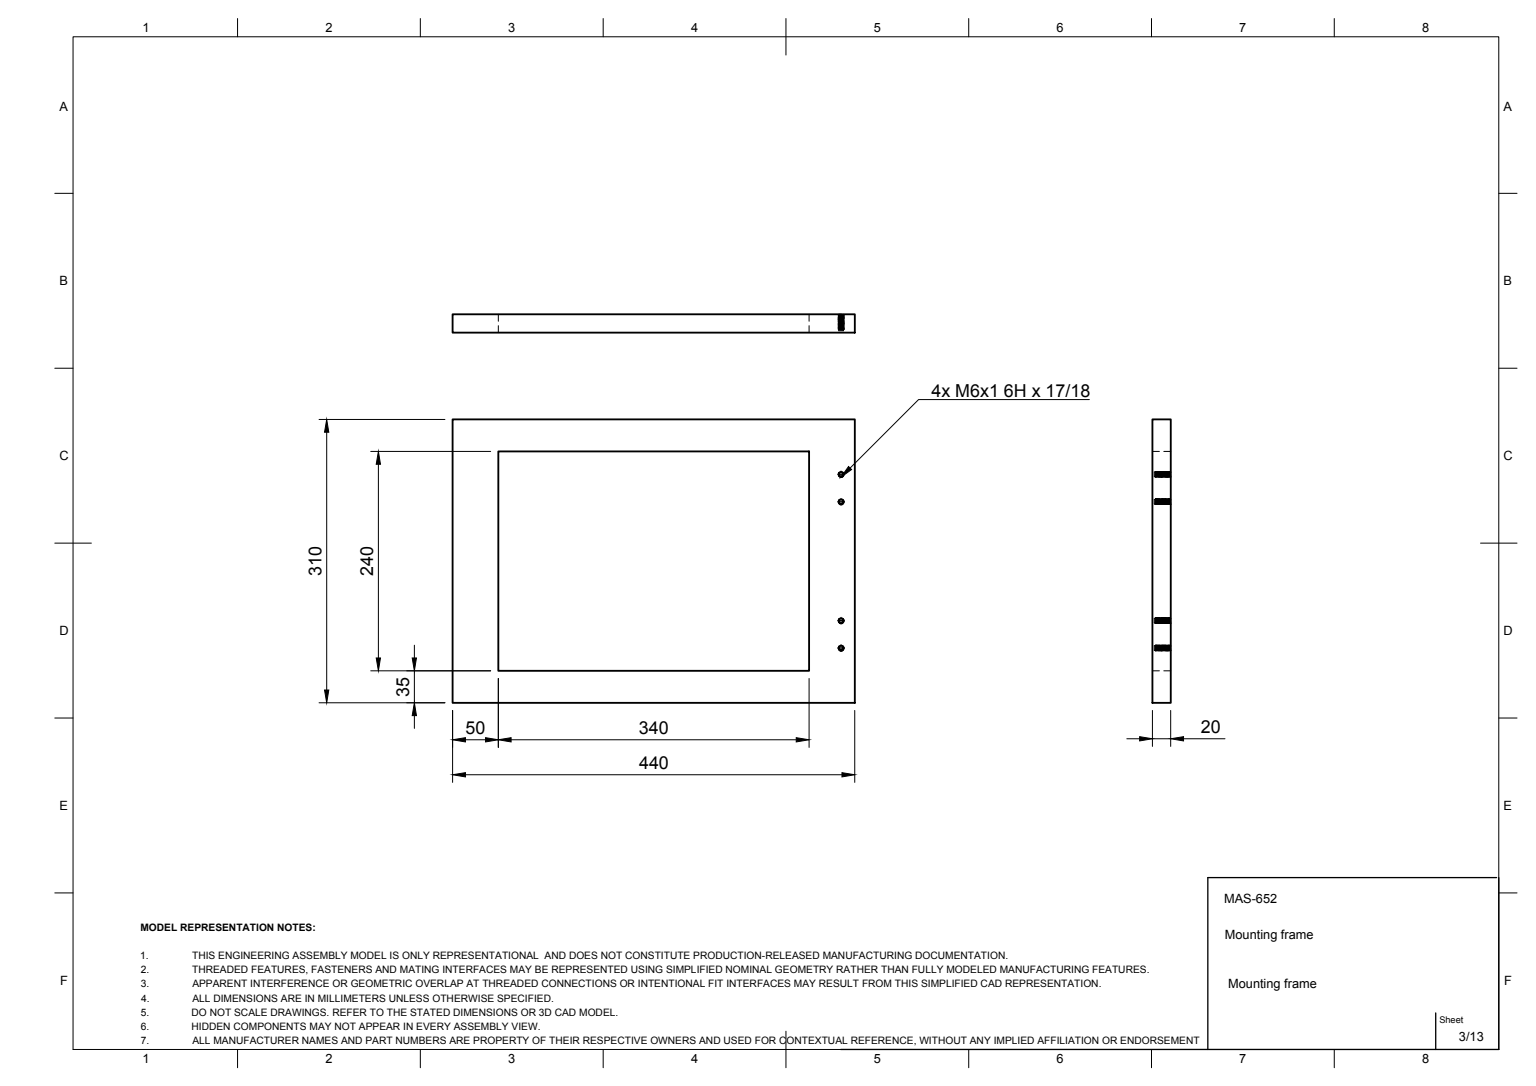
ISO-10303-21;
HEADER;
/* Generated by software containing ST-Developer
 * from STEP Tools, Inc. (www.steptools.com) 
 */

FILE_DESCRIPTION(
/* description */ ('Independent hinged machine back cover with retained hinge pins, perim
eter gasket and quarter-turn cam latch. Nominal cover 360 x 260 x 3 mm
, frame 430 x 300 x 20 mm. No guarding, structural or ingress rating a
ssigned.'),
/* implementation_level */ '2;1');

FILE_NAME(
/* name */ 'Mounting frame.step',
/* time_stamp */ '2026-11-09T19:36:59-08:00',
/* author */ (''),
/* organization */ (''),
/* preprocessor_version */ 'ST-DEVELOPER v20.2',
/* originating_system */ 'Autodesk Translation Framework v15.17.0.0',
/* authorisation */ '');

FILE_SCHEMA (('AUTOMOTIVE_DESIGN { 1 0 10303 214 3 1 1 }'));
ENDSEC;

DATA;
#10=MECHANICAL_DESIGN_GEOMETRIC_PRESENTATION_REPRESENTATION('',(#198),#32627);
#162=SHAPE_REPRESENTATION_RELATIONSHIP('SRR','None',#32708,#180);
#180=ADVANCED_BREP_SHAPE_REPRESENTATION('',(#216),#32609);
#198=STYLED_ITEM('',(#32807),#216);
#216=MANIFOLD_SOLID_BREP('Body1',#8675);
#234=FACE_BOUND('',#1096,.T.);
#235=FACE_BOUND('',#1098,.T.);
#236=FACE_BOUND('',#1099,.T.);
#237=FACE_BOUND('',#1100,.T.);
#238=FACE_BOUND('',#1101,.T.);
#239=FACE_BOUND('',#1102,.T.);
#293=B_SPLINE_SURFACE_WITH_KNOTS('',3,3,((#16428,#16429,#16430,#16431,#16432,
#16433,#16434,#16435,#16436,#16437,#16438,#16439,#16440,#16441,#16442,#16443,
#16444,#16445,#16446,#16447,#16448,#16449,#16450,#16451,#16452,#16453,#16454,
#16455,#16456,#16457,#16458,#16459,#16460,#16461,#16462,#16463,#16464,#16465,
#16466,#16467,#16468,#16469,#16470,#16471,#16472,#16473,#16474,#16475,#16476,
#16477,#16478,#16479,#16480,#16481,#16482,#16483,#16484,#16485,#16486,#16487,
#16488,#16489,#16490,#16491,#16492,#16493,#16494,#16495,#16496,#16497,#16498,
#16499,#16500,#16501,#16502,#16503,#16504,#16505,#16506,#16507,#16508,#16509,
#16510,#16511,#16512,#16513,#16514,#16515,#16516,#16517,#16518,#16519,#16520,
#16521,#16522,#16523,#16524,#16525,#16526,#16527,#16528,#16529,#16530,#16531,
#16532,#16533,#16534,#16535,#16536,#16537,#16538,#16539),(#16540,#16541,
#16542,#16543,#16544,#16545,#16546,#16547,#16548,#16549,#16550,#16551,#16552,
#16553,#16554,#16555,#16556,#16557,#16558,#16559,#16560,#16561,#16562,#16563,
#16564,#16565,#16566,#16567,#16568,#16569,#16570,#16571,#16572,#16573,#16574,
#16575,#16576,#16577,#16578,#16579,#16580,#16581,#16582,#16583,#16584,#16585,
#16586,#16587,#16588,#16589,#16590,#16591,#16592,#16593,#16594,#16595,#16596,
#16597,#16598,#16599,#16600,#16601,#16602,#16603,#16604,#16605,#16606,#16607,
#16608,#16609,#16610,#16611,#16612,#16613,#16614,#16615,#16616,#16617,#16618,
#16619,#16620,#16621,#16622,#16623,#16624,#16625,#16626,#16627,#16628,#16629,
#16630,#16631,#16632,#16633,#16634,#16635,#16636,#16637,#16638,#16639,#16640,
#16641,#16642,#16643,#16644,#16645,#16646,#16647,#16648,#16649,#16650,#16651),
(#16652,#16653,#16654,#16655,#16656,#16657,#16658,#16659,#16660,#16661,
#16662,#16663,#16664,#16665,#16666,#16667,#16668,#16669,#16670,#16671,#16672,
#16673,#16674,#16675,#16676,#16677,#16678,#16679,#16680,#16681,#16682,#16683,
#16684,#16685,#16686,#16687,#16688,#16689,#16690,#16691,#16692,#16693,#16694,
#16695,#16696,#16697,#16698,#16699,#16700,#16701,#16702,#16703,#16704,#16705,
#16706,#16707,#16708,#16709,#16710,#16711,#16712,#16713,#16714,#16715,#16716,
#16717,#16718,#16719,#16720,#16721,#16722,#16723,#16724,#16725,#16726,#16727,
#16728,#16729,#16730,#16731,#16732,#16733,#16734,#16735,#16736,#16737,#16738,
#16739,#16740,#16741,#16742,#16743,#16744,#16745,#16746,#16747,#16748,#16749,
#16750,#16751,#16752,#16753,#16754,#16755,#16756,#16757,#16758,#16759,#16760,
#16761,#16762,#16763),(#16764,#16765,#16766,#16767,#16768,#16769,#16770,
#16771,#16772,#16773,#16774,#16775,#16776,#16777,#16778,#16779,#16780,#16781,
#16782,#16783,#16784,#16785,#16786,#16787,#16788,#16789,#16790,#16791,#16792,
#16793,#16794,#16795,#16796,#16797,#16798,#16799,#16800,#16801,#16802,#16803,
#16804,#16805,#16806,#16807,#16808,#16809,#16810,#16811,#16812,#16813,#16814,
#16815,#16816,#16817,#16818,#16819,#16820,#16821,#16822,#16823,#16824,#16825,
#16826,#16827,#16828,#16829,#16830,#16831,#16832,#16833,#16834,#16835,#16836,
#16837,#16838,#16839,#16840,#16841,#16842,#16843,#16844,#16845,#16846,#16847,
#16848,#16849,#16850,#16851,#16852,#16853,#16854,#16855,#16856,#16857,#16858,
#16859,#16860,#16861,#16862,#16863,#16864,#16865,#16866,#16867,#16868,#16869,
#16870,#16871,#16872,#16873,#16874,#16875)),.UNSPECIFIED.,.F.,.F.,.F.,(4,
4),(4,1,1,1,1,1,1,1,1,1,1,1,1,1,1,1,1,1,1,1,1,1,1,1,1,1,1,1,1,1,1,1,1,1,
1,1,1,1,1,1,1,1,1,1,1,1,1,1,1,1,1,1,1,1,1,1,1,1,1,1,1,1,1,1,1,1,1,1,1,1,
1,1,1,1,1,1,1,1,1,1,1,1,1,1,1,1,1,1,1,1,1,1,1,1,1,1,1,1,1,1,1,1,1,1,1,1,
1,1,1,4),(0.,0.064201349933888),(11.8589888623077,12.8574392762075,13.8558896901074,
14.8543401040072,15.852790517907,16.8512409318069,17.8496913457067,18.8481417596065,
19.8465921735064,20.8450425874062,21.843493001306,22.8419434152058,23.8403938291057,
24.8388442430055,25.8372946569053,26.8357450708052,27.834195484705,28.8326458986048,
29.8310963125046,30.8295467264045,31.8279971403043,32.8264475542041,33.824897968104,
34.8233483820038,35.8217987959036,36.8202492098035,37.8186996237033,38.8171500376031,
39.8156004515029,40.8140508654028,41.8125012793026,42.8109516932024,43.8094021071023,
44.8078525210021,45.8063029349019,46.8047533488018,47.8032037627016,48.8016541766014,
49.8001045905012,50.7985550044011,51.7970054183009,52.7954558322007,53.7939062461006,
54.7923566600004,55.7908070739002,56.7892574878001,57.7877079016999,58.7861583155997,
59.7846087294995,60.7830591433994,61.7815095572992,62.779959971199,63.7784103850989,
64.7768607989987,65.7753112128985,66.7737616267983,67.7722120406982,68.770662454598,
69.7691128684978,70.7675632823977,71.7660136962975,72.7644641101973,73.7629145240972,
74.761364937997,75.7598153518968,76.7582657657966,77.7567161796965,78.7551665935963,
79.7536170074961,80.7520674213959,81.7505178352958,82.7489682491956,83.7474186630954,
84.7458690769953,85.7443194908951,86.7427699047949,87.7412203186948,88.7396707325946,
89.7381211464944,90.7365715603943,91.7350219742941,92.7334723881939,93.7319228020937,
94.7303732159936,95.7288236298934,96.7272740437932,97.7257244576931,98.7241748715929,
99.7226252854927,100.721075699393,101.719526113292,102.717976527192,103.716426941092,
104.714877354992,105.713327768892,106.711778182792,107.710228596691,108.708679010591,
109.707129424491,110.705579838391,111.704030252291,112.70248066619,113.70093108009,
114.69938149399,115.69783190789,116.69628232179,117.69473273569,118.693183149589,
119.691633563489,120.690083977389),.UNSPECIFIED.);
#294=B_SPLINE_SURFACE_WITH_KNOTS('',3,3,((#16998,#16999,#17000,#17001,#17002,
#17003,#17004,#17005,#17006,#17007,#17008,#17009,#17010,#17011,#17012,#17013,
#17014,#17015,#17016,#17017,#17018,#17019,#17020,#17021,#17022,#17023,#17024,
#17025,#17026,#17027,#17028,#17029,#17030,#17031,#17032,#17033,#17034,#17035,
#17036,#17037,#17038,#17039,#17040,#17041,#17042,#17043,#17044,#17045,#17046,
#17047,#17048,#17049,#17050,#17051,#17052,#17053,#17054,#17055,#17056,#17057,
#17058,#17059,#17060,#17061,#17062,#17063,#17064,#17065,#17066,#17067,#17068,
#17069,#17070,#17071,#17072,#17073,#17074,#17075,#17076,#17077,#17078,#17079,
#17080,#17081,#17082,#17083,#17084,#17085,#17086,#17087,#17088,#17089,#17090,
#17091,#17092,#17093,#17094,#17095,#17096,#17097,#17098,#17099,#17100,#17101,
#17102,#17103,#17104,#17105,#17106,#17107,#17108,#17109),(#17110,#17111,
#17112,#17113,#17114,#17115,#17116,#17117,#17118,#17119,#17120,#17121,#17122,
#17123,#17124,#17125,#17126,#17127,#17128,#17129,#17130,#17131,#17132,#17133,
#17134,#17135,#17136,#17137,#17138,#17139,#17140,#17141,#17142,#17143,#17144,
#17145,#17146,#17147,#17148,#17149,#17150,#17151,#17152,#17153,#17154,#17155,
#17156,#17157,#17158,#17159,#17160,#17161,#17162,#17163,#17164,#17165,#17166,
#17167,#17168,#17169,#17170,#17171,#17172,#17173,#17174,#17175,#17176,#17177,
#17178,#17179,#17180,#17181,#17182,#17183,#17184,#17185,#17186,#17187,#17188,
#17189,#17190,#17191,#17192,#17193,#17194,#17195,#17196,#17197,#17198,#17199,
#17200,#17201,#17202,#17203,#17204,#17205,#17206,#17207,#17208,#17209,#17210,
#17211,#17212,#17213,#17214,#17215,#17216,#17217,#17218,#17219,#17220,#17221),
(#17222,#17223,#17224,#17225,#17226,#17227,#17228,#17229,#17230,#17231,
#17232,#17233,#17234,#17235,#17236,#17237,#17238,#17239,#17240,#17241,#17242,
#17243,#17244,#17245,#17246,#17247,#17248,#17249,#17250,#17251,#17252,#17253,
#17254,#17255,#17256,#17257,#17258,#17259,#17260,#17261,#17262,#17263,#17264,
#17265,#17266,#17267,#17268,#17269,#17270,#17271,#17272,#17273,#17274,#17275,
#17276,#17277,#17278,#17279,#17280,#17281,#17282,#17283,#17284,#17285,#17286,
#17287,#17288,#17289,#17290,#17291,#17292,#17293,#17294,#17295,#17296,#17297,
#17298,#17299,#17300,#17301,#17302,#17303,#17304,#17305,#17306,#17307,#17308,
#17309,#17310,#17311,#17312,#17313,#17314,#17315,#17316,#17317,#17318,#17319,
#17320,#17321,#17322,#17323,#17324,#17325,#17326,#17327,#17328,#17329,#17330,
#17331,#17332,#17333),(#17334,#17335,#17336,#17337,#17338,#17339,#17340,
#17341,#17342,#17343,#17344,#17345,#17346,#17347,#17348,#17349,#17350,#17351,
#17352,#17353,#17354,#17355,#17356,#17357,#17358,#17359,#17360,#17361,#17362,
#17363,#17364,#17365,#17366,#17367,#17368,#17369,#17370,#17371,#17372,#17373,
#17374,#17375,#17376,#17377,#17378,#17379,#17380,#17381,#17382,#17383,#17384,
#17385,#17386,#17387,#17388,#17389,#17390,#17391,#17392,#17393,#17394,#17395,
#17396,#17397,#17398,#17399,#17400,#17401,#17402,#17403,#17404,#17405,#17406,
#17407,#17408,#17409,#17410,#17411,#17412,#17413,#17414,#17415,#17416,#17417,
#17418,#17419,#17420,#17421,#17422,#17423,#17424,#17425,#17426,#17427,#17428,
#17429,#17430,#17431,#17432,#17433,#17434,#17435,#17436,#17437,#17438,#17439,
#17440,#17441,#17442,#17443,#17444,#17445)),.UNSPECIFIED.,.F.,.F.,.F.,(4,
4),(4,1,1,1,1,1,1,1,1,1,1,1,1,1,1,1,1,1,1,1,1,1,1,1,1,1,1,1,1,1,1,1,1,1,
1,1,1,1,1,1,1,1,1,1,1,1,1,1,1,1,1,1,1,1,1,1,1,1,1,1,1,1,1,1,1,1,1,1,1,1,
1,1,1,1,1,1,1,1,1,1,1,1,1,1,1,1,1,1,1,1,1,1,1,1,1,1,1,1,1,1,1,1,1,1,1,1,
1,1,1,4),(0.,0.064201349933888),(14.3984001269718,15.3968505408716,16.3953009547714,
17.3937513686712,18.3922017825711,19.3906521964709,20.3891026103707,21.3875530242706,
22.3860034381704,23.3844538520702,24.3829042659701,25.3813546798699,26.3798050937697,
27.3782555076695,28.3767059215694,29.3751563354692,30.373606749369,31.3720571632689,
32.3705075771687,33.3689579910685,34.3674084049683,35.3658588188682,36.364309232768,
37.3627596466678,38.3612100605677,39.3596604744675,40.3581108883673,41.3565613022672,
42.355011716167,43.3534621300668,44.3519125439666,45.3503629578665,46.3488133717663,
47.3472637856661,48.345714199566,49.3441646134658,50.3426150273656,51.3410654412654,
52.3395158551653,53.3379662690651,54.3364166829649,55.3348670968648,56.3333175107646,
57.3317679246644,58.3302183385643,59.3286687524641,60.3271191663639,61.3255695802637,
62.3240199941636,63.3224704080634,64.3209208219632,65.3193712358631,66.3178216497629,
67.3162720636627,68.3147224775625,69.3131728914624,70.3116233053622,71.310073719262,
72.3085241331619,73.3069745470617,74.3054249609615,75.3038753748613,76.3023257887612,
77.300776202661,78.2992266165608,79.2976770304607,80.2961274443605,81.2945778582603,
82.2930282721602,83.29147868606,84.2899290999598,85.2883795138596,86.2868299277595,
87.2852803416593,88.2837307555591,89.282181169459,90.2806315833588,91.2790819972586,
92.2775324111584,93.2759828250583,94.2744332389581,95.2728836528579,96.2713340667578,
97.2697844806576,98.2682348945574,99.2666853084573,100.265135722357,101.263586136257,
102.262036550157,103.260486964057,104.258937377956,105.257387791856,106.255838205756,
107.254288619656,108.252739033556,109.251189447456,110.249639861355,111.248090275255,
112.246540689155,113.244991103055,114.243441516955,115.241891930855,116.240342344754,
117.238792758654,118.237243172554,119.235693586454,120.234144000354,121.232594414253,
122.231044828153,123.229495242053),.UNSPECIFIED.);
#295=B_SPLINE_SURFACE_WITH_KNOTS('',3,3,((#17768,#17769,#17770,#17771,#17772,
#17773,#17774,#17775,#17776,#17777,#17778,#17779,#17780,#17781,#17782,#17783,
#17784,#17785,#17786,#17787,#17788,#17789,#17790,#17791,#17792,#17793,#17794,
#17795,#17796,#17797,#17798,#17799,#17800,#17801,#17802,#17803,#17804,#17805,
#17806,#17807,#17808,#17809,#17810,#17811,#17812,#17813,#17814,#17815,#17816,
#17817,#17818,#17819,#17820,#17821,#17822,#17823,#17824,#17825,#17826,#17827,
#17828,#17829,#17830,#17831,#17832,#17833,#17834,#17835,#17836,#17837,#17838,
#17839,#17840,#17841,#17842,#17843,#17844,#17845,#17846,#17847,#17848,#17849,
#17850,#17851,#17852,#17853,#17854,#17855,#17856,#17857,#17858,#17859,#17860,
#17861,#17862,#17863,#17864,#17865,#17866,#17867,#17868,#17869,#17870,#17871,
#17872,#17873,#17874,#17875,#17876,#17877,#17878,#17879),(#17880,#17881,
#17882,#17883,#17884,#17885,#17886,#17887,#17888,#17889,#17890,#17891,#17892,
#17893,#17894,#17895,#17896,#17897,#17898,#17899,#17900,#17901,#17902,#17903,
#17904,#17905,#17906,#17907,#17908,#17909,#17910,#17911,#17912,#17913,#17914,
#17915,#17916,#17917,#17918,#17919,#17920,#17921,#17922,#17923,#17924,#17925,
#17926,#17927,#17928,#17929,#17930,#17931,#17932,#17933,#17934,#17935,#17936,
#17937,#17938,#17939,#17940,#17941,#17942,#17943,#17944,#17945,#17946,#17947,
#17948,#17949,#17950,#17951,#17952,#17953,#17954,#17955,#17956,#17957,#17958,
#17959,#17960,#17961,#17962,#17963,#17964,#17965,#17966,#17967,#17968,#17969,
#17970,#17971,#17972,#17973,#17974,#17975,#17976,#17977,#17978,#17979,#17980,
#17981,#17982,#17983,#17984,#17985,#17986,#17987,#17988,#17989,#17990,#17991),
(#17992,#17993,#17994,#17995,#17996,#17997,#17998,#17999,#18000,#18001,
#18002,#18003,#18004,#18005,#18006,#18007,#18008,#18009,#18010,#18011,#18012,
#18013,#18014,#18015,#18016,#18017,#18018,#18019,#18020,#18021,#18022,#18023,
#18024,#18025,#18026,#18027,#18028,#18029,#18030,#18031,#18032,#18033,#18034,
#18035,#18036,#18037,#18038,#18039,#18040,#18041,#18042,#18043,#18044,#18045,
#18046,#18047,#18048,#18049,#18050,#18051,#18052,#18053,#18054,#18055,#18056,
#18057,#18058,#18059,#18060,#18061,#18062,#18063,#18064,#18065,#18066,#18067,
#18068,#18069,#18070,#18071,#18072,#18073,#18074,#18075,#18076,#18077,#18078,
#18079,#18080,#18081,#18082,#18083,#18084,#18085,#18086,#18087,#18088,#18089,
#18090,#18091,#18092,#18093,#18094,#18095,#18096,#18097,#18098,#18099,#18100,
#18101,#18102,#18103),(#18104,#18105,#18106,#18107,#18108,#18109,#18110,
#18111,#18112,#18113,#18114,#18115,#18116,#18117,#18118,#18119,#18120,#18121,
#18122,#18123,#18124,#18125,#18126,#18127,#18128,#18129,#18130,#18131,#18132,
#18133,#18134,#18135,#18136,#18137,#18138,#18139,#18140,#18141,#18142,#18143,
#18144,#18145,#18146,#18147,#18148,#18149,#18150,#18151,#18152,#18153,#18154,
#18155,#18156,#18157,#18158,#18159,#18160,#18161,#18162,#18163,#18164,#18165,
#18166,#18167,#18168,#18169,#18170,#18171,#18172,#18173,#18174,#18175,#18176,
#18177,#18178,#18179,#18180,#18181,#18182,#18183,#18184,#18185,#18186,#18187,
#18188,#18189,#18190,#18191,#18192,#18193,#18194,#18195,#18196,#18197,#18198,
#18199,#18200,#18201,#18202,#18203,#18204,#18205,#18206,#18207,#18208,#18209,
#18210,#18211,#18212,#18213,#18214,#18215)),.UNSPECIFIED.,.F.,.F.,.F.,(4,
4),(4,1,1,1,1,1,1,1,1,1,1,1,1,1,1,1,1,1,1,1,1,1,1,1,1,1,1,1,1,1,1,1,1,1,
1,1,1,1,1,1,1,1,1,1,1,1,1,1,1,1,1,1,1,1,1,1,1,1,1,1,1,1,1,1,1,1,1,1,1,1,
1,1,1,1,1,1,1,1,1,1,1,1,1,1,1,1,1,1,1,1,1,1,1,1,1,1,1,1,1,1,1,1,1,1,1,1,
1,1,1,4),(0.,0.064201349933888),(11.8589888623077,12.8574392762076,13.8558896901074,
14.8543401040072,15.852790517907,16.8512409318069,17.8496913457067,18.8481417596065,
19.8465921735064,20.8450425874062,21.843493001306,22.8419434152058,23.8403938291057,
24.8388442430055,25.8372946569053,26.8357450708052,27.834195484705,28.8326458986048,
29.8310963125047,30.8295467264045,31.8279971403043,32.8264475542041,33.824897968104,
34.8233483820038,35.8217987959036,36.8202492098035,37.8186996237033,38.8171500376031,
39.8156004515029,40.8140508654028,41.8125012793026,42.8109516932024,43.8094021071023,
44.8078525210021,45.8063029349019,46.8047533488018,47.8032037627016,48.8016541766014,
49.8001045905012,50.7985550044011,51.7970054183009,52.7954558322007,53.7939062461006,
54.7923566600004,55.7908070739002,56.7892574878001,57.7877079016999,58.7861583155997,
59.7846087294995,60.7830591433994,61.7815095572992,62.779959971199,63.7784103850989,
64.7768607989987,65.7753112128985,66.7737616267983,67.7722120406982,68.770662454598,
69.7691128684978,70.7675632823977,71.7660136962975,72.7644641101973,73.7629145240971,
74.761364937997,75.7598153518968,76.7582657657966,77.7567161796965,78.7551665935963,
79.7536170074961,80.7520674213959,81.7505178352958,82.7489682491956,83.7474186630954,
84.7458690769953,85.7443194908951,86.7427699047949,87.7412203186948,88.7396707325946,
89.7381211464944,90.7365715603942,91.7350219742941,92.7334723881939,93.7319228020937,
94.7303732159936,95.7288236298934,96.7272740437932,97.725724457693,98.7241748715929,
99.7226252854927,100.721075699393,101.719526113292,102.717976527192,103.716426941092,
104.714877354992,105.713327768892,106.711778182792,107.710228596691,108.708679010591,
109.707129424491,110.705579838391,111.704030252291,112.70248066619,113.70093108009,
114.69938149399,115.69783190789,116.69628232179,117.69473273569,118.693183149589,
119.691633563489,120.690083977389),.UNSPECIFIED.);
#296=B_SPLINE_SURFACE_WITH_KNOTS('',3,3,((#18338,#18339,#18340,#18341,#18342,
#18343,#18344,#18345,#18346,#18347,#18348,#18349,#18350,#18351,#18352,#18353,
#18354,#18355,#18356,#18357,#18358,#18359,#18360,#18361,#18362,#18363,#18364,
#18365,#18366,#18367,#18368,#18369,#18370,#18371,#18372,#18373,#18374,#18375,
#18376,#18377,#18378,#18379,#18380,#18381,#18382,#18383,#18384,#18385,#18386,
#18387,#18388,#18389,#18390,#18391,#18392,#18393,#18394,#18395,#18396,#18397,
#18398,#18399,#18400,#18401,#18402,#18403,#18404,#18405,#18406,#18407,#18408,
#18409,#18410,#18411,#18412,#18413,#18414,#18415,#18416,#18417,#18418,#18419,
#18420,#18421,#18422,#18423,#18424,#18425,#18426,#18427,#18428,#18429,#18430,
#18431,#18432,#18433,#18434,#18435,#18436,#18437,#18438,#18439,#18440,#18441,
#18442,#18443,#18444,#18445,#18446,#18447,#18448,#18449),(#18450,#18451,
#18452,#18453,#18454,#18455,#18456,#18457,#18458,#18459,#18460,#18461,#18462,
#18463,#18464,#18465,#18466,#18467,#18468,#18469,#18470,#18471,#18472,#18473,
#18474,#18475,#18476,#18477,#18478,#18479,#18480,#18481,#18482,#18483,#18484,
#18485,#18486,#18487,#18488,#18489,#18490,#18491,#18492,#18493,#18494,#18495,
#18496,#18497,#18498,#18499,#18500,#18501,#18502,#18503,#18504,#18505,#18506,
#18507,#18508,#18509,#18510,#18511,#18512,#18513,#18514,#18515,#18516,#18517,
#18518,#18519,#18520,#18521,#18522,#18523,#18524,#18525,#18526,#18527,#18528,
#18529,#18530,#18531,#18532,#18533,#18534,#18535,#18536,#18537,#18538,#18539,
#18540,#18541,#18542,#18543,#18544,#18545,#18546,#18547,#18548,#18549,#18550,
#18551,#18552,#18553,#18554,#18555,#18556,#18557,#18558,#18559,#18560,#18561),
(#18562,#18563,#18564,#18565,#18566,#18567,#18568,#18569,#18570,#18571,
#18572,#18573,#18574,#18575,#18576,#18577,#18578,#18579,#18580,#18581,#18582,
#18583,#18584,#18585,#18586,#18587,#18588,#18589,#18590,#18591,#18592,#18593,
#18594,#18595,#18596,#18597,#18598,#18599,#18600,#18601,#18602,#18603,#18604,
#18605,#18606,#18607,#18608,#18609,#18610,#18611,#18612,#18613,#18614,#18615,
#18616,#18617,#18618,#18619,#18620,#18621,#18622,#18623,#18624,#18625,#18626,
#18627,#18628,#18629,#18630,#18631,#18632,#18633,#18634,#18635,#18636,#18637,
#18638,#18639,#18640,#18641,#18642,#18643,#18644,#18645,#18646,#18647,#18648,
#18649,#18650,#18651,#18652,#18653,#18654,#18655,#18656,#18657,#18658,#18659,
#18660,#18661,#18662,#18663,#18664,#18665,#18666,#18667,#18668,#18669,#18670,
#18671,#18672,#18673),(#18674,#18675,#18676,#18677,#18678,#18679,#18680,
#18681,#18682,#18683,#18684,#18685,#18686,#18687,#18688,#18689,#18690,#18691,
#18692,#18693,#18694,#18695,#18696,#18697,#18698,#18699,#18700,#18701,#18702,
#18703,#18704,#18705,#18706,#18707,#18708,#18709,#18710,#18711,#18712,#18713,
#18714,#18715,#18716,#18717,#18718,#18719,#18720,#18721,#18722,#18723,#18724,
#18725,#18726,#18727,#18728,#18729,#18730,#18731,#18732,#18733,#18734,#18735,
#18736,#18737,#18738,#18739,#18740,#18741,#18742,#18743,#18744,#18745,#18746,
#18747,#18748,#18749,#18750,#18751,#18752,#18753,#18754,#18755,#18756,#18757,
#18758,#18759,#18760,#18761,#18762,#18763,#18764,#18765,#18766,#18767,#18768,
#18769,#18770,#18771,#18772,#18773,#18774,#18775,#18776,#18777,#18778,#18779,
#18780,#18781,#18782,#18783,#18784,#18785)),.UNSPECIFIED.,.F.,.F.,.F.,(4,
4),(4,1,1,1,1,1,1,1,1,1,1,1,1,1,1,1,1,1,1,1,1,1,1,1,1,1,1,1,1,1,1,1,1,1,
1,1,1,1,1,1,1,1,1,1,1,1,1,1,1,1,1,1,1,1,1,1,1,1,1,1,1,1,1,1,1,1,1,1,1,1,
1,1,1,1,1,1,1,1,1,1,1,1,1,1,1,1,1,1,1,1,1,1,1,1,1,1,1,1,1,1,1,1,1,1,1,1,
1,1,1,4),(0.,0.064201349933888),(14.3984001269718,15.3968505408716,16.3953009547714,
17.3937513686712,18.3922017825711,19.3906521964709,20.3891026103707,21.3875530242706,
22.3860034381704,23.3844538520702,24.38290426597,25.3813546798699,26.3798050937697,
27.3782555076695,28.3767059215694,29.3751563354692,30.373606749369,31.3720571632688,
32.3705075771687,33.3689579910685,34.3674084049683,35.3658588188682,36.364309232768,
37.3627596466678,38.3612100605677,39.3596604744675,40.3581108883673,41.3565613022671,
42.355011716167,43.3534621300668,44.3519125439666,45.3503629578665,46.3488133717663,
47.3472637856661,48.3457141995659,49.3441646134658,50.3426150273656,51.3410654412654,
52.3395158551653,53.3379662690651,54.3364166829649,55.3348670968648,56.3333175107646,
57.3317679246644,58.3302183385642,59.3286687524641,60.3271191663639,61.3255695802637,
62.3240199941636,63.3224704080634,64.3209208219632,65.319371235863,66.3178216497629,
67.3162720636627,68.3147224775625,69.3131728914624,70.3116233053622,71.310073719262,
72.3085241331619,73.3069745470617,74.3054249609615,75.3038753748613,76.3023257887612,
77.300776202661,78.2992266165608,79.2976770304607,80.2961274443605,81.2945778582603,
82.2930282721601,83.29147868606,84.2899290999598,85.2883795138596,86.2868299277595,
87.2852803416593,88.2837307555591,89.282181169459,90.2806315833588,91.2790819972586,
92.2775324111584,93.2759828250583,94.2744332389581,95.2728836528579,96.2713340667578,
97.2697844806576,98.2682348945574,99.2666853084572,100.265135722357,101.263586136257,
102.262036550157,103.260486964057,104.258937377956,105.257387791856,106.255838205756,
107.254288619656,108.252739033556,109.251189447456,110.249639861355,111.248090275255,
112.246540689155,113.244991103055,114.243441516955,115.241891930855,116.240342344754,
117.238792758654,118.237243172554,119.235693586454,120.234144000354,121.232594414253,
122.231044828153,123.229495242053),.UNSPECIFIED.);
#297=B_SPLINE_SURFACE_WITH_KNOTS('',3,3,((#19108,#19109,#19110,#19111,#19112,
#19113,#19114,#19115,#19116,#19117,#19118,#19119,#19120,#19121,#19122,#19123,
#19124,#19125,#19126,#19127,#19128,#19129,#19130,#19131,#19132,#19133,#19134,
#19135,#19136,#19137,#19138,#19139,#19140,#19141,#19142,#19143,#19144,#19145,
#19146,#19147,#19148,#19149,#19150,#19151,#19152,#19153,#19154,#19155,#19156,
#19157,#19158,#19159,#19160,#19161,#19162,#19163,#19164,#19165,#19166,#19167,
#19168,#19169,#19170,#19171,#19172,#19173,#19174,#19175,#19176,#19177,#19178,
#19179,#19180,#19181,#19182,#19183,#19184,#19185,#19186,#19187,#19188,#19189,
#19190,#19191,#19192,#19193,#19194,#19195,#19196,#19197,#19198,#19199,#19200,
#19201,#19202,#19203,#19204,#19205,#19206,#19207,#19208,#19209,#19210,#19211,
#19212,#19213,#19214,#19215,#19216,#19217,#19218,#19219),(#19220,#19221,
#19222,#19223,#19224,#19225,#19226,#19227,#19228,#19229,#19230,#19231,#19232,
#19233,#19234,#19235,#19236,#19237,#19238,#19239,#19240,#19241,#19242,#19243,
#19244,#19245,#19246,#19247,#19248,#19249,#19250,#19251,#19252,#19253,#19254,
#19255,#19256,#19257,#19258,#19259,#19260,#19261,#19262,#19263,#19264,#19265,
#19266,#19267,#19268,#19269,#19270,#19271,#19272,#19273,#19274,#19275,#19276,
#19277,#19278,#19279,#19280,#19281,#19282,#19283,#19284,#19285,#19286,#19287,
#19288,#19289,#19290,#19291,#19292,#19293,#19294,#19295,#19296,#19297,#19298,
#19299,#19300,#19301,#19302,#19303,#19304,#19305,#19306,#19307,#19308,#19309,
#19310,#19311,#19312,#19313,#19314,#19315,#19316,#19317,#19318,#19319,#19320,
#19321,#19322,#19323,#19324,#19325,#19326,#19327,#19328,#19329,#19330,#19331),
(#19332,#19333,#19334,#19335,#19336,#19337,#19338,#19339,#19340,#19341,
#19342,#19343,#19344,#19345,#19346,#19347,#19348,#19349,#19350,#19351,#19352,
#19353,#19354,#19355,#19356,#19357,#19358,#19359,#19360,#19361,#19362,#19363,
#19364,#19365,#19366,#19367,#19368,#19369,#19370,#19371,#19372,#19373,#19374,
#19375,#19376,#19377,#19378,#19379,#19380,#19381,#19382,#19383,#19384,#19385,
#19386,#19387,#19388,#19389,#19390,#19391,#19392,#19393,#19394,#19395,#19396,
#19397,#19398,#19399,#19400,#19401,#19402,#19403,#19404,#19405,#19406,#19407,
#19408,#19409,#19410,#19411,#19412,#19413,#19414,#19415,#19416,#19417,#19418,
#19419,#19420,#19421,#19422,#19423,#19424,#19425,#19426,#19427,#19428,#19429,
#19430,#19431,#19432,#19433,#19434,#19435,#19436,#19437,#19438,#19439,#19440,
#19441,#19442,#19443),(#19444,#19445,#19446,#19447,#19448,#19449,#19450,
#19451,#19452,#19453,#19454,#19455,#19456,#19457,#19458,#19459,#19460,#19461,
#19462,#19463,#19464,#19465,#19466,#19467,#19468,#19469,#19470,#19471,#19472,
#19473,#19474,#19475,#19476,#19477,#19478,#19479,#19480,#19481,#19482,#19483,
#19484,#19485,#19486,#19487,#19488,#19489,#19490,#19491,#19492,#19493,#19494,
#19495,#19496,#19497,#19498,#19499,#19500,#19501,#19502,#19503,#19504,#19505,
#19506,#19507,#19508,#19509,#19510,#19511,#19512,#19513,#19514,#19515,#19516,
#19517,#19518,#19519,#19520,#19521,#19522,#19523,#19524,#19525,#19526,#19527,
#19528,#19529,#19530,#19531,#19532,#19533,#19534,#19535,#19536,#19537,#19538,
#19539,#19540,#19541,#19542,#19543,#19544,#19545,#19546,#19547,#19548,#19549,
#19550,#19551,#19552,#19553,#19554,#19555)),.UNSPECIFIED.,.F.,.F.,.F.,(4,
4),(4,1,1,1,1,1,1,1,1,1,1,1,1,1,1,1,1,1,1,1,1,1,1,1,1,1,1,1,1,1,1,1,1,1,
1,1,1,1,1,1,1,1,1,1,1,1,1,1,1,1,1,1,1,1,1,1,1,1,1,1,1,1,1,1,1,1,1,1,1,1,
1,1,1,1,1,1,1,1,1,1,1,1,1,1,1,1,1,1,1,1,1,1,1,1,1,1,1,1,1,1,1,1,1,1,1,1,
1,1,1,4),(0.,0.064201349933888),(11.8589888623077,12.8574392762076,13.8558896901074,
14.8543401040072,15.852790517907,16.8512409318069,17.8496913457067,18.8481417596065,
19.8465921735064,20.8450425874062,21.843493001306,22.8419434152058,23.8403938291057,
24.8388442430055,25.8372946569053,26.8357450708052,27.834195484705,28.8326458986048,
29.8310963125047,30.8295467264045,31.8279971403043,32.8264475542041,33.824897968104,
34.8233483820038,35.8217987959036,36.8202492098035,37.8186996237033,38.8171500376031,
39.8156004515029,40.8140508654028,41.8125012793026,42.8109516932024,43.8094021071023,
44.8078525210021,45.8063029349019,46.8047533488018,47.8032037627016,48.8016541766014,
49.8001045905012,50.7985550044011,51.7970054183009,52.7954558322007,53.7939062461006,
54.7923566600004,55.7908070739002,56.7892574878,57.7877079016999,58.7861583155997,
59.7846087294995,60.7830591433994,61.7815095572992,62.779959971199,63.7784103850989,
64.7768607989987,65.7753112128985,66.7737616267983,67.7722120406982,68.770662454598,
69.7691128684978,70.7675632823977,71.7660136962975,72.7644641101973,73.7629145240972,
74.761364937997,75.7598153518968,76.7582657657966,77.7567161796965,78.7551665935963,
79.7536170074961,80.752067421396,81.7505178352958,82.7489682491956,83.7474186630954,
84.7458690769953,85.7443194908951,86.7427699047949,87.7412203186948,88.7396707325946,
89.7381211464944,90.7365715603943,91.7350219742941,92.7334723881939,93.7319228020937,
94.7303732159936,95.7288236298934,96.7272740437932,97.7257244576931,98.7241748715929,
99.7226252854927,100.721075699393,101.719526113292,102.717976527192,103.716426941092,
104.714877354992,105.713327768892,106.711778182792,107.710228596691,108.708679010591,
109.707129424491,110.705579838391,111.704030252291,112.70248066619,113.70093108009,
114.69938149399,115.69783190789,116.69628232179,117.69473273569,118.693183149589,
119.691633563489,120.690083977389),.UNSPECIFIED.);
#298=B_SPLINE_SURFACE_WITH_KNOTS('',3,3,((#19678,#19679,#19680,#19681,#19682,
#19683,#19684,#19685,#19686,#19687,#19688,#19689,#19690,#19691,#19692,#19693,
#19694,#19695,#19696,#19697,#19698,#19699,#19700,#19701,#19702,#19703,#19704,
#19705,#19706,#19707,#19708,#19709,#19710,#19711,#19712,#19713,#19714,#19715,
#19716,#19717,#19718,#19719,#19720,#19721,#19722,#19723,#19724,#19725,#19726,
#19727,#19728,#19729,#19730,#19731,#19732,#19733,#19734,#19735,#19736,#19737,
#19738,#19739,#19740,#19741,#19742,#19743,#19744,#19745,#19746,#19747,#19748,
#19749,#19750,#19751,#19752,#19753,#19754,#19755,#19756,#19757,#19758,#19759,
#19760,#19761,#19762,#19763,#19764,#19765,#19766,#19767,#19768,#19769,#19770,
#19771,#19772,#19773,#19774,#19775,#19776,#19777,#19778,#19779,#19780,#19781,
#19782,#19783,#19784,#19785,#19786,#19787,#19788,#19789),(#19790,#19791,
#19792,#19793,#19794,#19795,#19796,#19797,#19798,#19799,#19800,#19801,#19802,
#19803,#19804,#19805,#19806,#19807,#19808,#19809,#19810,#19811,#19812,#19813,
#19814,#19815,#19816,#19817,#19818,#19819,#19820,#19821,#19822,#19823,#19824,
#19825,#19826,#19827,#19828,#19829,#19830,#19831,#19832,#19833,#19834,#19835,
#19836,#19837,#19838,#19839,#19840,#19841,#19842,#19843,#19844,#19845,#19846,
#19847,#19848,#19849,#19850,#19851,#19852,#19853,#19854,#19855,#19856,#19857,
#19858,#19859,#19860,#19861,#19862,#19863,#19864,#19865,#19866,#19867,#19868,
#19869,#19870,#19871,#19872,#19873,#19874,#19875,#19876,#19877,#19878,#19879,
#19880,#19881,#19882,#19883,#19884,#19885,#19886,#19887,#19888,#19889,#19890,
#19891,#19892,#19893,#19894,#19895,#19896,#19897,#19898,#19899,#19900,#19901),
(#19902,#19903,#19904,#19905,#19906,#19907,#19908,#19909,#19910,#19911,
#19912,#19913,#19914,#19915,#19916,#19917,#19918,#19919,#19920,#19921,#19922,
#19923,#19924,#19925,#19926,#19927,#19928,#19929,#19930,#19931,#19932,#19933,
#19934,#19935,#19936,#19937,#19938,#19939,#19940,#19941,#19942,#19943,#19944,
#19945,#19946,#19947,#19948,#19949,#19950,#19951,#19952,#19953,#19954,#19955,
#19956,#19957,#19958,#19959,#19960,#19961,#19962,#19963,#19964,#19965,#19966,
#19967,#19968,#19969,#19970,#19971,#19972,#19973,#19974,#19975,#19976,#19977,
#19978,#19979,#19980,#19981,#19982,#19983,#19984,#19985,#19986,#19987,#19988,
#19989,#19990,#19991,#19992,#19993,#19994,#19995,#19996,#19997,#19998,#19999,
#20000,#20001,#20002,#20003,#20004,#20005,#20006,#20007,#20008,#20009,#20010,
#20011,#20012,#20013),(#20014,#20015,#20016,#20017,#20018,#20019,#20020,
#20021,#20022,#20023,#20024,#20025,#20026,#20027,#20028,#20029,#20030,#20031,
#20032,#20033,#20034,#20035,#20036,#20037,#20038,#20039,#20040,#20041,#20042,
#20043,#20044,#20045,#20046,#20047,#20048,#20049,#20050,#20051,#20052,#20053,
#20054,#20055,#20056,#20057,#20058,#20059,#20060,#20061,#20062,#20063,#20064,
#20065,#20066,#20067,#20068,#20069,#20070,#20071,#20072,#20073,#20074,#20075,
#20076,#20077,#20078,#20079,#20080,#20081,#20082,#20083,#20084,#20085,#20086,
#20087,#20088,#20089,#20090,#20091,#20092,#20093,#20094,#20095,#20096,#20097,
#20098,#20099,#20100,#20101,#20102,#20103,#20104,#20105,#20106,#20107,#20108,
#20109,#20110,#20111,#20112,#20113,#20114,#20115,#20116,#20117,#20118,#20119,
#20120,#20121,#20122,#20123,#20124,#20125)),.UNSPECIFIED.,.F.,.F.,.F.,(4,
4),(4,1,1,1,1,1,1,1,1,1,1,1,1,1,1,1,1,1,1,1,1,1,1,1,1,1,1,1,1,1,1,1,1,1,
1,1,1,1,1,1,1,1,1,1,1,1,1,1,1,1,1,1,1,1,1,1,1,1,1,1,1,1,1,1,1,1,1,1,1,1,
1,1,1,1,1,1,1,1,1,1,1,1,1,1,1,1,1,1,1,1,1,1,1,1,1,1,1,1,1,1,1,1,1,1,1,1,
1,1,1,4),(0.,0.064201349933888),(14.3984001269717,15.3968505408716,16.3953009547714,
17.3937513686712,18.3922017825711,19.3906521964709,20.3891026103707,21.3875530242705,
22.3860034381704,23.3844538520702,24.38290426597,25.3813546798699,26.3798050937697,
27.3782555076695,28.3767059215694,29.3751563354692,30.373606749369,31.3720571632688,
32.3705075771687,33.3689579910685,34.3674084049683,35.3658588188682,36.364309232768,
37.3627596466678,38.3612100605677,39.3596604744675,40.3581108883673,41.3565613022671,
42.355011716167,43.3534621300668,44.3519125439666,45.3503629578665,46.3488133717663,
47.3472637856661,48.3457141995659,49.3441646134658,50.3426150273656,51.3410654412654,
52.3395158551653,53.3379662690651,54.3364166829649,55.3348670968648,56.3333175107646,
57.3317679246644,58.3302183385642,59.3286687524641,60.3271191663639,61.3255695802637,
62.3240199941636,63.3224704080634,64.3209208219632,65.319371235863,66.3178216497629,
67.3162720636627,68.3147224775625,69.3131728914624,70.3116233053622,71.310073719262,
72.3085241331619,73.3069745470617,74.3054249609615,75.3038753748613,76.3023257887612,
77.300776202661,78.2992266165608,79.2976770304606,80.2961274443605,81.2945778582603,
82.2930282721601,83.29147868606,84.2899290999598,85.2883795138596,86.2868299277595,
87.2852803416593,88.2837307555591,89.282181169459,90.2806315833588,91.2790819972586,
92.2775324111584,93.2759828250583,94.2744332389581,95.2728836528579,96.2713340667578,
97.2697844806576,98.2682348945574,99.2666853084572,100.265135722357,101.263586136257,
102.262036550157,103.260486964057,104.258937377956,105.257387791856,106.255838205756,
107.254288619656,108.252739033556,109.251189447456,110.249639861355,111.248090275255,
112.246540689155,113.244991103055,114.243441516955,115.241891930855,116.240342344754,
117.238792758654,118.237243172554,119.235693586454,120.234144000354,121.232594414253,
122.231044828153,123.229495242053),.UNSPECIFIED.);
#299=B_SPLINE_SURFACE_WITH_KNOTS('',3,3,((#20448,#20449,#20450,#20451,#20452,
#20453,#20454,#20455,#20456,#20457,#20458,#20459,#20460,#20461,#20462,#20463,
#20464,#20465,#20466,#20467,#20468,#20469,#20470,#20471,#20472,#20473,#20474,
#20475,#20476,#20477,#20478,#20479,#20480,#20481,#20482,#20483,#20484,#20485,
#20486,#20487,#20488,#20489,#20490,#20491,#20492,#20493,#20494,#20495,#20496,
#20497,#20498,#20499,#20500,#20501,#20502,#20503,#20504,#20505,#20506,#20507,
#20508,#20509,#20510,#20511,#20512,#20513,#20514,#20515,#20516,#20517,#20518,
#20519,#20520,#20521,#20522,#20523,#20524,#20525,#20526,#20527,#20528,#20529,
#20530,#20531,#20532,#20533,#20534,#20535,#20536,#20537,#20538,#20539,#20540,
#20541,#20542,#20543,#20544,#20545,#20546,#20547,#20548,#20549,#20550,#20551,
#20552,#20553,#20554,#20555,#20556,#20557,#20558,#20559),(#20560,#20561,
#20562,#20563,#20564,#20565,#20566,#20567,#20568,#20569,#20570,#20571,#20572,
#20573,#20574,#20575,#20576,#20577,#20578,#20579,#20580,#20581,#20582,#20583,
#20584,#20585,#20586,#20587,#20588,#20589,#20590,#20591,#20592,#20593,#20594,
#20595,#20596,#20597,#20598,#20599,#20600,#20601,#20602,#20603,#20604,#20605,
#20606,#20607,#20608,#20609,#20610,#20611,#20612,#20613,#20614,#20615,#20616,
#20617,#20618,#20619,#20620,#20621,#20622,#20623,#20624,#20625,#20626,#20627,
#20628,#20629,#20630,#20631,#20632,#20633,#20634,#20635,#20636,#20637,#20638,
#20639,#20640,#20641,#20642,#20643,#20644,#20645,#20646,#20647,#20648,#20649,
#20650,#20651,#20652,#20653,#20654,#20655,#20656,#20657,#20658,#20659,#20660,
#20661,#20662,#20663,#20664,#20665,#20666,#20667,#20668,#20669,#20670,#20671),
(#20672,#20673,#20674,#20675,#20676,#20677,#20678,#20679,#20680,#20681,
#20682,#20683,#20684,#20685,#20686,#20687,#20688,#20689,#20690,#20691,#20692,
#20693,#20694,#20695,#20696,#20697,#20698,#20699,#20700,#20701,#20702,#20703,
#20704,#20705,#20706,#20707,#20708,#20709,#20710,#20711,#20712,#20713,#20714,
#20715,#20716,#20717,#20718,#20719,#20720,#20721,#20722,#20723,#20724,#20725,
#20726,#20727,#20728,#20729,#20730,#20731,#20732,#20733,#20734,#20735,#20736,
#20737,#20738,#20739,#20740,#20741,#20742,#20743,#20744,#20745,#20746,#20747,
#20748,#20749,#20750,#20751,#20752,#20753,#20754,#20755,#20756,#20757,#20758,
#20759,#20760,#20761,#20762,#20763,#20764,#20765,#20766,#20767,#20768,#20769,
#20770,#20771,#20772,#20773,#20774,#20775,#20776,#20777,#20778,#20779,#20780,
#20781,#20782,#20783),(#20784,#20785,#20786,#20787,#20788,#20789,#20790,
#20791,#20792,#20793,#20794,#20795,#20796,#20797,#20798,#20799,#20800,#20801,
#20802,#20803,#20804,#20805,#20806,#20807,#20808,#20809,#20810,#20811,#20812,
#20813,#20814,#20815,#20816,#20817,#20818,#20819,#20820,#20821,#20822,#20823,
#20824,#20825,#20826,#20827,#20828,#20829,#20830,#20831,#20832,#20833,#20834,
#20835,#20836,#20837,#20838,#20839,#20840,#20841,#20842,#20843,#20844,#20845,
#20846,#20847,#20848,#20849,#20850,#20851,#20852,#20853,#20854,#20855,#20856,
#20857,#20858,#20859,#20860,#20861,#20862,#20863,#20864,#20865,#20866,#20867,
#20868,#20869,#20870,#20871,#20872,#20873,#20874,#20875,#20876,#20877,#20878,
#20879,#20880,#20881,#20882,#20883,#20884,#20885,#20886,#20887,#20888,#20889,
#20890,#20891,#20892,#20893,#20894,#20895)),.UNSPECIFIED.,.F.,.F.,.F.,(4,
4),(4,1,1,1,1,1,1,1,1,1,1,1,1,1,1,1,1,1,1,1,1,1,1,1,1,1,1,1,1,1,1,1,1,1,
1,1,1,1,1,1,1,1,1,1,1,1,1,1,1,1,1,1,1,1,1,1,1,1,1,1,1,1,1,1,1,1,1,1,1,1,
1,1,1,1,1,1,1,1,1,1,1,1,1,1,1,1,1,1,1,1,1,1,1,1,1,1,1,1,1,1,1,1,1,1,1,1,
1,1,1,4),(0.,0.064201349933888),(11.8589888623077,12.8574392762076,13.8558896901074,
14.8543401040072,15.852790517907,16.8512409318069,17.8496913457067,18.8481417596065,
19.8465921735064,20.8450425874062,21.843493001306,22.8419434152059,23.8403938291057,
24.8388442430055,25.8372946569053,26.8357450708052,27.834195484705,28.8326458986048,
29.8310963125047,30.8295467264045,31.8279971403043,32.8264475542042,33.824897968104,
34.8233483820038,35.8217987959036,36.8202492098035,37.8186996237033,38.8171500376031,
39.815600451503,40.8140508654028,41.8125012793026,42.8109516932024,43.8094021071023,
44.8078525210021,45.8063029349019,46.8047533488018,47.8032037627016,48.8016541766014,
49.8001045905012,50.7985550044011,51.7970054183009,52.7954558322007,53.7939062461006,
54.7923566600004,55.7908070739002,56.7892574878001,57.7877079016999,58.7861583155997,
59.7846087294995,60.7830591433994,61.7815095572992,62.779959971199,63.7784103850989,
64.7768607989987,65.7753112128985,66.7737616267983,67.7722120406982,68.770662454598,
69.7691128684978,70.7675632823977,71.7660136962975,72.7644641101973,73.7629145240972,
74.761364937997,75.7598153518968,76.7582657657966,77.7567161796965,78.7551665935963,
79.7536170074961,80.7520674213959,81.7505178352958,82.7489682491956,83.7474186630954,
84.7458690769953,85.7443194908951,86.7427699047949,87.7412203186948,88.7396707325946,
89.7381211464944,90.7365715603942,91.7350219742941,92.7334723881939,93.7319228020937,
94.7303732159936,95.7288236298934,96.7272740437932,97.725724457693,98.7241748715929,
99.7226252854927,100.721075699393,101.719526113292,102.717976527192,103.716426941092,
104.714877354992,105.713327768892,106.711778182792,107.710228596691,108.708679010591,
109.707129424491,110.705579838391,111.704030252291,112.70248066619,113.70093108009,
114.69938149399,115.69783190789,116.69628232179,117.69473273569,118.693183149589,
119.691633563489,120.690083977389),.UNSPECIFIED.);
#300=B_SPLINE_SURFACE_WITH_KNOTS('',3,3,((#21018,#21019,#21020,#21021,#21022,
#21023,#21024,#21025,#21026,#21027,#21028,#21029,#21030,#21031,#21032,#21033,
#21034,#21035,#21036,#21037,#21038,#21039,#21040,#21041,#21042,#21043,#21044,
#21045,#21046,#21047,#21048,#21049,#21050,#21051,#21052,#21053,#21054,#21055,
#21056,#21057,#21058,#21059,#21060,#21061,#21062,#21063,#21064,#21065,#21066,
#21067,#21068,#21069,#21070,#21071,#21072,#21073,#21074,#21075,#21076,#21077,
#21078,#21079,#21080,#21081,#21082,#21083,#21084,#21085,#21086,#21087,#21088,
#21089,#21090,#21091,#21092,#21093,#21094,#21095,#21096,#21097,#21098,#21099,
#21100,#21101,#21102,#21103,#21104,#21105,#21106,#21107,#21108,#21109,#21110,
#21111,#21112,#21113,#21114,#21115,#21116,#21117,#21118,#21119,#21120,#21121,
#21122,#21123,#21124,#21125,#21126,#21127,#21128,#21129),(#21130,#21131,
#21132,#21133,#21134,#21135,#21136,#21137,#21138,#21139,#21140,#21141,#21142,
#21143,#21144,#21145,#21146,#21147,#21148,#21149,#21150,#21151,#21152,#21153,
#21154,#21155,#21156,#21157,#21158,#21159,#21160,#21161,#21162,#21163,#21164,
#21165,#21166,#21167,#21168,#21169,#21170,#21171,#21172,#21173,#21174,#21175,
#21176,#21177,#21178,#21179,#21180,#21181,#21182,#21183,#21184,#21185,#21186,
#21187,#21188,#21189,#21190,#21191,#21192,#21193,#21194,#21195,#21196,#21197,
#21198,#21199,#21200,#21201,#21202,#21203,#21204,#21205,#21206,#21207,#21208,
#21209,#21210,#21211,#21212,#21213,#21214,#21215,#21216,#21217,#21218,#21219,
#21220,#21221,#21222,#21223,#21224,#21225,#21226,#21227,#21228,#21229,#21230,
#21231,#21232,#21233,#21234,#21235,#21236,#21237,#21238,#21239,#21240,#21241),
(#21242,#21243,#21244,#21245,#21246,#21247,#21248,#21249,#21250,#21251,
#21252,#21253,#21254,#21255,#21256,#21257,#21258,#21259,#21260,#21261,#21262,
#21263,#21264,#21265,#21266,#21267,#21268,#21269,#21270,#21271,#21272,#21273,
#21274,#21275,#21276,#21277,#21278,#21279,#21280,#21281,#21282,#21283,#21284,
#21285,#21286,#21287,#21288,#21289,#21290,#21291,#21292,#21293,#21294,#21295,
#21296,#21297,#21298,#21299,#21300,#21301,#21302,#21303,#21304,#21305,#21306,
#21307,#21308,#21309,#21310,#21311,#21312,#21313,#21314,#21315,#21316,#21317,
#21318,#21319,#21320,#21321,#21322,#21323,#21324,#21325,#21326,#21327,#21328,
#21329,#21330,#21331,#21332,#21333,#21334,#21335,#21336,#21337,#21338,#21339,
#21340,#21341,#21342,#21343,#21344,#21345,#21346,#21347,#21348,#21349,#21350,
#21351,#21352,#21353),(#21354,#21355,#21356,#21357,#21358,#21359,#21360,
#21361,#21362,#21363,#21364,#21365,#21366,#21367,#21368,#21369,#21370,#21371,
#21372,#21373,#21374,#21375,#21376,#21377,#21378,#21379,#21380,#21381,#21382,
#21383,#21384,#21385,#21386,#21387,#21388,#21389,#21390,#21391,#21392,#21393,
#21394,#21395,#21396,#21397,#21398,#21399,#21400,#21401,#21402,#21403,#21404,
#21405,#21406,#21407,#21408,#21409,#21410,#21411,#21412,#21413,#21414,#21415,
#21416,#21417,#21418,#21419,#21420,#21421,#21422,#21423,#21424,#21425,#21426,
#21427,#21428,#21429,#21430,#21431,#21432,#21433,#21434,#21435,#21436,#21437,
#21438,#21439,#21440,#21441,#21442,#21443,#21444,#21445,#21446,#21447,#21448,
#21449,#21450,#21451,#21452,#21453,#21454,#21455,#21456,#21457,#21458,#21459,
#21460,#21461,#21462,#21463,#21464,#21465)),.UNSPECIFIED.,.F.,.F.,.F.,(4,
4),(4,1,1,1,1,1,1,1,1,1,1,1,1,1,1,1,1,1,1,1,1,1,1,1,1,1,1,1,1,1,1,1,1,1,
1,1,1,1,1,1,1,1,1,1,1,1,1,1,1,1,1,1,1,1,1,1,1,1,1,1,1,1,1,1,1,1,1,1,1,1,
1,1,1,1,1,1,1,1,1,1,1,1,1,1,1,1,1,1,1,1,1,1,1,1,1,1,1,1,1,1,1,1,1,1,1,1,
1,1,1,4),(0.,0.064201349933888),(14.3984001269718,15.3968505408716,16.3953009547714,
17.3937513686712,18.3922017825711,19.3906521964709,20.3891026103707,21.3875530242706,
22.3860034381704,23.3844538520702,24.38290426597,25.3813546798699,26.3798050937697,
27.3782555076695,28.3767059215694,29.3751563354692,30.373606749369,31.3720571632689,
32.3705075771687,33.3689579910685,34.3674084049683,35.3658588188682,36.364309232768,
37.3627596466678,38.3612100605677,39.3596604744675,40.3581108883673,41.3565613022671,
42.355011716167,43.3534621300668,44.3519125439666,45.3503629578665,46.3488133717663,
47.3472637856661,48.345714199566,49.3441646134658,50.3426150273656,51.3410654412654,
52.3395158551653,53.3379662690651,54.3364166829649,55.3348670968648,56.3333175107646,
57.3317679246644,58.3302183385643,59.3286687524641,60.3271191663639,61.3255695802637,
62.3240199941636,63.3224704080634,64.3209208219632,65.3193712358631,66.3178216497629,
67.3162720636627,68.3147224775625,69.3131728914624,70.3116233053622,71.310073719262,
72.3085241331619,73.3069745470617,74.3054249609615,75.3038753748613,76.3023257887612,
77.300776202661,78.2992266165608,79.2976770304607,80.2961274443605,81.2945778582603,
82.2930282721602,83.29147868606,84.2899290999598,85.2883795138596,86.2868299277595,
87.2852803416593,88.2837307555591,89.282181169459,90.2806315833588,91.2790819972586,
92.2775324111584,93.2759828250583,94.2744332389581,95.2728836528579,96.2713340667578,
97.2697844806576,98.2682348945574,99.2666853084573,100.265135722357,101.263586136257,
102.262036550157,103.260486964057,104.258937377956,105.257387791856,106.255838205756,
107.254288619656,108.252739033556,109.251189447456,110.249639861355,111.248090275255,
112.246540689155,113.244991103055,114.243441516955,115.241891930855,116.240342344754,
117.238792758654,118.237243172554,119.235693586454,120.234144000354,121.232594414253,
122.231044828153,123.229495242053),.UNSPECIFIED.);
#311=PLANE('',#9054);
#312=PLANE('',#9057);
#313=PLANE('',#9060);
#314=PLANE('',#9063);
#315=PLANE('',#9066);
#316=PLANE('',#9067);
#317=PLANE('',#9068);
#318=PLANE('',#9069);
#319=PLANE('',#9070);
#320=PLANE('',#9071);
#321=PLANE('',#9072);
#322=PLANE('',#9073);
#323=PLANE('',#9074);
#324=PLANE('',#9075);
#325=PLANE('',#9076);
#326=PLANE('',#9077);
#327=PLANE('',#9078);
#328=PLANE('',#9079);
#452=FACE_OUTER_BOUND('',#927,.T.);
#453=FACE_OUTER_BOUND('',#928,.T.);
#454=FACE_OUTER_BOUND('',#929,.T.);
#455=FACE_OUTER_BOUND('',#930,.T.);
#456=FACE_OUTER_BOUND('',#931,.T.);
#457=FACE_OUTER_BOUND('',#932,.T.);
#458=FACE_OUTER_BOUND('',#933,.T.);
#459=FACE_OUTER_BOUND('',#934,.T.);
#460=FACE_OUTER_BOUND('',#935,.T.);
#461=FACE_OUTER_BOUND('',#936,.T.);
#462=FACE_OUTER_BOUND('',#937,.T.);
#463=FACE_OUTER_BOUND('',#938,.T.);
#464=FACE_OUTER_BOUND('',#939,.T.);
#465=FACE_OUTER_BOUND('',#940,.T.);
#466=FACE_OUTER_BOUND('',#941,.T.);
#467=FACE_OUTER_BOUND('',#942,.T.);
#468=FACE_OUTER_BOUND('',#943,.T.);
#469=FACE_OUTER_BOUND('',#944,.T.);
#470=FACE_OUTER_BOUND('',#945,.T.);
#471=FACE_OUTER_BOUND('',#946,.T.);
#472=FACE_OUTER_BOUND('',#947,.T.);
#473=FACE_OUTER_BOUND('',#948,.T.);
#474=FACE_OUTER_BOUND('',#949,.T.);
#475=FACE_OUTER_BOUND('',#950,.T.);
#476=FACE_OUTER_BOUND('',#951,.T.);
#477=FACE_OUTER_BOUND('',#952,.T.);
#478=FACE_OUTER_BOUND('',#953,.T.);
#479=FACE_OUTER_BOUND('',#954,.T.);
#480=FACE_OUTER_BOUND('',#955,.T.);
#481=FACE_OUTER_BOUND('',#956,.T.);
#482=FACE_OUTER_BOUND('',#957,.T.);
#483=FACE_OUTER_BOUND('',#958,.T.);
#484=FACE_OUTER_BOUND('',#959,.T.);
#485=FACE_OUTER_BOUND('',#960,.T.);
#486=FACE_OUTER_BOUND('',#961,.T.);
#487=FACE_OUTER_BOUND('',#962,.T.);
#488=FACE_OUTER_BOUND('',#963,.T.);
#489=FACE_OUTER_BOUND('',#964,.T.);
#490=FACE_OUTER_BOUND('',#965,.T.);
#491=FACE_OUTER_BOUND('',#966,.T.);
#492=FACE_OUTER_BOUND('',#967,.T.);
#493=FACE_OUTER_BOUND('',#968,.T.);
#494=FACE_OUTER_BOUND('',#969,.T.);
#495=FACE_OUTER_BOUND('',#970,.T.);
#496=FACE_OUTER_BOUND('',#971,.T.);
#497=FACE_OUTER_BOUND('',#972,.T.);
#498=FACE_OUTER_BOUND('',#973,.T.);
#499=FACE_OUTER_BOUND('',#974,.T.);
#500=FACE_OUTER_BOUND('',#975,.T.);
#501=FACE_OUTER_BOUND('',#976,.T.);
#502=FACE_OUTER_BOUND('',#977,.T.);
#503=FACE_OUTER_BOUND('',#978,.T.);
#504=FACE_OUTER_BOUND('',#979,.T.);
#505=FACE_OUTER_BOUND('',#980,.T.);
#506=FACE_OUTER_BOUND('',#981,.T.);
#507=FACE_OUTER_BOUND('',#982,.T.);
#508=FACE_OUTER_BOUND('',#983,.T.);
#509=FACE_OUTER_BOUND('',#984,.T.);
#510=FACE_OUTER_BOUND('',#985,.T.);
#511=FACE_OUTER_BOUND('',#986,.T.);
#512=FACE_OUTER_BOUND('',#987,.T.);
#513=FACE_OUTER_BOUND('',#988,.T.);
#514=FACE_OUTER_BOUND('',#989,.T.);
#515=FACE_OUTER_BOUND('',#990,.T.);
#516=FACE_OUTER_BOUND('',#991,.T.);
#517=FACE_OUTER_BOUND('',#992,.T.);
#518=FACE_OUTER_BOUND('',#993,.T.);
#519=FACE_OUTER_BOUND('',#994,.T.);
#520=FACE_OUTER_BOUND('',#995,.T.);
#521=FACE_OUTER_BOUND('',#996,.T.);
#522=FACE_OUTER_BOUND('',#997,.T.);
#523=FACE_OUTER_BOUND('',#998,.T.);
#524=FACE_OUTER_BOUND('',#999,.T.);
#525=FACE_OUTER_BOUND('',#1000,.T.);
#526=FACE_OUTER_BOUND('',#1001,.T.);
#527=FACE_OUTER_BOUND('',#1002,.T.);
#528=FACE_OUTER_BOUND('',#1003,.T.);
#529=FACE_OUTER_BOUND('',#1004,.T.);
#530=FACE_OUTER_BOUND('',#1005,.T.);
#531=FACE_OUTER_BOUND('',#1006,.T.);
#532=FACE_OUTER_BOUND('',#1007,.T.);
#533=FACE_OUTER_BOUND('',#1008,.T.);
#534=FACE_OUTER_BOUND('',#1009,.T.);
#535=FACE_OUTER_BOUND('',#1010,.T.);
#536=FACE_OUTER_BOUND('',#1011,.T.);
#537=FACE_OUTER_BOUND('',#1012,.T.);
#538=FACE_OUTER_BOUND('',#1013,.T.);
#539=FACE_OUTER_BOUND('',#1014,.T.);
#540=FACE_OUTER_BOUND('',#1015,.T.);
#541=FACE_OUTER_BOUND('',#1016,.T.);
#542=FACE_OUTER_BOUND('',#1017,.T.);
#543=FACE_OUTER_BOUND('',#1018,.T.);
#544=FACE_OUTER_BOUND('',#1019,.T.);
#545=FACE_OUTER_BOUND('',#1020,.T.);
#546=FACE_OUTER_BOUND('',#1021,.T.);
#547=FACE_OUTER_BOUND('',#1022,.T.);
#548=FACE_OUTER_BOUND('',#1023,.T.);
#549=FACE_OUTER_BOUND('',#1024,.T.);
#550=FACE_OUTER_BOUND('',#1025,.T.);
#551=FACE_OUTER_BOUND('',#1026,.T.);
#552=FACE_OUTER_BOUND('',#1027,.T.);
#553=FACE_OUTER_BOUND('',#1028,.T.);
#554=FACE_OUTER_BOUND('',#1029,.T.);
#555=FACE_OUTER_BOUND('',#1030,.T.);
#556=FACE_OUTER_BOUND('',#1031,.T.);
#557=FACE_OUTER_BOUND('',#1032,.T.);
#558=FACE_OUTER_BOUND('',#1033,.T.);
#559=FACE_OUTER_BOUND('',#1034,.T.);
#560=FACE_OUTER_BOUND('',#1035,.T.);
#561=FACE_OUTER_BOUND('',#1036,.T.);
#562=FACE_OUTER_BOUND('',#1037,.T.);
#563=FACE_OUTER_BOUND('',#1038,.T.);
#564=FACE_OUTER_BOUND('',#1039,.T.);
#565=FACE_OUTER_BOUND('',#1040,.T.);
#566=FACE_OUTER_BOUND('',#1041,.T.);
#567=FACE_OUTER_BOUND('',#1042,.T.);
#568=FACE_OUTER_BOUND('',#1043,.T.);
#569=FACE_OUTER_BOUND('',#1044,.T.);
#570=FACE_OUTER_BOUND('',#1045,.T.);
#571=FACE_OUTER_BOUND('',#1046,.T.);
#572=FACE_OUTER_BOUND('',#1047,.T.);
#573=FACE_OUTER_BOUND('',#1048,.T.);
#574=FACE_OUTER_BOUND('',#1049,.T.);
#575=FACE_OUTER_BOUND('',#1050,.T.);
#576=FACE_OUTER_BOUND('',#1051,.T.);
#577=FACE_OUTER_BOUND('',#1052,.T.);
#578=FACE_OUTER_BOUND('',#1053,.T.);
#579=FACE_OUTER_BOUND('',#1054,.T.);
#580=FACE_OUTER_BOUND('',#1055,.T.);
#581=FACE_OUTER_BOUND('',#1056,.T.);
#582=FACE_OUTER_BOUND('',#1057,.T.);
#583=FACE_OUTER_BOUND('',#1058,.T.);
#584=FACE_OUTER_BOUND('',#1059,.T.);
#585=FACE_OUTER_BOUND('',#1060,.T.);
#586=FACE_OUTER_BOUND('',#1061,.T.);
#587=FACE_OUTER_BOUND('',#1062,.T.);
#588=FACE_OUTER_BOUND('',#1063,.T.);
#589=FACE_OUTER_BOUND('',#1064,.T.);
#590=FACE_OUTER_BOUND('',#1065,.T.);
#591=FACE_OUTER_BOUND('',#1066,.T.);
#592=FACE_OUTER_BOUND('',#1067,.T.);
#593=FACE_OUTER_BOUND('',#1068,.T.);
#594=FACE_OUTER_BOUND('',#1069,.T.);
#595=FACE_OUTER_BOUND('',#1070,.T.);
#596=FACE_OUTER_BOUND('',#1071,.T.);
#597=FACE_OUTER_BOUND('',#1072,.T.);
#598=FACE_OUTER_BOUND('',#1073,.T.);
#599=FACE_OUTER_BOUND('',#1074,.T.);
#600=FACE_OUTER_BOUND('',#1075,.T.);
#601=FACE_OUTER_BOUND('',#1076,.T.);
#602=FACE_OUTER_BOUND('',#1077,.T.);
#603=FACE_OUTER_BOUND('',#1078,.T.);
#604=FACE_OUTER_BOUND('',#1079,.T.);
#605=FACE_OUTER_BOUND('',#1080,.T.);
#606=FACE_OUTER_BOUND('',#1081,.T.);
#607=FACE_OUTER_BOUND('',#1082,.T.);
#608=FACE_OUTER_BOUND('',#1083,.T.);
#609=FACE_OUTER_BOUND('',#1084,.T.);
#610=FACE_OUTER_BOUND('',#1085,.T.);
#611=FACE_OUTER_BOUND('',#1086,.T.);
#612=FACE_OUTER_BOUND('',#1087,.T.);
#613=FACE_OUTER_BOUND('',#1088,.T.);
#614=FACE_OUTER_BOUND('',#1089,.T.);
#615=FACE_OUTER_BOUND('',#1090,.T.);
#616=FACE_OUTER_BOUND('',#1091,.T.);
#617=FACE_OUTER_BOUND('',#1092,.T.);
#618=FACE_OUTER_BOUND('',#1093,.T.);
#619=FACE_OUTER_BOUND('',#1094,.T.);
#620=FACE_OUTER_BOUND('',#1095,.T.);
#621=FACE_OUTER_BOUND('',#1097,.T.);
#927=EDGE_LOOP('',(#5367,#5368,#5369,#5370,#5371,#5372,#5373,#5374));
#928=EDGE_LOOP('',(#5375,#5376,#5377,#5378));
#929=EDGE_LOOP('',(#5379,#5380,#5381,#5382));
#930=EDGE_LOOP('',(#5383,#5384,#5385,#5386));
#931=EDGE_LOOP('',(#5387,#5388,#5389,#5390));
#932=EDGE_LOOP('',(#5391,#5392,#5393,#5394));
#933=EDGE_LOOP('',(#5395,#5396,#5397,#5398));
#934=EDGE_LOOP('',(#5399,#5400,#5401,#5402));
#935=EDGE_LOOP('',(#5403,#5404,#5405,#5406));
#936=EDGE_LOOP('',(#5407,#5408,#5409,#5410));
#937=EDGE_LOOP('',(#5411,#5412,#5413,#5414));
#938=EDGE_LOOP('',(#5415,#5416,#5417,#5418));
#939=EDGE_LOOP('',(#5419,#5420,#5421,#5422));
#940=EDGE_LOOP('',(#5423,#5424,#5425,#5426));
#941=EDGE_LOOP('',(#5427,#5428,#5429,#5430));
#942=EDGE_LOOP('',(#5431,#5432,#5433,#5434));
#943=EDGE_LOOP('',(#5435,#5436,#5437,#5438));
#944=EDGE_LOOP('',(#5439,#5440,#5441,#5442));
#945=EDGE_LOOP('',(#5443,#5444,#5445,#5446));
#946=EDGE_LOOP('',(#5447,#5448,#5449,#5450));
#947=EDGE_LOOP('',(#5451,#5452,#5453,#5454));
#948=EDGE_LOOP('',(#5455,#5456,#5457,#5458));
#949=EDGE_LOOP('',(#5459,#5460,#5461,#5462));
#950=EDGE_LOOP('',(#5463,#5464,#5465,#5466));
#951=EDGE_LOOP('',(#5467,#5468,#5469,#5470));
#952=EDGE_LOOP('',(#5471,#5472,#5473,#5474));
#953=EDGE_LOOP('',(#5475,#5476,#5477,#5478));
#954=EDGE_LOOP('',(#5479,#5480,#5481,#5482));
#955=EDGE_LOOP('',(#5483,#5484,#5485,#5486));
#956=EDGE_LOOP('',(#5487,#5488,#5489,#5490));
#957=EDGE_LOOP('',(#5491,#5492,#5493,#5494));
#958=EDGE_LOOP('',(#5495,#5496,#5497,#5498));
#959=EDGE_LOOP('',(#5499,#5500,#5501,#5502));
#960=EDGE_LOOP('',(#5503,#5504,#5505,#5506));
#961=EDGE_LOOP('',(#5507,#5508,#5509,#5510,#5511,#5512,#5513,#5514));
#962=EDGE_LOOP('',(#5515,#5516,#5517,#5518));
#963=EDGE_LOOP('',(#5519,#5520,#5521,#5522));
#964=EDGE_LOOP('',(#5523,#5524,#5525,#5526));
#965=EDGE_LOOP('',(#5527,#5528,#5529,#5530));
#966=EDGE_LOOP('',(#5531,#5532,#5533,#5534));
#967=EDGE_LOOP('',(#5535,#5536,#5537,#5538));
#968=EDGE_LOOP('',(#5539,#5540,#5541,#5542));
#969=EDGE_LOOP('',(#5543,#5544,#5545,#5546));
#970=EDGE_LOOP('',(#5547,#5548,#5549,#5550));
#971=EDGE_LOOP('',(#5551,#5552,#5553,#5554));
#972=EDGE_LOOP('',(#5555,#5556,#5557,#5558));
#973=EDGE_LOOP('',(#5559,#5560,#5561,#5562));
#974=EDGE_LOOP('',(#5563,#5564,#5565,#5566));
#975=EDGE_LOOP('',(#5567,#5568,#5569,#5570));
#976=EDGE_LOOP('',(#5571,#5572,#5573,#5574));
#977=EDGE_LOOP('',(#5575,#5576,#5577,#5578));
#978=EDGE_LOOP('',(#5579,#5580,#5581,#5582));
#979=EDGE_LOOP('',(#5583,#5584,#5585,#5586));
#980=EDGE_LOOP('',(#5587,#5588,#5589,#5590));
#981=EDGE_LOOP('',(#5591,#5592,#5593,#5594));
#982=EDGE_LOOP('',(#5595,#5596,#5597,#5598));
#983=EDGE_LOOP('',(#5599,#5600,#5601,#5602));
#984=EDGE_LOOP('',(#5603,#5604,#5605,#5606));
#985=EDGE_LOOP('',(#5607,#5608,#5609,#5610));
#986=EDGE_LOOP('',(#5611,#5612,#5613,#5614));
#987=EDGE_LOOP('',(#5615,#5616,#5617,#5618));
#988=EDGE_LOOP('',(#5619,#5620,#5621,#5622));
#989=EDGE_LOOP('',(#5623,#5624,#5625,#5626));
#990=EDGE_LOOP('',(#5627,#5628,#5629,#5630));
#991=EDGE_LOOP('',(#5631,#5632,#5633,#5634));
#992=EDGE_LOOP('',(#5635,#5636,#5637,#5638));
#993=EDGE_LOOP('',(#5639,#5640,#5641,#5642));
#994=EDGE_LOOP('',(#5643,#5644,#5645,#5646));
#995=EDGE_LOOP('',(#5647,#5648,#5649,#5650,#5651,#5652,#5653,#5654));
#996=EDGE_LOOP('',(#5655,#5656,#5657,#5658));
#997=EDGE_LOOP('',(#5659,#5660,#5661,#5662));
#998=EDGE_LOOP('',(#5663,#5664,#5665,#5666));
#999=EDGE_LOOP('',(#5667,#5668,#5669,#5670));
#1000=EDGE_LOOP('',(#5671,#5672,#5673,#5674));
#1001=EDGE_LOOP('',(#5675,#5676,#5677,#5678));
#1002=EDGE_LOOP('',(#5679,#5680,#5681,#5682));
#1003=EDGE_LOOP('',(#5683,#5684,#5685,#5686));
#1004=EDGE_LOOP('',(#5687,#5688,#5689,#5690));
#1005=EDGE_LOOP('',(#5691,#5692,#5693,#5694));
#1006=EDGE_LOOP('',(#5695,#5696,#5697,#5698));
#1007=EDGE_LOOP('',(#5699,#5700,#5701,#5702));
#1008=EDGE_LOOP('',(#5703,#5704,#5705,#5706));
#1009=EDGE_LOOP('',(#5707,#5708,#5709,#5710));
#1010=EDGE_LOOP('',(#5711,#5712,#5713,#5714));
#1011=EDGE_LOOP('',(#5715,#5716,#5717,#5718));
#1012=EDGE_LOOP('',(#5719,#5720,#5721,#5722));
#1013=EDGE_LOOP('',(#5723,#5724,#5725,#5726));
#1014=EDGE_LOOP('',(#5727,#5728,#5729,#5730));
#1015=EDGE_LOOP('',(#5731,#5732,#5733,#5734));
#1016=EDGE_LOOP('',(#5735,#5736,#5737,#5738));
#1017=EDGE_LOOP('',(#5739,#5740,#5741,#5742));
#1018=EDGE_LOOP('',(#5743,#5744,#5745,#5746));
#1019=EDGE_LOOP('',(#5747,#5748,#5749,#5750));
#1020=EDGE_LOOP('',(#5751,#5752,#5753,#5754));
#1021=EDGE_LOOP('',(#5755,#5756,#5757,#5758));
#1022=EDGE_LOOP('',(#5759,#5760,#5761,#5762));
#1023=EDGE_LOOP('',(#5763,#5764,#5765,#5766));
#1024=EDGE_LOOP('',(#5767,#5768,#5769,#5770));
#1025=EDGE_LOOP('',(#5771,#5772,#5773,#5774));
#1026=EDGE_LOOP('',(#5775,#5776,#5777,#5778));
#1027=EDGE_LOOP('',(#5779,#5780,#5781,#5782));
#1028=EDGE_LOOP('',(#5783,#5784,#5785,#5786));
#1029=EDGE_LOOP('',(#5787,#5788,#5789,#5790,#5791,#5792,#5793,#5794));
#1030=EDGE_LOOP('',(#5795,#5796,#5797,#5798));
#1031=EDGE_LOOP('',(#5799,#5800,#5801,#5802));
#1032=EDGE_LOOP('',(#5803,#5804,#5805,#5806));
#1033=EDGE_LOOP('',(#5807,#5808,#5809,#5810));
#1034=EDGE_LOOP('',(#5811,#5812,#5813,#5814));
#1035=EDGE_LOOP('',(#5815,#5816,#5817,#5818));
#1036=EDGE_LOOP('',(#5819,#5820,#5821,#5822));
#1037=EDGE_LOOP('',(#5823,#5824,#5825,#5826));
#1038=EDGE_LOOP('',(#5827,#5828,#5829,#5830));
#1039=EDGE_LOOP('',(#5831,#5832,#5833,#5834));
#1040=EDGE_LOOP('',(#5835,#5836,#5837,#5838));
#1041=EDGE_LOOP('',(#5839,#5840,#5841,#5842));
#1042=EDGE_LOOP('',(#5843,#5844,#5845,#5846));
#1043=EDGE_LOOP('',(#5847,#5848,#5849,#5850));
#1044=EDGE_LOOP('',(#5851,#5852,#5853,#5854));
#1045=EDGE_LOOP('',(#5855,#5856,#5857,#5858));
#1046=EDGE_LOOP('',(#5859,#5860,#5861,#5862));
#1047=EDGE_LOOP('',(#5863,#5864,#5865,#5866));
#1048=EDGE_LOOP('',(#5867,#5868,#5869,#5870));
#1049=EDGE_LOOP('',(#5871,#5872,#5873,#5874));
#1050=EDGE_LOOP('',(#5875,#5876,#5877,#5878));
#1051=EDGE_LOOP('',(#5879,#5880,#5881,#5882));
#1052=EDGE_LOOP('',(#5883,#5884,#5885,#5886));
#1053=EDGE_LOOP('',(#5887,#5888,#5889,#5890));
#1054=EDGE_LOOP('',(#5891,#5892,#5893,#5894));
#1055=EDGE_LOOP('',(#5895,#5896,#5897,#5898));
#1056=EDGE_LOOP('',(#5899,#5900,#5901,#5902));
#1057=EDGE_LOOP('',(#5903,#5904,#5905,#5906));
#1058=EDGE_LOOP('',(#5907,#5908,#5909,#5910));
#1059=EDGE_LOOP('',(#5911,#5912,#5913,#5914));
#1060=EDGE_LOOP('',(#5915,#5916,#5917,#5918));
#1061=EDGE_LOOP('',(#5919,#5920,#5921,#5922));
#1062=EDGE_LOOP('',(#5923,#5924,#5925,#5926));
#1063=EDGE_LOOP('',(#5927,#5928,#5929,#5930,#5931));
#1064=EDGE_LOOP('',(#5932,#5933,#5934,#5935));
#1065=EDGE_LOOP('',(#5936,#5937,#5938,#5939,#5940,#5941,#5942,#5943,#5944,
#5945,#5946,#5947,#5948,#5949,#5950,#5951,#5952,#5953,#5954,#5955,#5956,
#5957,#5958,#5959,#5960,#5961,#5962,#5963,#5964,#5965,#5966,#5967,#5968,
#5969,#5970,#5971,#5972,#5973));
#1066=EDGE_LOOP('',(#5974,#5975,#5976,#5977,#5978,#5979,#5980,#5981,#5982,
#5983,#5984,#5985,#5986,#5987,#5988,#5989,#5990,#5991,#5992,#5993,#5994,
#5995,#5996,#5997,#5998,#5999,#6000,#6001,#6002,#6003,#6004,#6005,#6006,
#6007,#6008,#6009,#6010,#6011));
#1067=EDGE_LOOP('',(#6012,#6013,#6014,#6015));
#1068=EDGE_LOOP('',(#6016,#6017,#6018,#6019,#6020));
#1069=EDGE_LOOP('',(#6021,#6022,#6023,#6024));
#1070=EDGE_LOOP('',(#6025,#6026,#6027,#6028,#6029,#6030,#6031,#6032,#6033,
#6034,#6035,#6036,#6037,#6038,#6039,#6040,#6041,#6042,#6043,#6044,#6045,
#6046,#6047,#6048,#6049,#6050,#6051,#6052,#6053,#6054,#6055,#6056,#6057,
#6058,#6059,#6060,#6061,#6062));
#1071=EDGE_LOOP('',(#6063,#6064,#6065,#6066,#6067,#6068,#6069,#6070,#6071,
#6072,#6073,#6074,#6075,#6076,#6077,#6078,#6079,#6080,#6081,#6082,#6083,
#6084,#6085,#6086,#6087,#6088,#6089,#6090,#6091,#6092,#6093,#6094,#6095,
#6096,#6097,#6098,#6099,#6100));
#1072=EDGE_LOOP('',(#6101,#6102,#6103,#6104));
#1073=EDGE_LOOP('',(#6105,#6106,#6107,#6108,#6109));
#1074=EDGE_LOOP('',(#6110,#6111,#6112,#6113));
#1075=EDGE_LOOP('',(#6114,#6115,#6116,#6117,#6118,#6119,#6120,#6121,#6122,
#6123,#6124,#6125,#6126,#6127,#6128,#6129,#6130,#6131,#6132,#6133,#6134,
#6135,#6136,#6137,#6138,#6139,#6140,#6141,#6142,#6143,#6144,#6145,#6146,
#6147,#6148,#6149,#6150,#6151));
#1076=EDGE_LOOP('',(#6152,#6153,#6154,#6155,#6156,#6157,#6158,#6159,#6160,
#6161,#6162,#6163,#6164,#6165,#6166,#6167,#6168,#6169,#6170,#6171,#6172,
#6173,#6174,#6175,#6176,#6177,#6178,#6179,#6180,#6181,#6182,#6183,#6184,
#6185,#6186,#6187,#6188,#6189));
#1077=EDGE_LOOP('',(#6190,#6191,#6192,#6193));
#1078=EDGE_LOOP('',(#6194,#6195,#6196,#6197,#6198));
#1079=EDGE_LOOP('',(#6199,#6200,#6201,#6202));
#1080=EDGE_LOOP('',(#6203,#6204,#6205,#6206,#6207,#6208,#6209,#6210,#6211,
#6212,#6213,#6214,#6215,#6216,#6217,#6218,#6219,#6220,#6221,#6222,#6223,
#6224,#6225,#6226,#6227,#6228,#6229,#6230,#6231,#6232,#6233,#6234,#6235,
#6236,#6237,#6238,#6239,#6240));
#1081=EDGE_LOOP('',(#6241,#6242,#6243,#6244,#6245,#6246,#6247,#6248,#6249,
#6250,#6251,#6252,#6253,#6254,#6255,#6256,#6257,#6258,#6259,#6260,#6261,
#6262,#6263,#6264,#6265,#6266,#6267,#6268,#6269,#6270,#6271,#6272,#6273,
#6274,#6275,#6276,#6277,#6278));
#1082=EDGE_LOOP('',(#6279,#6280,#6281,#6282));
#1083=EDGE_LOOP('',(#6283));
#1084=EDGE_LOOP('',(#6284));
#1085=EDGE_LOOP('',(#6285));
#1086=EDGE_LOOP('',(#6286));
#1087=EDGE_LOOP('',(#6287,#6288,#6289,#6290));
#1088=EDGE_LOOP('',(#6291,#6292,#6293,#6294));
#1089=EDGE_LOOP('',(#6295,#6296,#6297,#6298));
#1090=EDGE_LOOP('',(#6299,#6300,#6301,#6302));
#1091=EDGE_LOOP('',(#6303,#6304,#6305,#6306));
#1092=EDGE_LOOP('',(#6307,#6308,#6309,#6310));
#1093=EDGE_LOOP('',(#6311,#6312,#6313,#6314));
#1094=EDGE_LOOP('',(#6315,#6316,#6317,#6318));
#1095=EDGE_LOOP('',(#6319,#6320,#6321,#6322));
#1096=EDGE_LOOP('',(#6323,#6324,#6325,#6326));
#1097=EDGE_LOOP('',(#6327,#6328,#6329,#6330));
#1098=EDGE_LOOP('',(#6331,#6332,#6333,#6334));
#1099=EDGE_LOOP('',(#6335,#6336,#6337,#6338));
#1100=EDGE_LOOP('',(#6339,#6340,#6341,#6342));
#1101=EDGE_LOOP('',(#6343,#6344,#6345,#6346));
#1102=EDGE_LOOP('',(#6347,#6348,#6349,#6350));
#1461=CIRCLE('',#8895,2.5175);
#1462=CIRCLE('',#8896,2.5175);
#1463=CIRCLE('',#8897,2.5175);
#1464=CIRCLE('',#8914,2.5175);
#1465=CIRCLE('',#8916,3.07349999999999);
#1466=CIRCLE('',#8933,3.0735);
#1467=CIRCLE('',#8935,2.5175);
#1468=CIRCLE('',#8936,2.5175);
#1469=CIRCLE('',#8937,2.5175);
#1470=CIRCLE('',#8954,2.5175);
#1471=CIRCLE('',#8956,3.07349999999999);
#1472=CIRCLE('',#8973,3.0735);
#1473=CIRCLE('',#8975,2.5175);
#1474=CIRCLE('',#8976,2.5175);
#1475=CIRCLE('',#8977,2.5175);
#1476=CIRCLE('',#8994,2.5175);
#1477=CIRCLE('',#8996,3.07349999999996);
#1478=CIRCLE('',#9013,3.07349999999996);
#1479=CIRCLE('',#9015,2.5175);
#1480=CIRCLE('',#9016,2.5175);
#1481=CIRCLE('',#9017,2.5175);
#1482=CIRCLE('',#9034,2.5175);
#1483=CIRCLE('',#9036,3.07350000000003);
#1484=CIRCLE('',#9053,3.07350000000003);
#1585=B_SPLINE_CURVE_WITH_KNOTS('',3,(#11356,#11357,#11358,#11359),
 .UNSPECIFIED.,.F.,.F.,(4,4),(108.12371336303,108.831095115081),
 .UNSPECIFIED.);
#1586=B_SPLINE_CURVE_WITH_KNOTS('',3,(#11367,#11368,#11369,#11370,#11371,
#11372,#11373,#11374,#11375,#11376),.UNSPECIFIED.,.F.,.F.,(4,3,3,4),(-106.814150222053,
-105.835743873382,-104.837293459482,-104.379939320515),.UNSPECIFIED.);
#1587=B_SPLINE_CURVE_WITH_KNOTS('',3,(#11381,#11382,#11383,#11384,#11385,
#11386,#11387,#11388,#11389,#11390,#11391,#11392,#11393,#11394,#11395,#11396,
#11397,#11398,#11399,#11400,#11401,#11402),.UNSPECIFIED.,.F.,.F.,(4,3,3,
3,3,3,3,4),(101.84052805585,102.840392631682,103.838843045582,104.837293459482,
105.835743873382,106.834194287282,107.832644701182,108.12371336303),
 .UNSPECIFIED.);
#1588=B_SPLINE_CURVE_WITH_KNOTS('',3,(#11403,#11404,#11405,#11406,#11407,
#11408,#11409,#11410,#11411,#11412,#11413,#11414,#11415,#11416,#11417,#11418,
#11419,#11420,#11421,#11422,#11423,#11424),.UNSPECIFIED.,.F.,.F.,(4,3,3,
3,3,3,3,4),(-104.379939320515,-103.838843045582,-102.840392631682,-101.841942217783,
-100.843491803883,-99.8450413899829,-98.8465909760831,-98.096754013335),
 .UNSPECIFIED.);
#1589=B_SPLINE_CURVE_WITH_KNOTS('',3,(#11429,#11430,#11431,#11432,#11433,
#11434,#11435,#11436,#11437,#11438,#11439,#11440,#11441,#11442,#11443,#11444,
#11445,#11446,#11447,#11448,#11449,#11450),.UNSPECIFIED.,.F.,.F.,(4,3,3,
3,3,3,3,4),(95.5573427486709,95.8512397343836,96.8496901482835,97.8481405621833,
98.8465909760831,99.845041389983,100.843491803883,101.84052805585),
 .UNSPECIFIED.);
#1590=B_SPLINE_CURVE_WITH_KNOTS('',3,(#11451,#11452,#11453,#11454,#11455,
#11456,#11457,#11458,#11459,#11460,#11461,#11462,#11463,#11464,#11465,#11466,
#11467,#11468,#11469,#11470,#11471,#11472,#11473,#11474,#11475),
 .UNSPECIFIED.,.F.,.F.,(4,3,3,3,3,3,3,3,4),(-98.096754013335,-97.8481405621833,
-96.8496901482834,-95.8512397343836,-94.8527893204838,-93.854338906584,
-92.8558884926841,-91.8574380787843,-91.8135687061554),.UNSPECIFIED.);
#1591=B_SPLINE_CURVE_WITH_KNOTS('',3,(#11480,#11481,#11482,#11483,#11484,
#11485,#11486,#11487,#11488,#11489,#11490,#11491,#11492,#11493,#11494,#11495,
#11496,#11497,#11498,#11499,#11500,#11501),.UNSPECIFIED.,.F.,.F.,(4,3,3,
3,3,3,3,4),(89.2741574414913,89.8605372509847,90.8589876648845,91.8574380787843,
92.8558884926841,93.854338906584,94.8527893204838,95.5573427486709),
 .UNSPECIFIED.);
#1592=B_SPLINE_CURVE_WITH_KNOTS('',3,(#11502,#11503,#11504,#11505,#11506,
#11507,#11508,#11509,#11510,#11511,#11512,#11513,#11514,#11515,#11516,#11517,
#11518,#11519,#11520,#11521,#11522,#11523),.UNSPECIFIED.,.F.,.F.,(4,3,3,
3,3,3,3,4),(-91.8135687061554,-90.8589876648845,-89.8605372509847,-88.8620868370848,
-87.863636423185,-86.8651860092852,-85.8667355953853,-85.5303833989758),
 .UNSPECIFIED.);
#1593=B_SPLINE_CURVE_WITH_KNOTS('',3,(#11528,#11529,#11530,#11531,#11532,
#11533,#11534,#11535,#11536,#11537,#11538,#11539,#11540,#11541,#11542,#11543,
#11544,#11545,#11546,#11547,#11548,#11549),.UNSPECIFIED.,.F.,.F.,(4,3,3,
3,3,3,3,4),(82.9909721343117,83.8698347675857,84.8682851814855,85.8667355953854,
86.8651860092852,87.863636423185,88.8620868370848,89.2741574414913),
 .UNSPECIFIED.);
#1594=B_SPLINE_CURVE_WITH_KNOTS('',3,(#11550,#11551,#11552,#11553,#11554,
#11555,#11556,#11557,#11558,#11559,#11560,#11561,#11562,#11563,#11564,#11565,
#11566,#11567,#11568,#11569,#11570,#11571),.UNSPECIFIED.,.F.,.F.,(4,3,3,
3,3,3,3,4),(-85.5303833989758,-84.8682851814855,-83.8698347675857,-82.8713843536859,
-81.872933939786,-80.8744835258862,-79.8760331119863,-79.2471980917962),
 .UNSPECIFIED.);
#1595=B_SPLINE_CURVE_WITH_KNOTS('',3,(#11576,#11577,#11578,#11579,#11580,
#11581,#11582,#11583,#11584,#11585,#11586,#11587,#11588,#11589,#11590,#11591,
#11592,#11593,#11594,#11595,#11596,#11597,#11598,#11599,#11600),
 .UNSPECIFIED.,.F.,.F.,(4,3,3,3,3,3,3,3,4),(76.7077868271321,76.8806818702869,
77.8791322841867,78.8775826980865,79.8760331119864,80.8744835258862,81.872933939786,
82.8713843536859,82.9909721343117),.UNSPECIFIED.);
#1596=B_SPLINE_CURVE_WITH_KNOTS('',3,(#11601,#11602,#11603,#11604,#11605,
#11606,#11607,#11608,#11609,#11610,#11611,#11612,#11613,#11614,#11615,#11616,
#11617,#11618,#11619,#11620,#11621,#11622),.UNSPECIFIED.,.F.,.F.,(4,3,3,
3,3,3,3,4),(-79.2471980917962,-78.8775826980865,-77.8791322841867,-76.8806818702868,
-75.882231456387,-74.8837810424872,-73.8853306285873,-72.9640127846166),
 .UNSPECIFIED.);
#1597=B_SPLINE_CURVE_WITH_KNOTS('',3,(#11627,#11628,#11629,#11630,#11631,
#11632,#11633,#11634,#11635,#11636,#11637,#11638,#11639,#11640,#11641,#11642,
#11643,#11644,#11645,#11646,#11647,#11648),.UNSPECIFIED.,.F.,.F.,(4,3,3,
3,3,3,3,4),(70.4246015199525,70.8899793868879,71.8884298007877,72.8868802146876,
73.8853306285874,74.8837810424872,75.882231456387,76.7077868271321),
 .UNSPECIFIED.);
#1598=B_SPLINE_CURVE_WITH_KNOTS('',3,(#11649,#11650,#11651,#11652,#11653,
#11654,#11655,#11656,#11657,#11658,#11659,#11660,#11661,#11662,#11663,#11664,
#11665,#11666,#11667,#11668,#11669,#11670,#11671,#11672,#11673),
 .UNSPECIFIED.,.F.,.F.,(4,3,3,3,3,3,3,3,4),(-72.9640127846166,-72.8868802146875,
-71.8884298007877,-70.8899793868879,-69.891528972988,-68.8930785590882,
-67.8946281451884,-66.8961777312885,-66.680827477437),.UNSPECIFIED.);
#1599=B_SPLINE_CURVE_WITH_KNOTS('',3,(#11678,#11679,#11680,#11681,#11682,
#11683,#11684,#11685,#11686,#11687,#11688,#11689,#11690,#11691,#11692,#11693,
#11694,#11695,#11696,#11697,#11698,#11699),.UNSPECIFIED.,.F.,.F.,(4,3,3,
3,3,3,3,4),(64.1414162127729,64.8992769034889,65.8977273173887,66.8961777312886,
67.8946281451884,68.8930785590882,69.8915289729881,70.4246015199525),
 .UNSPECIFIED.);
#1600=B_SPLINE_CURVE_WITH_KNOTS('',3,(#11700,#11701,#11702,#11703,#11704,
#11705,#11706,#11707,#11708,#11709,#11710,#11711,#11712,#11713,#11714,#11715,
#11716,#11717,#11718,#11719,#11720,#11721),.UNSPECIFIED.,.F.,.F.,(4,3,3,
3,3,3,3,4),(-66.680827477437,-65.8977273173887,-64.8992769034889,-63.9008264895891,
-62.9023760756892,-61.9039256617894,-60.9054752478896,-60.3976421702574),
 .UNSPECIFIED.);
#1601=B_SPLINE_CURVE_WITH_KNOTS('',3,(#11726,#11727,#11728,#11729,#11730,
#11731,#11732,#11733,#11734,#11735,#11736,#11737,#11738,#11739,#11740,#11741,
#11742,#11743,#11744,#11745,#11746,#11747,#11748,#11749,#11750),
 .UNSPECIFIED.,.F.,.F.,(4,3,3,3,3,3,3,3,4),(57.8582309055933,57.9101240061901,
58.9085744200899,59.9070248339898,60.9054752478896,61.9039256617894,62.9023760756893,
63.9008264895891,64.1414162127729),.UNSPECIFIED.);
#1602=B_SPLINE_CURVE_WITH_KNOTS('',3,(#11751,#11752,#11753,#11754,#11755,
#11756,#11757,#11758,#11759,#11760,#11761,#11762,#11763,#11764,#11765,#11766,
#11767,#11768,#11769,#11770,#11771,#11772),.UNSPECIFIED.,.F.,.F.,(4,3,3,
3,3,3,3,4),(-60.3976421702574,-59.9070248339898,-58.9085744200899,-57.9101240061901,
-56.9116735922903,-55.9132231783904,-54.9147727644906,-54.1144568630778),
 .UNSPECIFIED.);
#1603=B_SPLINE_CURVE_WITH_KNOTS('',3,(#11777,#11778,#11779,#11780,#11781,
#11782,#11783,#11784,#11785,#11786,#11787,#11788,#11789,#11790,#11791,#11792,
#11793,#11794,#11795,#11796,#11797,#11798),.UNSPECIFIED.,.F.,.F.,(4,3,3,
3,3,3,3,4),(51.5750455984138,51.9194215227911,52.917871936691,53.9163223505908,
54.9147727644906,55.9132231783905,56.9116735922903,57.8582309055933),
 .UNSPECIFIED.);
#1604=B_SPLINE_CURVE_WITH_KNOTS('',3,(#11799,#11800,#11801,#11802,#11803,
#11804,#11805,#11806,#11807,#11808,#11809,#11810,#11811,#11812,#11813,#11814,
#11815,#11816,#11817,#11818,#11819,#11820,#11821,#11822,#11823),
 .UNSPECIFIED.,.F.,.F.,(4,3,3,3,3,3,3,3,4),(-54.1144568630778,-53.9163223505908,
-52.917871936691,-51.9194215227911,-50.9209711088913,-49.9225206949915,
-48.9240702810916,-47.9256198671918,-47.8312715558982),.UNSPECIFIED.);
#1605=B_SPLINE_CURVE_WITH_KNOTS('',3,(#11828,#11829,#11830,#11831,#11832,
#11833,#11834,#11835,#11836,#11837,#11838,#11839,#11840,#11841,#11842,#11843,
#11844,#11845,#11846,#11847,#11848,#11849),.UNSPECIFIED.,.F.,.F.,(4,3,3,
3,3,3,3,4),(45.2918602912342,45.9287190393922,46.927169453292,47.9256198671918,
48.9240702810916,49.9225206949915,50.9209711088913,51.5750455984138),
 .UNSPECIFIED.);
#1606=B_SPLINE_CURVE_WITH_KNOTS('',3,(#11850,#11851,#11852,#11853,#11854,
#11855,#11856,#11857,#11858,#11859,#11860,#11861,#11862,#11863,#11864,#11865,
#11866,#11867,#11868,#11869,#11870,#11871),.UNSPECIFIED.,.F.,.F.,(4,3,3,
3,3,3,3,4),(-47.8312715558982,-46.927169453292,-45.9287190393921,-44.9302686254923,
-43.9318182115925,-42.9333677976927,-41.9349173837928,-41.5480862487187),
 .UNSPECIFIED.);
#1607=B_SPLINE_CURVE_WITH_KNOTS('',3,(#11876,#11877,#11878,#11879,#11880,
#11881,#11882,#11883,#11884,#11885,#11886,#11887,#11888,#11889,#11890,#11891,
#11892,#11893,#11894,#11895,#11896,#11897),.UNSPECIFIED.,.F.,.F.,(4,3,3,
3,3,3,3,4),(39.0086749840546,39.9380165559932,40.936466969893,41.9349173837928,
42.9333677976927,43.9318182115925,44.9302686254923,45.2918602912342),
 .UNSPECIFIED.);
#1608=B_SPLINE_CURVE_WITH_KNOTS('',3,(#11898,#11899,#11900,#11901,#11902,
#11903,#11904,#11905,#11906,#11907,#11908,#11909,#11910,#11911,#11912,#11913,
#11914,#11915,#11916,#11917,#11918,#11919),.UNSPECIFIED.,.F.,.F.,(4,3,3,
3,3,3,3,4),(-41.5480862487187,-40.936466969893,-39.9380165559932,-38.9395661420933,
-37.9411157281935,-36.9426653142937,-35.9442149003939,-35.2649009415391),
 .UNSPECIFIED.);
#1609=B_SPLINE_CURVE_WITH_KNOTS('',3,(#11924,#11925,#11926,#11927,#11928,
#11929,#11930,#11931,#11932,#11933,#11934,#11935,#11936,#11937,#11938,#11939,
#11940,#11941,#11942,#11943,#11944,#11945,#11946,#11947,#11948),
 .UNSPECIFIED.,.F.,.F.,(4,3,3,3,3,3,3,3,4),(32.725489676875,32.9488636586944,
33.9473140725942,34.945764486494,35.9442149003939,36.9426653142937,37.9411157281935,
38.9395661420933,39.0086749840546),.UNSPECIFIED.);
#1610=B_SPLINE_CURVE_WITH_KNOTS('',3,(#11949,#11950,#11951,#11952,#11953,
#11954,#11955,#11956,#11957,#11958,#11959,#11960,#11961,#11962,#11963,#11964,
#11965,#11966,#11967,#11968,#11969,#11970),.UNSPECIFIED.,.F.,.F.,(4,3,3,
3,3,3,3,4),(-35.2649009415391,-34.945764486494,-33.9473140725942,-32.9488636586944,
-31.9504132447945,-30.9519628308947,-29.9535124169949,-28.9817156343595),
 .UNSPECIFIED.);
#1611=B_SPLINE_CURVE_WITH_KNOTS('',3,(#11975,#11976,#11977,#11978,#11979,
#11980,#11981,#11982,#11983,#11984,#11985,#11986,#11987,#11988,#11989,#11990,
#11991,#11992,#11993,#11994,#11995,#11996),.UNSPECIFIED.,.F.,.F.,(4,3,3,
3,3,3,3,4),(26.4423043696954,26.9581611752954,27.9566115891952,28.955062003095,
29.9535124169949,30.9519628308947,31.9504132447945,32.725489676875),
 .UNSPECIFIED.);
#1612=B_SPLINE_CURVE_WITH_KNOTS('',3,(#11997,#11998,#11999,#12000,#12001,
#12002,#12003,#12004,#12005,#12006,#12007,#12008,#12009,#12010,#12011,#12012,
#12013,#12014,#12015,#12016,#12017,#12018,#12019,#12020,#12021),
 .UNSPECIFIED.,.F.,.F.,(4,3,3,3,3,3,3,3,4),(-28.9817156343595,-28.955062003095,
-27.9566115891952,-26.9581611752954,-25.9597107613956,-24.9612603474957,
-23.9628099335959,-22.9643595196961,-22.6985303271799),.UNSPECIFIED.);
#1613=B_SPLINE_CURVE_WITH_KNOTS('',3,(#12026,#12027,#12028,#12029,#12030,
#12031,#12032,#12033,#12034,#12035,#12036,#12037,#12038,#12039,#12040,#12041,
#12042,#12043,#12044,#12045,#12046,#12047),.UNSPECIFIED.,.F.,.F.,(4,3,3,
3,3,3,3,4),(20.1591190625158,20.9674586918964,21.9659091057962,22.9643595196961,
23.9628099335959,24.9612603474957,25.9597107613956,26.4423043696954),
 .UNSPECIFIED.);
#1614=B_SPLINE_CURVE_WITH_KNOTS('',3,(#12048,#12049,#12050,#12051,#12052,
#12053,#12054,#12055,#12056,#12057,#12058,#12059,#12060,#12061,#12062,#12063,
#12064,#12065,#12066,#12067,#12068,#12069),.UNSPECIFIED.,.F.,.F.,(4,3,3,
3,3,3,3,4),(-22.6985303271799,-21.9659091057962,-20.9674586918964,-19.9690082779966,
-18.9705578640968,-17.9721074501969,-16.9736570362971,-16.4153450200003),
 .UNSPECIFIED.);
#1615=B_SPLINE_CURVE_WITH_KNOTS('',3,(#12074,#12075,#12076,#12077,#12078,
#12079,#12080,#12081,#12082,#12083,#12084,#12085,#12086,#12087,#12088,#12089,
#12090,#12091,#12092,#12093,#12094,#12095,#12096,#12097,#12098),
 .UNSPECIFIED.,.F.,.F.,(4,3,3,3,3,3,3,3,4),(13.8759337553362,13.9783057945976,
14.9767562084974,15.9752066223973,16.9736570362971,17.9721074501969,18.9705578640968,
19.9690082779966,20.1591190625158),.UNSPECIFIED.);
#1616=B_SPLINE_CURVE_WITH_KNOTS('',3,(#12099,#12100,#12101,#12102,#12103,
#12104,#12105,#12106,#12107,#12108,#12109,#12110,#12111,#12112,#12113,#12114,
#12115,#12116,#12117,#12118,#12119,#12120),.UNSPECIFIED.,.F.,.F.,(4,3,3,
3,3,3,3,4),(-16.4153450200003,-15.9752066223973,-14.9767562084974,-13.9783057945976,
-12.9798553806978,-11.9814049667979,-10.9829545528981,-10.1321597128207),
 .UNSPECIFIED.);
#1617=B_SPLINE_CURVE_WITH_KNOTS('',3,(#12126,#12127,#12128,#12129,#12130,
#12131,#12132,#12133,#12134,#12135,#12136,#12137,#12138),.UNSPECIFIED.,
 .F.,.F.,(4,3,3,3,4),(-3.84897440564113,-2.99535124169948,-1.99690082779965,
-0.998450413899827,0.),.UNSPECIFIED.);
#1618=B_SPLINE_CURVE_WITH_KNOTS('',3,(#12141,#12142,#12143,#12144,#12145,
#12146,#12147,#12148,#12149,#12150,#12151,#12152,#12153,#12154,#12155,#12156,
#12157,#12158,#12159),.UNSPECIFIED.,.F.,.F.,(4,3,3,3,3,3,4),(2.01694489302838,
2.99535124169949,3.99380165559932,4.99225206949915,5.99070248339898,6.98915289729881,
7.59274844815663),.UNSPECIFIED.);
#1619=B_SPLINE_CURVE_WITH_KNOTS('',3,(#12165,#12166,#12167,#12168,#12169,
#12170,#12171,#12172),.UNSPECIFIED.,.F.,.F.,(4,1,1,1,1,4),(116.238928182822,
116.69628232179,117.69473273569,118.693183149589,119.691633563489,120.690083977389),
 .UNSPECIFIED.);
#1620=B_SPLINE_CURVE_WITH_KNOTS('',3,(#12175,#12176,#12177,#12178,#12179,
#12180,#12181,#12182,#12183),.UNSPECIFIED.,.F.,.F.,(4,1,1,1,1,1,4),(116.238928182822,
116.240342344754,117.238792758654,118.237243172554,119.235693586454,120.234144000354,
121.212550349025),.UNSPECIFIED.);
#1621=B_SPLINE_CURVE_WITH_KNOTS('',3,(#12188,#12189,#12190,#12191,#12192,
#12193,#12194,#12195,#12196,#12197),.UNSPECIFIED.,.F.,.F.,(4,1,1,1,1,1,
1,4),(109.955742875643,110.705579838391,111.704030252291,112.70248066619,
113.70093108009,114.69938149399,115.69783190789,116.238928182822),
 .UNSPECIFIED.);
#1622=B_SPLINE_CURVE_WITH_KNOTS('',3,(#12198,#12199,#12200,#12201,#12202,
#12203,#12204,#12205,#12206,#12207),.UNSPECIFIED.,.F.,.F.,(4,1,1,1,1,1,
1,4),(109.955742875643,110.249639861355,111.248090275255,112.246540689155,
113.244991103055,114.243441516955,115.241891930855,116.238928182822),
 .UNSPECIFIED.);
#1623=B_SPLINE_CURVE_WITH_KNOTS('',3,(#12212,#12213,#12214,#12215,#12216,
#12217,#12218,#12219,#12220,#12221,#12222),.UNSPECIFIED.,.F.,.F.,(4,1,1,
1,1,1,1,1,4),(103.672557568463,103.716426941092,104.714877354992,105.713327768892,
106.711778182792,107.710228596691,108.708679010591,109.707129424491,109.955742875643),
 .UNSPECIFIED.);
#1624=B_SPLINE_CURVE_WITH_KNOTS('',3,(#12223,#12224,#12225,#12226,#12227,
#12228,#12229,#12230,#12231,#12232),.UNSPECIFIED.,.F.,.F.,(4,1,1,1,1,1,
1,4),(103.672557568463,104.258937377956,105.257387791856,106.255838205756,
107.254288619656,108.252739033556,109.251189447456,109.955742875643),
 .UNSPECIFIED.);
#1625=B_SPLINE_CURVE_WITH_KNOTS('',3,(#12237,#12238,#12239,#12240,#12241,
#12242,#12243,#12244,#12245,#12246),.UNSPECIFIED.,.F.,.F.,(4,1,1,1,1,1,
1,4),(97.3893722612835,97.725724457693,98.7241748715929,99.7226252854927,
100.721075699393,101.719526113292,102.717976527192,103.672557568463),
 .UNSPECIFIED.);
#1626=B_SPLINE_CURVE_WITH_KNOTS('',3,(#12247,#12248,#12249,#12250,#12251,
#12252,#12253,#12254,#12255,#12256),.UNSPECIFIED.,.F.,.F.,(4,1,1,1,1,1,
1,4),(97.3893722612835,98.2682348945574,99.2666853084573,100.265135722357,
101.263586136257,102.262036550157,103.260486964057,103.672557568463),
 .UNSPECIFIED.);
#1627=B_SPLINE_CURVE_WITH_KNOTS('',3,(#12261,#12262,#12263,#12264,#12265,
#12266,#12267,#12268,#12269,#12270),.UNSPECIFIED.,.F.,.F.,(4,1,1,1,1,1,
1,4),(91.106186954104,91.7350219742941,92.7334723881939,93.7319228020937,
94.7303732159936,95.7288236298934,96.7272740437932,97.3893722612835),
 .UNSPECIFIED.);
#1628=B_SPLINE_CURVE_WITH_KNOTS('',3,(#12271,#12272,#12273,#12274,#12275,
#12276,#12277,#12278,#12279,#12280,#12281),.UNSPECIFIED.,.F.,.F.,(4,1,1,
1,1,1,1,1,4),(91.106186954104,91.2790819972586,92.2775324111584,93.2759828250583,
94.2744332389581,95.2728836528579,96.2713340667578,97.2697844806576,97.3893722612835),
 .UNSPECIFIED.);
#1629=B_SPLINE_CURVE_WITH_KNOTS('',3,(#12286,#12287,#12288,#12289,#12290,
#12291,#12292,#12293,#12294,#12295),.UNSPECIFIED.,.F.,.F.,(4,1,1,1,1,1,
1,4),(84.8230016469244,85.7443194908951,86.7427699047949,87.7412203186948,
88.7396707325946,89.7381211464944,90.7365715603942,91.106186954104),
 .UNSPECIFIED.);
#1630=B_SPLINE_CURVE_WITH_KNOTS('',3,(#12296,#12297,#12298,#12299,#12300,
#12301,#12302,#12303,#12304,#12305),.UNSPECIFIED.,.F.,.F.,(4,1,1,1,1,1,
1,4),(84.8230016469244,85.2883795138596,86.2868299277595,87.2852803416593,
88.2837307555591,89.282181169459,90.2806315833588,91.106186954104),
 .UNSPECIFIED.);
#1631=B_SPLINE_CURVE_WITH_KNOTS('',3,(#12310,#12311,#12312,#12313,#12314,
#12315,#12316,#12317,#12318,#12319,#12320),.UNSPECIFIED.,.F.,.F.,(4,1,1,
1,1,1,1,1,4),(78.5398163397448,78.7551665935963,79.7536170074961,80.7520674213959,
81.7505178352958,82.7489682491956,83.7474186630954,84.7458690769953,84.8230016469244),
 .UNSPECIFIED.);
#1632=B_SPLINE_CURVE_WITH_KNOTS('',3,(#12321,#12322,#12323,#12324,#12325,
#12326,#12327,#12328,#12329,#12330),.UNSPECIFIED.,.F.,.F.,(4,1,1,1,1,1,
1,4),(78.5398163397448,79.2976770304607,80.2961274443605,81.2945778582603,
82.2930282721602,83.29147868606,84.2899290999598,84.8230016469244),
 .UNSPECIFIED.);
#1633=B_SPLINE_CURVE_WITH_KNOTS('',3,(#12335,#12336,#12337,#12338,#12339,
#12340,#12341,#12342,#12343,#12344),.UNSPECIFIED.,.F.,.F.,(4,1,1,1,1,1,
1,4),(72.2566310325652,72.7644641101973,73.7629145240972,74.761364937997,
75.7598153518968,76.7582657657966,77.7567161796965,78.5398163397448),
 .UNSPECIFIED.);
#1634=B_SPLINE_CURVE_WITH_KNOTS('',3,(#12345,#12346,#12347,#12348,#12349,
#12350,#12351,#12352,#12353,#12354,#12355),.UNSPECIFIED.,.F.,.F.,(4,1,1,
1,1,1,1,1,4),(72.2566310325652,72.3085241331619,73.3069745470617,74.3054249609615,
75.3038753748613,76.3023257887612,77.300776202661,78.2992266165608,78.5398163397448),
 .UNSPECIFIED.);
#1635=B_SPLINE_CURVE_WITH_KNOTS('',3,(#12360,#12361,#12362,#12363,#12364,
#12365,#12366,#12367,#12368,#12369),.UNSPECIFIED.,.F.,.F.,(4,1,1,1,1,1,
1,4),(65.9734457253856,66.7737616267983,67.7722120406982,68.770662454598,
69.7691128684978,70.7675632823977,71.7660136962975,72.2566310325652),
 .UNSPECIFIED.);
#1636=B_SPLINE_CURVE_WITH_KNOTS('',3,(#12370,#12371,#12372,#12373,#12374,
#12375,#12376,#12377,#12378,#12379),.UNSPECIFIED.,.F.,.F.,(4,1,1,1,1,1,
1,4),(65.9734457253856,66.3178216497629,67.3162720636627,68.3147224775625,
69.3131728914624,70.3116233053622,71.310073719262,72.2566310325652),
 .UNSPECIFIED.);
#1637=B_SPLINE_CURVE_WITH_KNOTS('',3,(#12384,#12385,#12386,#12387,#12388,
#12389,#12390,#12391,#12392,#12393,#12394),.UNSPECIFIED.,.F.,.F.,(4,1,1,
1,1,1,1,1,4),(59.690260418206,59.7846087294995,60.7830591433994,61.7815095572992,
62.779959971199,63.7784103850989,64.7768607989987,65.7753112128985,65.9734457253856),
 .UNSPECIFIED.);
#1638=B_SPLINE_CURVE_WITH_KNOTS('',3,(#12395,#12396,#12397,#12398,#12399,
#12400,#12401,#12402,#12403,#12404),.UNSPECIFIED.,.F.,.F.,(4,1,1,1,1,1,
1,4),(59.690260418206,60.3271191663639,61.3255695802637,62.3240199941636,
63.3224704080634,64.3209208219632,65.3193712358631,65.9734457253856),
 .UNSPECIFIED.);
#1639=B_SPLINE_CURVE_WITH_KNOTS('',3,(#12409,#12410,#12411,#12412,#12413,
#12414,#12415,#12416,#12417,#12418),.UNSPECIFIED.,.F.,.F.,(4,1,1,1,1,1,
1,4),(53.4070751110264,53.7939062461006,54.7923566600004,55.7908070739002,
56.7892574878001,57.7877079016999,58.7861583155997,59.690260418206),
 .UNSPECIFIED.);
#1640=B_SPLINE_CURVE_WITH_KNOTS('',3,(#12419,#12420,#12421,#12422,#12423,
#12424,#12425,#12426,#12427,#12428),.UNSPECIFIED.,.F.,.F.,(4,1,1,1,1,1,
1,4),(53.4070751110264,54.3364166829649,55.3348670968648,56.3333175107646,
57.3317679246644,58.3302183385643,59.3286687524641,59.690260418206),
 .UNSPECIFIED.);
#1641=B_SPLINE_CURVE_WITH_KNOTS('',3,(#12433,#12434,#12435,#12436,#12437,
#12438,#12439,#12440,#12441,#12442),.UNSPECIFIED.,.F.,.F.,(4,1,1,1,1,1,
1,4),(47.1238898038468,47.8032037627016,48.8016541766014,49.8001045905012,
50.7985550044011,51.7970054183009,52.7954558322007,53.4070751110264),
 .UNSPECIFIED.);
#1642=B_SPLINE_CURVE_WITH_KNOTS('',3,(#12443,#12444,#12445,#12446,#12447,
#12448,#12449,#12450,#12451,#12452,#12453),.UNSPECIFIED.,.F.,.F.,(4,1,1,
1,1,1,1,1,4),(47.1238898038468,47.3472637856661,48.345714199566,49.3441646134658,
50.3426150273656,51.3410654412654,52.3395158551653,53.3379662690651,53.4070751110264),
 .UNSPECIFIED.);
#1643=B_SPLINE_CURVE_WITH_KNOTS('',3,(#12458,#12459,#12460,#12461,#12462,
#12463,#12464,#12465,#12466,#12467),.UNSPECIFIED.,.F.,.F.,(4,1,1,1,1,1,
1,4),(40.8407044966672,41.8125012793026,42.8109516932024,43.8094021071023,
44.8078525210021,45.8063029349019,46.8047533488018,47.1238898038468),
 .UNSPECIFIED.);
#1644=B_SPLINE_CURVE_WITH_KNOTS('',3,(#12468,#12469,#12470,#12471,#12472,
#12473,#12474,#12475,#12476,#12477),.UNSPECIFIED.,.F.,.F.,(4,1,1,1,1,1,
1,4),(40.8407044966672,41.3565613022671,42.355011716167,43.3534621300668,
44.3519125439666,45.3503629578665,46.3488133717663,47.1238898038468),
 .UNSPECIFIED.);
#1645=B_SPLINE_CURVE_WITH_KNOTS('',3,(#12482,#12483,#12484,#12485,#12486,
#12487,#12488,#12489,#12490,#12491,#12492),.UNSPECIFIED.,.F.,.F.,(4,1,1,
1,1,1,1,1,4),(34.5575191894876,34.8233483820038,35.8217987959036,36.8202492098035,
37.8186996237033,38.8171500376031,39.815600451503,40.8140508654028,40.8407044966672),
 .UNSPECIFIED.);
#1646=B_SPLINE_CURVE_WITH_KNOTS('',3,(#12493,#12494,#12495,#12496,#12497,
#12498,#12499,#12500,#12501,#12502),.UNSPECIFIED.,.F.,.F.,(4,1,1,1,1,1,
1,4),(34.5575191894876,35.3658588188682,36.364309232768,37.3627596466678,
38.3612100605677,39.3596604744675,40.3581108883673,40.8407044966672),
 .UNSPECIFIED.);
#1647=B_SPLINE_CURVE_WITH_KNOTS('',3,(#12507,#12508,#12509,#12510,#12511,
#12512,#12513,#12514,#12515,#12516),.UNSPECIFIED.,.F.,.F.,(4,1,1,1,1,1,
1,4),(28.274333882308,28.8326458986048,29.8310963125047,30.8295467264045,
31.8279971403043,32.8264475542042,33.824897968104,34.5575191894876),
 .UNSPECIFIED.);
#1648=B_SPLINE_CURVE_WITH_KNOTS('',3,(#12517,#12518,#12519,#12520,#12521,
#12522,#12523,#12524,#12525,#12526,#12527),.UNSPECIFIED.,.F.,.F.,(4,1,1,
1,1,1,1,1,4),(28.274333882308,28.3767059215694,29.3751563354692,30.373606749369,
31.3720571632689,32.3705075771687,33.3689579910685,34.3674084049683,34.5575191894876),
 .UNSPECIFIED.);
#1649=B_SPLINE_CURVE_WITH_KNOTS('',3,(#12532,#12533,#12534,#12535,#12536,
#12537,#12538,#12539,#12540,#12541),.UNSPECIFIED.,.F.,.F.,(4,1,1,1,1,1,
1,4),(21.9911485751285,22.8419434152059,23.8403938291057,24.8388442430055,
25.8372946569053,26.8357450708052,27.834195484705,28.274333882308),
 .UNSPECIFIED.);
#1650=B_SPLINE_CURVE_WITH_KNOTS('',3,(#12542,#12543,#12544,#12545,#12546,
#12547,#12548,#12549,#12550,#12551),.UNSPECIFIED.,.F.,.F.,(4,1,1,1,1,1,
1,4),(21.9911485751285,22.3860034381704,23.3844538520702,24.38290426597,
25.3813546798699,26.3798050937697,27.3782555076695,28.274333882308),
 .UNSPECIFIED.);
#1651=B_SPLINE_CURVE_WITH_KNOTS('',3,(#12557,#12558,#12559,#12560,#12561),
 .UNSPECIFIED.,.F.,.F.,(4,1,4),(14.3984001269718,15.3968505408716,15.7079632679489),
 .UNSPECIFIED.);
#1652=B_SPLINE_CURVE_WITH_KNOTS('',3,(#12564,#12565,#12566,#12567,#12568),
 .UNSPECIFIED.,.F.,.F.,(4,1,4),(13.8759337553362,14.8543401040072,15.7079632679489),
 .UNSPECIFIED.);
#1653=B_SPLINE_CURVE_WITH_KNOTS('',3,(#12574,#12575,#12576,#12577),
 .UNSPECIFIED.,.F.,.F.,(4,4),(108.12371336303,108.831095115081),
 .UNSPECIFIED.);
#1654=B_SPLINE_CURVE_WITH_KNOTS('',3,(#12585,#12586,#12587,#12588,#12589,
#12590,#12591,#12592,#12593,#12594),.UNSPECIFIED.,.F.,.F.,(4,3,3,4),(-106.814150222053,
-105.835743873382,-104.837293459482,-104.379939320515),.UNSPECIFIED.);
#1655=B_SPLINE_CURVE_WITH_KNOTS('',3,(#12599,#12600,#12601,#12602,#12603,
#12604,#12605,#12606,#12607,#12608,#12609,#12610,#12611,#12612,#12613,#12614,
#12615,#12616,#12617,#12618,#12619,#12620),.UNSPECIFIED.,.F.,.F.,(4,3,3,
3,3,3,3,4),(101.84052805585,102.840392631682,103.838843045582,104.837293459482,
105.835743873382,106.834194287282,107.832644701182,108.12371336303),
 .UNSPECIFIED.);
#1656=B_SPLINE_CURVE_WITH_KNOTS('',3,(#12621,#12622,#12623,#12624,#12625,
#12626,#12627,#12628,#12629,#12630,#12631,#12632,#12633,#12634,#12635,#12636,
#12637,#12638,#12639,#12640,#12641,#12642),.UNSPECIFIED.,.F.,.F.,(4,3,3,
3,3,3,3,4),(-104.379939320515,-103.838843045582,-102.840392631682,-101.841942217783,
-100.843491803883,-99.8450413899829,-98.8465909760831,-98.096754013335),
 .UNSPECIFIED.);
#1657=B_SPLINE_CURVE_WITH_KNOTS('',3,(#12647,#12648,#12649,#12650,#12651,
#12652,#12653,#12654,#12655,#12656,#12657,#12658,#12659,#12660,#12661,#12662,
#12663,#12664,#12665,#12666,#12667,#12668),.UNSPECIFIED.,.F.,.F.,(4,3,3,
3,3,3,3,4),(95.5573427486709,95.8512397343836,96.8496901482835,97.8481405621833,
98.8465909760831,99.845041389983,100.843491803883,101.84052805585),
 .UNSPECIFIED.);
#1658=B_SPLINE_CURVE_WITH_KNOTS('',3,(#12669,#12670,#12671,#12672,#12673,
#12674,#12675,#12676,#12677,#12678,#12679,#12680,#12681,#12682,#12683,#12684,
#12685,#12686,#12687,#12688,#12689,#12690,#12691,#12692,#12693),
 .UNSPECIFIED.,.F.,.F.,(4,3,3,3,3,3,3,3,4),(-98.096754013335,-97.8481405621833,
-96.8496901482835,-95.8512397343836,-94.8527893204838,-93.854338906584,
-92.8558884926841,-91.8574380787843,-91.8135687061554),.UNSPECIFIED.);
#1659=B_SPLINE_CURVE_WITH_KNOTS('',3,(#12698,#12699,#12700,#12701,#12702,
#12703,#12704,#12705,#12706,#12707,#12708,#12709,#12710,#12711,#12712,#12713,
#12714,#12715,#12716,#12717,#12718,#12719),.UNSPECIFIED.,.F.,.F.,(4,3,3,
3,3,3,3,4),(89.2741574414913,89.8605372509847,90.8589876648845,91.8574380787843,
92.8558884926841,93.854338906584,94.8527893204838,95.5573427486709),
 .UNSPECIFIED.);
#1660=B_SPLINE_CURVE_WITH_KNOTS('',3,(#12720,#12721,#12722,#12723,#12724,
#12725,#12726,#12727,#12728,#12729,#12730,#12731,#12732,#12733,#12734,#12735,
#12736,#12737,#12738,#12739,#12740,#12741),.UNSPECIFIED.,.F.,.F.,(4,3,3,
3,3,3,3,4),(-91.8135687061554,-90.8589876648845,-89.8605372509847,-88.8620868370848,
-87.863636423185,-86.8651860092852,-85.8667355953854,-85.5303833989758),
 .UNSPECIFIED.);
#1661=B_SPLINE_CURVE_WITH_KNOTS('',3,(#12746,#12747,#12748,#12749,#12750,
#12751,#12752,#12753,#12754,#12755,#12756,#12757,#12758,#12759,#12760,#12761,
#12762,#12763,#12764,#12765,#12766,#12767),.UNSPECIFIED.,.F.,.F.,(4,3,3,
3,3,3,3,4),(82.9909721343117,83.8698347675857,84.8682851814855,85.8667355953853,
86.8651860092852,87.863636423185,88.8620868370848,89.2741574414913),
 .UNSPECIFIED.);
#1662=B_SPLINE_CURVE_WITH_KNOTS('',3,(#12768,#12769,#12770,#12771,#12772,
#12773,#12774,#12775,#12776,#12777,#12778,#12779,#12780,#12781,#12782,#12783,
#12784,#12785,#12786,#12787,#12788,#12789),.UNSPECIFIED.,.F.,.F.,(4,3,3,
3,3,3,3,4),(-85.5303833989758,-84.8682851814855,-83.8698347675857,-82.8713843536858,
-81.872933939786,-80.8744835258862,-79.8760331119864,-79.2471980917962),
 .UNSPECIFIED.);
#1663=B_SPLINE_CURVE_WITH_KNOTS('',3,(#12794,#12795,#12796,#12797,#12798,
#12799,#12800,#12801,#12802,#12803,#12804,#12805,#12806,#12807,#12808,#12809,
#12810,#12811,#12812,#12813,#12814,#12815,#12816,#12817,#12818),
 .UNSPECIFIED.,.F.,.F.,(4,3,3,3,3,3,3,3,4),(76.7077868271321,76.8806818702869,
77.8791322841867,78.8775826980865,79.8760331119864,80.8744835258862,81.872933939786,
82.8713843536859,82.9909721343117),.UNSPECIFIED.);
#1664=B_SPLINE_CURVE_WITH_KNOTS('',3,(#12819,#12820,#12821,#12822,#12823,
#12824,#12825,#12826,#12827,#12828,#12829,#12830,#12831,#12832,#12833,#12834,
#12835,#12836,#12837,#12838,#12839,#12840),.UNSPECIFIED.,.F.,.F.,(4,3,3,
3,3,3,3,4),(-79.2471980917962,-78.8775826980865,-77.8791322841867,-76.8806818702869,
-75.882231456387,-74.8837810424872,-73.8853306285874,-72.9640127846166),
 .UNSPECIFIED.);
#1665=B_SPLINE_CURVE_WITH_KNOTS('',3,(#12845,#12846,#12847,#12848,#12849,
#12850,#12851,#12852,#12853,#12854,#12855,#12856,#12857,#12858,#12859,#12860,
#12861,#12862,#12863,#12864,#12865,#12866),.UNSPECIFIED.,.F.,.F.,(4,3,3,
3,3,3,3,4),(70.4246015199525,70.8899793868879,71.8884298007877,72.8868802146876,
73.8853306285874,74.8837810424872,75.882231456387,76.7077868271321),
 .UNSPECIFIED.);
#1666=B_SPLINE_CURVE_WITH_KNOTS('',3,(#12867,#12868,#12869,#12870,#12871,
#12872,#12873,#12874,#12875,#12876,#12877,#12878,#12879,#12880,#12881,#12882,
#12883,#12884,#12885,#12886,#12887,#12888,#12889,#12890,#12891),
 .UNSPECIFIED.,.F.,.F.,(4,3,3,3,3,3,3,3,4),(-72.9640127846166,-72.8868802146875,
-71.8884298007877,-70.8899793868879,-69.8915289729881,-68.8930785590882,
-67.8946281451884,-66.8961777312886,-66.680827477437),.UNSPECIFIED.);
#1667=B_SPLINE_CURVE_WITH_KNOTS('',3,(#12896,#12897,#12898,#12899,#12900,
#12901,#12902,#12903,#12904,#12905,#12906,#12907,#12908,#12909,#12910,#12911,
#12912,#12913,#12914,#12915,#12916,#12917),.UNSPECIFIED.,.F.,.F.,(4,3,3,
3,3,3,3,4),(64.1414162127729,64.8992769034889,65.8977273173887,66.8961777312886,
67.8946281451884,68.8930785590882,69.8915289729881,70.4246015199525),
 .UNSPECIFIED.);
#1668=B_SPLINE_CURVE_WITH_KNOTS('',3,(#12918,#12919,#12920,#12921,#12922,
#12923,#12924,#12925,#12926,#12927,#12928,#12929,#12930,#12931,#12932,#12933,
#12934,#12935,#12936,#12937,#12938,#12939),.UNSPECIFIED.,.F.,.F.,(4,3,3,
3,3,3,3,4),(-66.680827477437,-65.8977273173887,-64.8992769034889,-63.9008264895891,
-62.9023760756892,-61.9039256617894,-60.9054752478896,-60.3976421702574),
 .UNSPECIFIED.);
#1669=B_SPLINE_CURVE_WITH_KNOTS('',3,(#12944,#12945,#12946,#12947,#12948,
#12949,#12950,#12951,#12952,#12953,#12954,#12955,#12956,#12957,#12958,#12959,
#12960,#12961,#12962,#12963,#12964,#12965,#12966,#12967,#12968),
 .UNSPECIFIED.,.F.,.F.,(4,3,3,3,3,3,3,3,4),(57.8582309055933,57.9101240061901,
58.9085744200899,59.9070248339898,60.9054752478896,61.9039256617894,62.9023760756893,
63.9008264895891,64.1414162127729),.UNSPECIFIED.);
#1670=B_SPLINE_CURVE_WITH_KNOTS('',3,(#12969,#12970,#12971,#12972,#12973,
#12974,#12975,#12976,#12977,#12978,#12979,#12980,#12981,#12982,#12983,#12984,
#12985,#12986,#12987,#12988,#12989,#12990),.UNSPECIFIED.,.F.,.F.,(4,3,3,
3,3,3,3,4),(-60.3976421702574,-59.9070248339898,-58.9085744200899,-57.9101240061901,
-56.9116735922903,-55.9132231783904,-54.9147727644906,-54.1144568630778),
 .UNSPECIFIED.);
#1671=B_SPLINE_CURVE_WITH_KNOTS('',3,(#12995,#12996,#12997,#12998,#12999,
#13000,#13001,#13002,#13003,#13004,#13005,#13006,#13007,#13008,#13009,#13010,
#13011,#13012,#13013,#13014,#13015,#13016),.UNSPECIFIED.,.F.,.F.,(4,3,3,
3,3,3,3,4),(51.5750455984138,51.9194215227911,52.917871936691,53.9163223505908,
54.9147727644906,55.9132231783905,56.9116735922903,57.8582309055933),
 .UNSPECIFIED.);
#1672=B_SPLINE_CURVE_WITH_KNOTS('',3,(#13017,#13018,#13019,#13020,#13021,
#13022,#13023,#13024,#13025,#13026,#13027,#13028,#13029,#13030,#13031,#13032,
#13033,#13034,#13035,#13036,#13037,#13038,#13039,#13040,#13041),
 .UNSPECIFIED.,.F.,.F.,(4,3,3,3,3,3,3,3,4),(-54.1144568630778,-53.9163223505908,
-52.917871936691,-51.9194215227911,-50.9209711088913,-49.9225206949915,
-48.9240702810916,-47.9256198671918,-47.8312715558982),.UNSPECIFIED.);
#1673=B_SPLINE_CURVE_WITH_KNOTS('',3,(#13046,#13047,#13048,#13049,#13050,
#13051,#13052,#13053,#13054,#13055,#13056,#13057,#13058,#13059,#13060,#13061,
#13062,#13063,#13064,#13065,#13066,#13067),.UNSPECIFIED.,.F.,.F.,(4,3,3,
3,3,3,3,4),(45.2918602912342,45.9287190393922,46.927169453292,47.9256198671918,
48.9240702810917,49.9225206949915,50.9209711088913,51.5750455984138),
 .UNSPECIFIED.);
#1674=B_SPLINE_CURVE_WITH_KNOTS('',3,(#13068,#13069,#13070,#13071,#13072,
#13073,#13074,#13075,#13076,#13077,#13078,#13079,#13080,#13081,#13082,#13083,
#13084,#13085,#13086,#13087,#13088,#13089),.UNSPECIFIED.,.F.,.F.,(4,3,3,
3,3,3,3,4),(-47.8312715558982,-46.927169453292,-45.9287190393921,-44.9302686254923,
-43.9318182115925,-42.9333677976927,-41.9349173837928,-41.5480862487186),
 .UNSPECIFIED.);
#1675=B_SPLINE_CURVE_WITH_KNOTS('',3,(#13094,#13095,#13096,#13097,#13098,
#13099,#13100,#13101,#13102,#13103,#13104,#13105,#13106,#13107,#13108,#13109,
#13110,#13111,#13112,#13113,#13114,#13115),.UNSPECIFIED.,.F.,.F.,(4,3,3,
3,3,3,3,4),(39.0086749840546,39.9380165559932,40.936466969893,41.9349173837928,
42.9333677976927,43.9318182115925,44.9302686254923,45.2918602912342),
 .UNSPECIFIED.);
#1676=B_SPLINE_CURVE_WITH_KNOTS('',3,(#13116,#13117,#13118,#13119,#13120,
#13121,#13122,#13123,#13124,#13125,#13126,#13127,#13128,#13129,#13130,#13131,
#13132,#13133,#13134,#13135,#13136,#13137),.UNSPECIFIED.,.F.,.F.,(4,3,3,
3,3,3,3,4),(-41.5480862487186,-40.936466969893,-39.9380165559932,-38.9395661420933,
-37.9411157281935,-36.9426653142937,-35.9442149003939,-35.2649009415391),
 .UNSPECIFIED.);
#1677=B_SPLINE_CURVE_WITH_KNOTS('',3,(#13142,#13143,#13144,#13145,#13146,
#13147,#13148,#13149,#13150,#13151,#13152,#13153,#13154,#13155,#13156,#13157,
#13158,#13159,#13160,#13161,#13162,#13163,#13164,#13165,#13166),
 .UNSPECIFIED.,.F.,.F.,(4,3,3,3,3,3,3,3,4),(32.725489676875,32.9488636586944,
33.9473140725942,34.945764486494,35.9442149003939,36.9426653142937,37.9411157281935,
38.9395661420934,39.0086749840546),.UNSPECIFIED.);
#1678=B_SPLINE_CURVE_WITH_KNOTS('',3,(#13167,#13168,#13169,#13170,#13171,
#13172,#13173,#13174,#13175,#13176,#13177,#13178,#13179,#13180,#13181,#13182,
#13183,#13184,#13185,#13186,#13187,#13188),.UNSPECIFIED.,.F.,.F.,(4,3,3,
3,3,3,3,4),(-35.2649009415391,-34.945764486494,-33.9473140725942,-32.9488636586944,
-31.9504132447945,-30.9519628308947,-29.9535124169949,-28.9817156343595),
 .UNSPECIFIED.);
#1679=B_SPLINE_CURVE_WITH_KNOTS('',3,(#13193,#13194,#13195,#13196,#13197,
#13198,#13199,#13200,#13201,#13202,#13203,#13204,#13205,#13206,#13207,#13208,
#13209,#13210,#13211,#13212,#13213,#13214),.UNSPECIFIED.,.F.,.F.,(4,3,3,
3,3,3,3,4),(26.4423043696954,26.9581611752954,27.9566115891952,28.9550620030951,
29.9535124169949,30.9519628308947,31.9504132447945,32.725489676875),
 .UNSPECIFIED.);
#1680=B_SPLINE_CURVE_WITH_KNOTS('',3,(#13215,#13216,#13217,#13218,#13219,
#13220,#13221,#13222,#13223,#13224,#13225,#13226,#13227,#13228,#13229,#13230,
#13231,#13232,#13233,#13234,#13235,#13236,#13237,#13238,#13239),
 .UNSPECIFIED.,.F.,.F.,(4,3,3,3,3,3,3,3,4),(-28.9817156343595,-28.955062003095,
-27.9566115891952,-26.9581611752954,-25.9597107613956,-24.9612603474957,
-23.9628099335959,-22.9643595196961,-22.6985303271799),.UNSPECIFIED.);
#1681=B_SPLINE_CURVE_WITH_KNOTS('',3,(#13244,#13245,#13246,#13247,#13248,
#13249,#13250,#13251,#13252,#13253,#13254,#13255,#13256,#13257,#13258,#13259,
#13260,#13261,#13262,#13263,#13264,#13265),.UNSPECIFIED.,.F.,.F.,(4,3,3,
3,3,3,3,4),(20.1591190625158,20.9674586918964,21.9659091057963,22.9643595196961,
23.9628099335959,24.9612603474957,25.9597107613956,26.4423043696954),
 .UNSPECIFIED.);
#1682=B_SPLINE_CURVE_WITH_KNOTS('',3,(#13266,#13267,#13268,#13269,#13270,
#13271,#13272,#13273,#13274,#13275,#13276,#13277,#13278,#13279,#13280,#13281,
#13282,#13283,#13284,#13285,#13286,#13287),.UNSPECIFIED.,.F.,.F.,(4,3,3,
3,3,3,3,4),(-22.6985303271799,-21.9659091057962,-20.9674586918964,-19.9690082779966,
-18.9705578640968,-17.9721074501969,-16.9736570362971,-16.4153450200003),
 .UNSPECIFIED.);
#1683=B_SPLINE_CURVE_WITH_KNOTS('',3,(#13292,#13293,#13294,#13295,#13296,
#13297,#13298,#13299,#13300,#13301,#13302,#13303,#13304,#13305,#13306,#13307,
#13308,#13309,#13310,#13311,#13312,#13313,#13314,#13315,#13316),
 .UNSPECIFIED.,.F.,.F.,(4,3,3,3,3,3,3,3,4),(13.8759337553362,13.9783057945976,
14.9767562084975,15.9752066223973,16.9736570362971,17.9721074501969,18.9705578640968,
19.9690082779966,20.1591190625158),.UNSPECIFIED.);
#1684=B_SPLINE_CURVE_WITH_KNOTS('',3,(#13317,#13318,#13319,#13320,#13321,
#13322,#13323,#13324,#13325,#13326,#13327,#13328,#13329,#13330,#13331,#13332,
#13333,#13334,#13335,#13336,#13337,#13338),.UNSPECIFIED.,.F.,.F.,(4,3,3,
3,3,3,3,4),(-16.4153450200003,-15.9752066223973,-14.9767562084974,-13.9783057945976,
-12.9798553806978,-11.9814049667979,-10.9829545528981,-10.1321597128207),
 .UNSPECIFIED.);
#1685=B_SPLINE_CURVE_WITH_KNOTS('',3,(#13344,#13345,#13346,#13347,#13348,
#13349,#13350,#13351,#13352,#13353,#13354,#13355,#13356),.UNSPECIFIED.,
 .F.,.F.,(4,3,3,3,4),(-3.84897440564112,-2.99535124169948,-1.99690082779965,
-0.998450413899823,0.),.UNSPECIFIED.);
#1686=B_SPLINE_CURVE_WITH_KNOTS('',3,(#13359,#13360,#13361,#13362,#13363,
#13364,#13365,#13366,#13367,#13368,#13369,#13370,#13371,#13372,#13373,#13374,
#13375,#13376,#13377),.UNSPECIFIED.,.F.,.F.,(4,3,3,3,3,3,4),(2.01694489302834,
2.99535124169949,3.99380165559932,4.99225206949915,5.99070248339898,6.98915289729881,
7.59274844815663),.UNSPECIFIED.);
#1687=B_SPLINE_CURVE_WITH_KNOTS('',3,(#13383,#13384,#13385,#13386,#13387,
#13388,#13389,#13390),.UNSPECIFIED.,.F.,.F.,(4,1,1,1,1,4),(116.238928182822,
116.69628232179,117.69473273569,118.693183149589,119.691633563489,120.690083977389),
 .UNSPECIFIED.);
#1688=B_SPLINE_CURVE_WITH_KNOTS('',3,(#13393,#13394,#13395,#13396,#13397,
#13398,#13399,#13400,#13401),.UNSPECIFIED.,.F.,.F.,(4,1,1,1,1,1,4),(116.238928182822,
116.240342344754,117.238792758654,118.237243172554,119.235693586454,120.234144000354,
121.212550349025),.UNSPECIFIED.);
#1689=B_SPLINE_CURVE_WITH_KNOTS('',3,(#13406,#13407,#13408,#13409,#13410,
#13411,#13412,#13413,#13414,#13415),.UNSPECIFIED.,.F.,.F.,(4,1,1,1,1,1,
1,4),(109.955742875643,110.705579838391,111.704030252291,112.70248066619,
113.70093108009,114.69938149399,115.69783190789,116.238928182822),
 .UNSPECIFIED.);
#1690=B_SPLINE_CURVE_WITH_KNOTS('',3,(#13416,#13417,#13418,#13419,#13420,
#13421,#13422,#13423,#13424,#13425),.UNSPECIFIED.,.F.,.F.,(4,1,1,1,1,1,
1,4),(109.955742875643,110.249639861355,111.248090275255,112.246540689155,
113.244991103055,114.243441516955,115.241891930855,116.238928182822),
 .UNSPECIFIED.);
#1691=B_SPLINE_CURVE_WITH_KNOTS('',3,(#13430,#13431,#13432,#13433,#13434,
#13435,#13436,#13437,#13438,#13439,#13440),.UNSPECIFIED.,.F.,.F.,(4,1,1,
1,1,1,1,1,4),(103.672557568463,103.716426941092,104.714877354992,105.713327768892,
106.711778182792,107.710228596691,108.708679010591,109.707129424491,109.955742875643),
 .UNSPECIFIED.);
#1692=B_SPLINE_CURVE_WITH_KNOTS('',3,(#13441,#13442,#13443,#13444,#13445,
#13446,#13447,#13448,#13449,#13450),.UNSPECIFIED.,.F.,.F.,(4,1,1,1,1,1,
1,4),(103.672557568463,104.258937377956,105.257387791856,106.255838205756,
107.254288619656,108.252739033556,109.251189447456,109.955742875643),
 .UNSPECIFIED.);
#1693=B_SPLINE_CURVE_WITH_KNOTS('',3,(#13455,#13456,#13457,#13458,#13459,
#13460,#13461,#13462,#13463,#13464),.UNSPECIFIED.,.F.,.F.,(4,1,1,1,1,1,
1,4),(97.3893722612836,97.7257244576931,98.7241748715929,99.7226252854927,
100.721075699393,101.719526113292,102.717976527192,103.672557568463),
 .UNSPECIFIED.);
#1694=B_SPLINE_CURVE_WITH_KNOTS('',3,(#13465,#13466,#13467,#13468,#13469,
#13470,#13471,#13472,#13473,#13474),.UNSPECIFIED.,.F.,.F.,(4,1,1,1,1,1,
1,4),(97.3893722612835,98.2682348945574,99.2666853084572,100.265135722357,
101.263586136257,102.262036550157,103.260486964057,103.672557568463),
 .UNSPECIFIED.);
#1695=B_SPLINE_CURVE_WITH_KNOTS('',3,(#13479,#13480,#13481,#13482,#13483,
#13484,#13485,#13486,#13487,#13488),.UNSPECIFIED.,.F.,.F.,(4,1,1,1,1,1,
1,4),(91.106186954104,91.7350219742941,92.7334723881939,93.7319228020937,
94.7303732159936,95.7288236298934,96.7272740437932,97.3893722612836),
 .UNSPECIFIED.);
#1696=B_SPLINE_CURVE_WITH_KNOTS('',3,(#13489,#13490,#13491,#13492,#13493,
#13494,#13495,#13496,#13497,#13498,#13499),.UNSPECIFIED.,.F.,.F.,(4,1,1,
1,1,1,1,1,4),(91.106186954104,91.2790819972586,92.2775324111584,93.2759828250583,
94.2744332389581,95.2728836528579,96.2713340667578,97.2697844806576,97.3893722612835),
 .UNSPECIFIED.);
#1697=B_SPLINE_CURVE_WITH_KNOTS('',3,(#13504,#13505,#13506,#13507,#13508,
#13509,#13510,#13511,#13512,#13513),.UNSPECIFIED.,.F.,.F.,(4,1,1,1,1,1,
1,4),(84.8230016469244,85.7443194908951,86.7427699047949,87.7412203186948,
88.7396707325946,89.7381211464944,90.7365715603943,91.106186954104),
 .UNSPECIFIED.);
#1698=B_SPLINE_CURVE_WITH_KNOTS('',3,(#13514,#13515,#13516,#13517,#13518,
#13519,#13520,#13521,#13522,#13523),.UNSPECIFIED.,.F.,.F.,(4,1,1,1,1,1,
1,4),(84.8230016469244,85.2883795138596,86.2868299277595,87.2852803416593,
88.2837307555591,89.282181169459,90.2806315833588,91.106186954104),
 .UNSPECIFIED.);
#1699=B_SPLINE_CURVE_WITH_KNOTS('',3,(#13528,#13529,#13530,#13531,#13532,
#13533,#13534,#13535,#13536,#13537,#13538),.UNSPECIFIED.,.F.,.F.,(4,1,1,
1,1,1,1,1,4),(78.5398163397448,78.7551665935963,79.7536170074961,80.752067421396,
81.7505178352958,82.7489682491956,83.7474186630954,84.7458690769953,84.8230016469244),
 .UNSPECIFIED.);
#1700=B_SPLINE_CURVE_WITH_KNOTS('',3,(#13539,#13540,#13541,#13542,#13543,
#13544,#13545,#13546,#13547,#13548),.UNSPECIFIED.,.F.,.F.,(4,1,1,1,1,1,
1,4),(78.5398163397448,79.2976770304606,80.2961274443605,81.2945778582603,
82.2930282721601,83.29147868606,84.2899290999598,84.8230016469244),
 .UNSPECIFIED.);
#1701=B_SPLINE_CURVE_WITH_KNOTS('',3,(#13553,#13554,#13555,#13556,#13557,
#13558,#13559,#13560,#13561,#13562),.UNSPECIFIED.,.F.,.F.,(4,1,1,1,1,1,
1,4),(72.2566310325652,72.7644641101973,73.7629145240972,74.761364937997,
75.7598153518968,76.7582657657966,77.7567161796965,78.5398163397448),
 .UNSPECIFIED.);
#1702=B_SPLINE_CURVE_WITH_KNOTS('',3,(#13563,#13564,#13565,#13566,#13567,
#13568,#13569,#13570,#13571,#13572,#13573),.UNSPECIFIED.,.F.,.F.,(4,1,1,
1,1,1,1,1,4),(72.2566310325652,72.3085241331619,73.3069745470617,74.3054249609615,
75.3038753748613,76.3023257887612,77.300776202661,78.2992266165608,78.5398163397448),
 .UNSPECIFIED.);
#1703=B_SPLINE_CURVE_WITH_KNOTS('',3,(#13578,#13579,#13580,#13581,#13582,
#13583,#13584,#13585,#13586,#13587),.UNSPECIFIED.,.F.,.F.,(4,1,1,1,1,1,
1,4),(65.9734457253856,66.7737616267983,67.7722120406982,68.770662454598,
69.7691128684978,70.7675632823977,71.7660136962975,72.2566310325652),
 .UNSPECIFIED.);
#1704=B_SPLINE_CURVE_WITH_KNOTS('',3,(#13588,#13589,#13590,#13591,#13592,
#13593,#13594,#13595,#13596,#13597),.UNSPECIFIED.,.F.,.F.,(4,1,1,1,1,1,
1,4),(65.9734457253856,66.3178216497629,67.3162720636627,68.3147224775625,
69.3131728914624,70.3116233053622,71.310073719262,72.2566310325652),
 .UNSPECIFIED.);
#1705=B_SPLINE_CURVE_WITH_KNOTS('',3,(#13602,#13603,#13604,#13605,#13606,
#13607,#13608,#13609,#13610,#13611,#13612),.UNSPECIFIED.,.F.,.F.,(4,1,1,
1,1,1,1,1,4),(59.690260418206,59.7846087294995,60.7830591433994,61.7815095572992,
62.779959971199,63.7784103850989,64.7768607989987,65.7753112128985,65.9734457253856),
 .UNSPECIFIED.);
#1706=B_SPLINE_CURVE_WITH_KNOTS('',3,(#13613,#13614,#13615,#13616,#13617,
#13618,#13619,#13620,#13621,#13622),.UNSPECIFIED.,.F.,.F.,(4,1,1,1,1,1,
1,4),(59.690260418206,60.3271191663639,61.3255695802637,62.3240199941636,
63.3224704080634,64.3209208219632,65.319371235863,65.9734457253856),
 .UNSPECIFIED.);
#1707=B_SPLINE_CURVE_WITH_KNOTS('',3,(#13627,#13628,#13629,#13630,#13631,
#13632,#13633,#13634,#13635,#13636),.UNSPECIFIED.,.F.,.F.,(4,1,1,1,1,1,
1,4),(53.4070751110264,53.7939062461006,54.7923566600004,55.7908070739002,
56.7892574878,57.7877079016999,58.7861583155997,59.690260418206),
 .UNSPECIFIED.);
#1708=B_SPLINE_CURVE_WITH_KNOTS('',3,(#13637,#13638,#13639,#13640,#13641,
#13642,#13643,#13644,#13645,#13646),.UNSPECIFIED.,.F.,.F.,(4,1,1,1,1,1,
1,4),(53.4070751110264,54.3364166829649,55.3348670968648,56.3333175107646,
57.3317679246644,58.3302183385642,59.3286687524641,59.690260418206),
 .UNSPECIFIED.);
#1709=B_SPLINE_CURVE_WITH_KNOTS('',3,(#13651,#13652,#13653,#13654,#13655,
#13656,#13657,#13658,#13659,#13660),.UNSPECIFIED.,.F.,.F.,(4,1,1,1,1,1,
1,4),(47.1238898038468,47.8032037627016,48.8016541766014,49.8001045905012,
50.7985550044011,51.7970054183009,52.7954558322007,53.4070751110264),
 .UNSPECIFIED.);
#1710=B_SPLINE_CURVE_WITH_KNOTS('',3,(#13661,#13662,#13663,#13664,#13665,
#13666,#13667,#13668,#13669,#13670,#13671),.UNSPECIFIED.,.F.,.F.,(4,1,1,
1,1,1,1,1,4),(47.1238898038468,47.3472637856661,48.3457141995659,49.3441646134658,
50.3426150273656,51.3410654412654,52.3395158551653,53.3379662690651,53.4070751110264),
 .UNSPECIFIED.);
#1711=B_SPLINE_CURVE_WITH_KNOTS('',3,(#13676,#13677,#13678,#13679,#13680,
#13681,#13682,#13683,#13684,#13685),.UNSPECIFIED.,.F.,.F.,(4,1,1,1,1,1,
1,4),(40.8407044966672,41.8125012793026,42.8109516932024,43.8094021071023,
44.8078525210021,45.8063029349019,46.8047533488018,47.1238898038468),
 .UNSPECIFIED.);
#1712=B_SPLINE_CURVE_WITH_KNOTS('',3,(#13686,#13687,#13688,#13689,#13690,
#13691,#13692,#13693,#13694,#13695),.UNSPECIFIED.,.F.,.F.,(4,1,1,1,1,1,
1,4),(40.8407044966672,41.3565613022671,42.355011716167,43.3534621300668,
44.3519125439666,45.3503629578665,46.3488133717663,47.1238898038468),
 .UNSPECIFIED.);
#1713=B_SPLINE_CURVE_WITH_KNOTS('',3,(#13700,#13701,#13702,#13703,#13704,
#13705,#13706,#13707,#13708,#13709,#13710),.UNSPECIFIED.,.F.,.F.,(4,1,1,
1,1,1,1,1,4),(34.5575191894876,34.8233483820038,35.8217987959036,36.8202492098035,
37.8186996237033,38.8171500376031,39.8156004515029,40.8140508654028,40.8407044966672),
 .UNSPECIFIED.);
#1714=B_SPLINE_CURVE_WITH_KNOTS('',3,(#13711,#13712,#13713,#13714,#13715,
#13716,#13717,#13718,#13719,#13720),.UNSPECIFIED.,.F.,.F.,(4,1,1,1,1,1,
1,4),(34.5575191894876,35.3658588188682,36.364309232768,37.3627596466678,
38.3612100605677,39.3596604744675,40.3581108883673,40.8407044966672),
 .UNSPECIFIED.);
#1715=B_SPLINE_CURVE_WITH_KNOTS('',3,(#13725,#13726,#13727,#13728,#13729,
#13730,#13731,#13732,#13733,#13734),.UNSPECIFIED.,.F.,.F.,(4,1,1,1,1,1,
1,4),(28.274333882308,28.8326458986048,29.8310963125047,30.8295467264045,
31.8279971403043,32.8264475542041,33.824897968104,34.5575191894876),
 .UNSPECIFIED.);
#1716=B_SPLINE_CURVE_WITH_KNOTS('',3,(#13735,#13736,#13737,#13738,#13739,
#13740,#13741,#13742,#13743,#13744,#13745),.UNSPECIFIED.,.F.,.F.,(4,1,1,
1,1,1,1,1,4),(28.274333882308,28.3767059215694,29.3751563354692,30.373606749369,
31.3720571632688,32.3705075771687,33.3689579910685,34.3674084049683,34.5575191894876),
 .UNSPECIFIED.);
#1717=B_SPLINE_CURVE_WITH_KNOTS('',3,(#13750,#13751,#13752,#13753,#13754,
#13755,#13756,#13757,#13758,#13759),.UNSPECIFIED.,.F.,.F.,(4,1,1,1,1,1,
1,4),(21.9911485751285,22.8419434152058,23.8403938291057,24.8388442430055,
25.8372946569053,26.8357450708052,27.834195484705,28.274333882308),
 .UNSPECIFIED.);
#1718=B_SPLINE_CURVE_WITH_KNOTS('',3,(#13760,#13761,#13762,#13763,#13764,
#13765,#13766,#13767,#13768,#13769),.UNSPECIFIED.,.F.,.F.,(4,1,1,1,1,1,
1,4),(21.9911485751285,22.3860034381704,23.3844538520702,24.38290426597,
25.3813546798699,26.3798050937697,27.3782555076695,28.274333882308),
 .UNSPECIFIED.);
#1719=B_SPLINE_CURVE_WITH_KNOTS('',3,(#13775,#13776,#13777,#13778,#13779),
 .UNSPECIFIED.,.F.,.F.,(4,1,4),(14.3984001269717,15.3968505408716,15.7079632679489),
 .UNSPECIFIED.);
#1720=B_SPLINE_CURVE_WITH_KNOTS('',3,(#13782,#13783,#13784,#13785,#13786),
 .UNSPECIFIED.,.F.,.F.,(4,1,4),(13.8759337553362,14.8543401040072,15.7079632679489),
 .UNSPECIFIED.);
#1721=B_SPLINE_CURVE_WITH_KNOTS('',3,(#13792,#13793,#13794,#13795),
 .UNSPECIFIED.,.F.,.F.,(4,4),(108.12371336303,108.831095115081),
 .UNSPECIFIED.);
#1722=B_SPLINE_CURVE_WITH_KNOTS('',3,(#13803,#13804,#13805,#13806,#13807,
#13808,#13809,#13810,#13811,#13812),.UNSPECIFIED.,.F.,.F.,(4,3,3,4),(-106.814150222053,
-105.835743873382,-104.837293459482,-104.379939320515),.UNSPECIFIED.);
#1723=B_SPLINE_CURVE_WITH_KNOTS('',3,(#13817,#13818,#13819,#13820,#13821,
#13822,#13823,#13824,#13825,#13826,#13827,#13828,#13829,#13830,#13831,#13832,
#13833,#13834,#13835,#13836,#13837,#13838),.UNSPECIFIED.,.F.,.F.,(4,3,3,
3,3,3,3,4),(101.84052805585,102.840392631682,103.838843045582,104.837293459482,
105.835743873382,106.834194287282,107.832644701182,108.12371336303),
 .UNSPECIFIED.);
#1724=B_SPLINE_CURVE_WITH_KNOTS('',3,(#13839,#13840,#13841,#13842,#13843,
#13844,#13845,#13846,#13847,#13848,#13849,#13850,#13851,#13852,#13853,#13854,
#13855,#13856,#13857,#13858,#13859,#13860),.UNSPECIFIED.,.F.,.F.,(4,3,3,
3,3,3,3,4),(-104.379939320515,-103.838843045582,-102.840392631682,-101.841942217783,
-100.843491803883,-99.8450413899829,-98.8465909760831,-98.096754013335),
 .UNSPECIFIED.);
#1725=B_SPLINE_CURVE_WITH_KNOTS('',3,(#13865,#13866,#13867,#13868,#13869,
#13870,#13871,#13872,#13873,#13874,#13875,#13876,#13877,#13878,#13879,#13880,
#13881,#13882,#13883,#13884,#13885,#13886),.UNSPECIFIED.,.F.,.F.,(4,3,3,
3,3,3,3,4),(95.5573427486709,95.8512397343836,96.8496901482835,97.8481405621833,
98.8465909760831,99.8450413899829,100.843491803883,101.84052805585),
 .UNSPECIFIED.);
#1726=B_SPLINE_CURVE_WITH_KNOTS('',3,(#13887,#13888,#13889,#13890,#13891,
#13892,#13893,#13894,#13895,#13896,#13897,#13898,#13899,#13900,#13901,#13902,
#13903,#13904,#13905,#13906,#13907,#13908,#13909,#13910,#13911),
 .UNSPECIFIED.,.F.,.F.,(4,3,3,3,3,3,3,3,4),(-98.096754013335,-97.8481405621833,
-96.8496901482834,-95.8512397343836,-94.8527893204838,-93.854338906584,
-92.8558884926841,-91.8574380787843,-91.8135687061554),.UNSPECIFIED.);
#1727=B_SPLINE_CURVE_WITH_KNOTS('',3,(#13916,#13917,#13918,#13919,#13920,
#13921,#13922,#13923,#13924,#13925,#13926,#13927,#13928,#13929,#13930,#13931,
#13932,#13933,#13934,#13935,#13936,#13937),.UNSPECIFIED.,.F.,.F.,(4,3,3,
3,3,3,3,4),(89.2741574414913,89.8605372509847,90.8589876648845,91.8574380787843,
92.8558884926841,93.854338906584,94.8527893204838,95.5573427486709),
 .UNSPECIFIED.);
#1728=B_SPLINE_CURVE_WITH_KNOTS('',3,(#13938,#13939,#13940,#13941,#13942,
#13943,#13944,#13945,#13946,#13947,#13948,#13949,#13950,#13951,#13952,#13953,
#13954,#13955,#13956,#13957,#13958,#13959),.UNSPECIFIED.,.F.,.F.,(4,3,3,
3,3,3,3,4),(-91.8135687061554,-90.8589876648845,-89.8605372509847,-88.8620868370848,
-87.863636423185,-86.8651860092852,-85.8667355953853,-85.5303833989758),
 .UNSPECIFIED.);
#1729=B_SPLINE_CURVE_WITH_KNOTS('',3,(#13964,#13965,#13966,#13967,#13968,
#13969,#13970,#13971,#13972,#13973,#13974,#13975,#13976,#13977,#13978,#13979,
#13980,#13981,#13982,#13983,#13984,#13985),.UNSPECIFIED.,.F.,.F.,(4,3,3,
3,3,3,3,4),(82.9909721343117,83.8698347675857,84.8682851814855,85.8667355953854,
86.8651860092852,87.863636423185,88.8620868370848,89.2741574414913),
 .UNSPECIFIED.);
#1730=B_SPLINE_CURVE_WITH_KNOTS('',3,(#13986,#13987,#13988,#13989,#13990,
#13991,#13992,#13993,#13994,#13995,#13996,#13997,#13998,#13999,#14000,#14001,
#14002,#14003,#14004,#14005,#14006,#14007),.UNSPECIFIED.,.F.,.F.,(4,3,3,
3,3,3,3,4),(-85.5303833989758,-84.8682851814855,-83.8698347675857,-82.8713843536859,
-81.872933939786,-80.8744835258862,-79.8760331119863,-79.2471980917962),
 .UNSPECIFIED.);
#1731=B_SPLINE_CURVE_WITH_KNOTS('',3,(#14012,#14013,#14014,#14015,#14016,
#14017,#14018,#14019,#14020,#14021,#14022,#14023,#14024,#14025,#14026,#14027,
#14028,#14029,#14030,#14031,#14032,#14033,#14034,#14035,#14036),
 .UNSPECIFIED.,.F.,.F.,(4,3,3,3,3,3,3,3,4),(76.7077868271321,76.8806818702869,
77.8791322841867,78.8775826980865,79.8760331119864,80.8744835258862,81.872933939786,
82.8713843536859,82.9909721343117),.UNSPECIFIED.);
#1732=B_SPLINE_CURVE_WITH_KNOTS('',3,(#14037,#14038,#14039,#14040,#14041,
#14042,#14043,#14044,#14045,#14046,#14047,#14048,#14049,#14050,#14051,#14052,
#14053,#14054,#14055,#14056,#14057,#14058),.UNSPECIFIED.,.F.,.F.,(4,3,3,
3,3,3,3,4),(-79.2471980917962,-78.8775826980865,-77.8791322841867,-76.8806818702869,
-75.882231456387,-74.8837810424872,-73.8853306285874,-72.9640127846166),
 .UNSPECIFIED.);
#1733=B_SPLINE_CURVE_WITH_KNOTS('',3,(#14063,#14064,#14065,#14066,#14067,
#14068,#14069,#14070,#14071,#14072,#14073,#14074,#14075,#14076,#14077,#14078,
#14079,#14080,#14081,#14082,#14083,#14084),.UNSPECIFIED.,.F.,.F.,(4,3,3,
3,3,3,3,4),(70.4246015199525,70.8899793868879,71.8884298007877,72.8868802146876,
73.8853306285874,74.8837810424872,75.882231456387,76.7077868271321),
 .UNSPECIFIED.);
#1734=B_SPLINE_CURVE_WITH_KNOTS('',3,(#14085,#14086,#14087,#14088,#14089,
#14090,#14091,#14092,#14093,#14094,#14095,#14096,#14097,#14098,#14099,#14100,
#14101,#14102,#14103,#14104,#14105,#14106,#14107,#14108,#14109),
 .UNSPECIFIED.,.F.,.F.,(4,3,3,3,3,3,3,3,4),(-72.9640127846166,-72.8868802146875,
-71.8884298007877,-70.8899793868879,-69.891528972988,-68.8930785590882,
-67.8946281451884,-66.8961777312885,-66.680827477437),.UNSPECIFIED.);
#1735=B_SPLINE_CURVE_WITH_KNOTS('',3,(#14114,#14115,#14116,#14117,#14118,
#14119,#14120,#14121,#14122,#14123,#14124,#14125,#14126,#14127,#14128,#14129,
#14130,#14131,#14132,#14133,#14134,#14135),.UNSPECIFIED.,.F.,.F.,(4,3,3,
3,3,3,3,4),(64.1414162127729,64.8992769034889,65.8977273173887,66.8961777312886,
67.8946281451884,68.8930785590882,69.8915289729881,70.4246015199525),
 .UNSPECIFIED.);
#1736=B_SPLINE_CURVE_WITH_KNOTS('',3,(#14136,#14137,#14138,#14139,#14140,
#14141,#14142,#14143,#14144,#14145,#14146,#14147,#14148,#14149,#14150,#14151,
#14152,#14153,#14154,#14155,#14156,#14157),.UNSPECIFIED.,.F.,.F.,(4,3,3,
3,3,3,3,4),(-66.680827477437,-65.8977273173887,-64.8992769034889,-63.9008264895891,
-62.9023760756893,-61.9039256617894,-60.9054752478896,-60.3976421702574),
 .UNSPECIFIED.);
#1737=B_SPLINE_CURVE_WITH_KNOTS('',3,(#14162,#14163,#14164,#14165,#14166,
#14167,#14168,#14169,#14170,#14171,#14172,#14173,#14174,#14175,#14176,#14177,
#14178,#14179,#14180,#14181,#14182,#14183,#14184,#14185,#14186),
 .UNSPECIFIED.,.F.,.F.,(4,3,3,3,3,3,3,3,4),(57.8582309055933,57.9101240061901,
58.9085744200899,59.9070248339898,60.9054752478896,61.9039256617894,62.9023760756893,
63.9008264895891,64.1414162127729),.UNSPECIFIED.);
#1738=B_SPLINE_CURVE_WITH_KNOTS('',3,(#14187,#14188,#14189,#14190,#14191,
#14192,#14193,#14194,#14195,#14196,#14197,#14198,#14199,#14200,#14201,#14202,
#14203,#14204,#14205,#14206,#14207,#14208),.UNSPECIFIED.,.F.,.F.,(4,3,3,
3,3,3,3,4),(-60.3976421702574,-59.9070248339898,-58.9085744200899,-57.9101240061901,
-56.9116735922903,-55.9132231783905,-54.9147727644906,-54.1144568630778),
 .UNSPECIFIED.);
#1739=B_SPLINE_CURVE_WITH_KNOTS('',3,(#14213,#14214,#14215,#14216,#14217,
#14218,#14219,#14220,#14221,#14222,#14223,#14224,#14225,#14226,#14227,#14228,
#14229,#14230,#14231,#14232,#14233,#14234),.UNSPECIFIED.,.F.,.F.,(4,3,3,
3,3,3,3,4),(51.5750455984138,51.9194215227911,52.917871936691,53.9163223505908,
54.9147727644906,55.9132231783905,56.9116735922903,57.8582309055933),
 .UNSPECIFIED.);
#1740=B_SPLINE_CURVE_WITH_KNOTS('',3,(#14235,#14236,#14237,#14238,#14239,
#14240,#14241,#14242,#14243,#14244,#14245,#14246,#14247,#14248,#14249,#14250,
#14251,#14252,#14253,#14254,#14255,#14256,#14257,#14258,#14259),
 .UNSPECIFIED.,.F.,.F.,(4,3,3,3,3,3,3,3,4),(-54.1144568630778,-53.9163223505908,
-52.917871936691,-51.9194215227911,-50.9209711088913,-49.9225206949915,
-48.9240702810916,-47.9256198671918,-47.8312715558982),.UNSPECIFIED.);
#1741=B_SPLINE_CURVE_WITH_KNOTS('',3,(#14264,#14265,#14266,#14267,#14268,
#14269,#14270,#14271,#14272,#14273,#14274,#14275,#14276,#14277,#14278,#14279,
#14280,#14281,#14282,#14283,#14284,#14285),.UNSPECIFIED.,.F.,.F.,(4,3,3,
3,3,3,3,4),(45.2918602912342,45.9287190393922,46.927169453292,47.9256198671918,
48.9240702810917,49.9225206949915,50.9209711088913,51.5750455984138),
 .UNSPECIFIED.);
#1742=B_SPLINE_CURVE_WITH_KNOTS('',3,(#14286,#14287,#14288,#14289,#14290,
#14291,#14292,#14293,#14294,#14295,#14296,#14297,#14298,#14299,#14300,#14301,
#14302,#14303,#14304,#14305,#14306,#14307),.UNSPECIFIED.,.F.,.F.,(4,3,3,
3,3,3,3,4),(-47.8312715558982,-46.927169453292,-45.9287190393921,-44.9302686254923,
-43.9318182115925,-42.9333677976927,-41.9349173837928,-41.5480862487187),
 .UNSPECIFIED.);
#1743=B_SPLINE_CURVE_WITH_KNOTS('',3,(#14312,#14313,#14314,#14315,#14316,
#14317,#14318,#14319,#14320,#14321,#14322,#14323,#14324,#14325,#14326,#14327,
#14328,#14329,#14330,#14331,#14332,#14333),.UNSPECIFIED.,.F.,.F.,(4,3,3,
3,3,3,3,4),(39.0086749840546,39.9380165559932,40.936466969893,41.9349173837928,
42.9333677976927,43.9318182115925,44.9302686254923,45.2918602912342),
 .UNSPECIFIED.);
#1744=B_SPLINE_CURVE_WITH_KNOTS('',3,(#14334,#14335,#14336,#14337,#14338,
#14339,#14340,#14341,#14342,#14343,#14344,#14345,#14346,#14347,#14348,#14349,
#14350,#14351,#14352,#14353,#14354,#14355),.UNSPECIFIED.,.F.,.F.,(4,3,3,
3,3,3,3,4),(-41.5480862487187,-40.936466969893,-39.9380165559932,-38.9395661420933,
-37.9411157281935,-36.9426653142937,-35.9442149003939,-35.2649009415391),
 .UNSPECIFIED.);
#1745=B_SPLINE_CURVE_WITH_KNOTS('',3,(#14360,#14361,#14362,#14363,#14364,
#14365,#14366,#14367,#14368,#14369,#14370,#14371,#14372,#14373,#14374,#14375,
#14376,#14377,#14378,#14379,#14380,#14381,#14382,#14383,#14384),
 .UNSPECIFIED.,.F.,.F.,(4,3,3,3,3,3,3,3,4),(32.725489676875,32.9488636586944,
33.9473140725942,34.945764486494,35.9442149003939,36.9426653142937,37.9411157281935,
38.9395661420934,39.0086749840546),.UNSPECIFIED.);
#1746=B_SPLINE_CURVE_WITH_KNOTS('',3,(#14385,#14386,#14387,#14388,#14389,
#14390,#14391,#14392,#14393,#14394,#14395,#14396,#14397,#14398,#14399,#14400,
#14401,#14402,#14403,#14404,#14405,#14406),.UNSPECIFIED.,.F.,.F.,(4,3,3,
3,3,3,3,4),(-35.2649009415391,-34.945764486494,-33.9473140725942,-32.9488636586944,
-31.9504132447945,-30.9519628308947,-29.9535124169949,-28.9817156343595),
 .UNSPECIFIED.);
#1747=B_SPLINE_CURVE_WITH_KNOTS('',3,(#14411,#14412,#14413,#14414,#14415,
#14416,#14417,#14418,#14419,#14420,#14421,#14422,#14423,#14424,#14425,#14426,
#14427,#14428,#14429,#14430,#14431,#14432),.UNSPECIFIED.,.F.,.F.,(4,3,3,
3,3,3,3,4),(26.4423043696954,26.9581611752954,27.9566115891952,28.9550620030951,
29.9535124169949,30.9519628308947,31.9504132447945,32.725489676875),
 .UNSPECIFIED.);
#1748=B_SPLINE_CURVE_WITH_KNOTS('',3,(#14433,#14434,#14435,#14436,#14437,
#14438,#14439,#14440,#14441,#14442,#14443,#14444,#14445,#14446,#14447,#14448,
#14449,#14450,#14451,#14452,#14453,#14454,#14455,#14456,#14457),
 .UNSPECIFIED.,.F.,.F.,(4,3,3,3,3,3,3,3,4),(-28.9817156343595,-28.955062003095,
-27.9566115891952,-26.9581611752954,-25.9597107613956,-24.9612603474957,
-23.9628099335959,-22.9643595196961,-22.6985303271799),.UNSPECIFIED.);
#1749=B_SPLINE_CURVE_WITH_KNOTS('',3,(#14462,#14463,#14464,#14465,#14466,
#14467,#14468,#14469,#14470,#14471,#14472,#14473,#14474,#14475,#14476,#14477,
#14478,#14479,#14480,#14481,#14482,#14483),.UNSPECIFIED.,.F.,.F.,(4,3,3,
3,3,3,3,4),(20.1591190625158,20.9674586918964,21.9659091057962,22.9643595196961,
23.9628099335959,24.9612603474957,25.9597107613956,26.4423043696954),
 .UNSPECIFIED.);
#1750=B_SPLINE_CURVE_WITH_KNOTS('',3,(#14484,#14485,#14486,#14487,#14488,
#14489,#14490,#14491,#14492,#14493,#14494,#14495,#14496,#14497,#14498,#14499,
#14500,#14501,#14502,#14503,#14504,#14505),.UNSPECIFIED.,.F.,.F.,(4,3,3,
3,3,3,3,4),(-22.6985303271799,-21.9659091057962,-20.9674586918964,-19.9690082779966,
-18.9705578640968,-17.9721074501969,-16.9736570362971,-16.4153450200003),
 .UNSPECIFIED.);
#1751=B_SPLINE_CURVE_WITH_KNOTS('',3,(#14510,#14511,#14512,#14513,#14514,
#14515,#14516,#14517,#14518,#14519,#14520,#14521,#14522,#14523,#14524,#14525,
#14526,#14527,#14528,#14529,#14530,#14531,#14532,#14533,#14534),
 .UNSPECIFIED.,.F.,.F.,(4,3,3,3,3,3,3,3,4),(13.8759337553362,13.9783057945976,
14.9767562084974,15.9752066223973,16.9736570362971,17.9721074501969,18.9705578640968,
19.9690082779966,20.1591190625158),.UNSPECIFIED.);
#1752=B_SPLINE_CURVE_WITH_KNOTS('',3,(#14535,#14536,#14537,#14538,#14539,
#14540,#14541,#14542,#14543,#14544,#14545,#14546,#14547,#14548,#14549,#14550,
#14551,#14552,#14553,#14554,#14555,#14556),.UNSPECIFIED.,.F.,.F.,(4,3,3,
3,3,3,3,4),(-16.4153450200003,-15.9752066223973,-14.9767562084974,-13.9783057945976,
-12.9798553806978,-11.9814049667979,-10.9829545528981,-10.1321597128207),
 .UNSPECIFIED.);
#1753=B_SPLINE_CURVE_WITH_KNOTS('',3,(#14562,#14563,#14564,#14565,#14566,
#14567,#14568,#14569,#14570,#14571,#14572,#14573,#14574),.UNSPECIFIED.,
 .F.,.F.,(4,3,3,3,4),(-3.84897440564114,-2.99535124169949,-1.99690082779966,
-0.99845041389983,0.),.UNSPECIFIED.);
#1754=B_SPLINE_CURVE_WITH_KNOTS('',3,(#14577,#14578,#14579,#14580,#14581,
#14582,#14583,#14584,#14585,#14586,#14587,#14588,#14589,#14590,#14591,#14592,
#14593,#14594,#14595),.UNSPECIFIED.,.F.,.F.,(4,3,3,3,3,3,4),(2.01694489302824,
2.99535124169949,3.99380165559932,4.99225206949915,5.99070248339898,6.98915289729881,
7.59274844815663),.UNSPECIFIED.);
#1755=B_SPLINE_CURVE_WITH_KNOTS('',3,(#14601,#14602,#14603,#14604,#14605,
#14606,#14607,#14608),.UNSPECIFIED.,.F.,.F.,(4,1,1,1,1,4),(116.238928182822,
116.69628232179,117.69473273569,118.693183149589,119.691633563489,120.690083977389),
 .UNSPECIFIED.);
#1756=B_SPLINE_CURVE_WITH_KNOTS('',3,(#14611,#14612,#14613,#14614,#14615,
#14616,#14617,#14618,#14619),.UNSPECIFIED.,.F.,.F.,(4,1,1,1,1,1,4),(116.238928182822,
116.240342344754,117.238792758654,118.237243172554,119.235693586454,120.234144000354,
121.212550349025),.UNSPECIFIED.);
#1757=B_SPLINE_CURVE_WITH_KNOTS('',3,(#14624,#14625,#14626,#14627,#14628,
#14629,#14630,#14631,#14632,#14633),.UNSPECIFIED.,.F.,.F.,(4,1,1,1,1,1,
1,4),(109.955742875643,110.705579838391,111.704030252291,112.70248066619,
113.70093108009,114.69938149399,115.69783190789,116.238928182822),
 .UNSPECIFIED.);
#1758=B_SPLINE_CURVE_WITH_KNOTS('',3,(#14634,#14635,#14636,#14637,#14638,
#14639,#14640,#14641,#14642,#14643),.UNSPECIFIED.,.F.,.F.,(4,1,1,1,1,1,
1,4),(109.955742875643,110.249639861355,111.248090275255,112.246540689155,
113.244991103055,114.243441516955,115.241891930855,116.238928182822),
 .UNSPECIFIED.);
#1759=B_SPLINE_CURVE_WITH_KNOTS('',3,(#14648,#14649,#14650,#14651,#14652,
#14653,#14654,#14655,#14656,#14657,#14658),.UNSPECIFIED.,.F.,.F.,(4,1,1,
1,1,1,1,1,4),(103.672557568463,103.716426941092,104.714877354992,105.713327768892,
106.711778182792,107.710228596691,108.708679010591,109.707129424491,109.955742875643),
 .UNSPECIFIED.);
#1760=B_SPLINE_CURVE_WITH_KNOTS('',3,(#14659,#14660,#14661,#14662,#14663,
#14664,#14665,#14666,#14667,#14668),.UNSPECIFIED.,.F.,.F.,(4,1,1,1,1,1,
1,4),(103.672557568463,104.258937377956,105.257387791856,106.255838205756,
107.254288619656,108.252739033556,109.251189447456,109.955742875643),
 .UNSPECIFIED.);
#1761=B_SPLINE_CURVE_WITH_KNOTS('',3,(#14673,#14674,#14675,#14676,#14677,
#14678,#14679,#14680,#14681,#14682),.UNSPECIFIED.,.F.,.F.,(4,1,1,1,1,1,
1,4),(97.3893722612835,97.725724457693,98.7241748715929,99.7226252854927,
100.721075699393,101.719526113292,102.717976527192,103.672557568463),
 .UNSPECIFIED.);
#1762=B_SPLINE_CURVE_WITH_KNOTS('',3,(#14683,#14684,#14685,#14686,#14687,
#14688,#14689,#14690,#14691,#14692),.UNSPECIFIED.,.F.,.F.,(4,1,1,1,1,1,
1,4),(97.3893722612835,98.2682348945574,99.2666853084572,100.265135722357,
101.263586136257,102.262036550157,103.260486964057,103.672557568463),
 .UNSPECIFIED.);
#1763=B_SPLINE_CURVE_WITH_KNOTS('',3,(#14697,#14698,#14699,#14700,#14701,
#14702,#14703,#14704,#14705,#14706),.UNSPECIFIED.,.F.,.F.,(4,1,1,1,1,1,
1,4),(91.106186954104,91.7350219742941,92.7334723881939,93.7319228020937,
94.7303732159936,95.7288236298934,96.7272740437932,97.3893722612835),
 .UNSPECIFIED.);
#1764=B_SPLINE_CURVE_WITH_KNOTS('',3,(#14707,#14708,#14709,#14710,#14711,
#14712,#14713,#14714,#14715,#14716,#14717),.UNSPECIFIED.,.F.,.F.,(4,1,1,
1,1,1,1,1,4),(91.106186954104,91.2790819972586,92.2775324111584,93.2759828250583,
94.2744332389581,95.2728836528579,96.2713340667578,97.2697844806576,97.3893722612835),
 .UNSPECIFIED.);
#1765=B_SPLINE_CURVE_WITH_KNOTS('',3,(#14722,#14723,#14724,#14725,#14726,
#14727,#14728,#14729,#14730,#14731),.UNSPECIFIED.,.F.,.F.,(4,1,1,1,1,1,
1,4),(84.8230016469244,85.7443194908951,86.7427699047949,87.7412203186948,
88.7396707325946,89.7381211464944,90.7365715603942,91.106186954104),
 .UNSPECIFIED.);
#1766=B_SPLINE_CURVE_WITH_KNOTS('',3,(#14732,#14733,#14734,#14735,#14736,
#14737,#14738,#14739,#14740,#14741),.UNSPECIFIED.,.F.,.F.,(4,1,1,1,1,1,
1,4),(84.8230016469244,85.2883795138596,86.2868299277595,87.2852803416593,
88.2837307555591,89.282181169459,90.2806315833588,91.106186954104),
 .UNSPECIFIED.);
#1767=B_SPLINE_CURVE_WITH_KNOTS('',3,(#14746,#14747,#14748,#14749,#14750,
#14751,#14752,#14753,#14754,#14755,#14756),.UNSPECIFIED.,.F.,.F.,(4,1,1,
1,1,1,1,1,4),(78.5398163397448,78.7551665935963,79.7536170074961,80.7520674213959,
81.7505178352958,82.7489682491956,83.7474186630954,84.7458690769953,84.8230016469244),
 .UNSPECIFIED.);
#1768=B_SPLINE_CURVE_WITH_KNOTS('',3,(#14757,#14758,#14759,#14760,#14761,
#14762,#14763,#14764,#14765,#14766),.UNSPECIFIED.,.F.,.F.,(4,1,1,1,1,1,
1,4),(78.5398163397448,79.2976770304607,80.2961274443605,81.2945778582603,
82.2930282721601,83.29147868606,84.2899290999598,84.8230016469244),
 .UNSPECIFIED.);
#1769=B_SPLINE_CURVE_WITH_KNOTS('',3,(#14771,#14772,#14773,#14774,#14775,
#14776,#14777,#14778,#14779,#14780),.UNSPECIFIED.,.F.,.F.,(4,1,1,1,1,1,
1,4),(72.2566310325652,72.7644641101973,73.7629145240971,74.761364937997,
75.7598153518968,76.7582657657966,77.7567161796965,78.5398163397448),
 .UNSPECIFIED.);
#1770=B_SPLINE_CURVE_WITH_KNOTS('',3,(#14781,#14782,#14783,#14784,#14785,
#14786,#14787,#14788,#14789,#14790,#14791),.UNSPECIFIED.,.F.,.F.,(4,1,1,
1,1,1,1,1,4),(72.2566310325652,72.3085241331619,73.3069745470617,74.3054249609615,
75.3038753748613,76.3023257887612,77.300776202661,78.2992266165608,78.5398163397448),
 .UNSPECIFIED.);
#1771=B_SPLINE_CURVE_WITH_KNOTS('',3,(#14796,#14797,#14798,#14799,#14800,
#14801,#14802,#14803,#14804,#14805),.UNSPECIFIED.,.F.,.F.,(4,1,1,1,1,1,
1,4),(65.9734457253856,66.7737616267983,67.7722120406982,68.770662454598,
69.7691128684978,70.7675632823977,71.7660136962975,72.2566310325652),
 .UNSPECIFIED.);
#1772=B_SPLINE_CURVE_WITH_KNOTS('',3,(#14806,#14807,#14808,#14809,#14810,
#14811,#14812,#14813,#14814,#14815),.UNSPECIFIED.,.F.,.F.,(4,1,1,1,1,1,
1,4),(65.9734457253856,66.3178216497629,67.3162720636627,68.3147224775625,
69.3131728914624,70.3116233053622,71.310073719262,72.2566310325652),
 .UNSPECIFIED.);
#1773=B_SPLINE_CURVE_WITH_KNOTS('',3,(#14820,#14821,#14822,#14823,#14824,
#14825,#14826,#14827,#14828,#14829,#14830),.UNSPECIFIED.,.F.,.F.,(4,1,1,
1,1,1,1,1,4),(59.690260418206,59.7846087294995,60.7830591433994,61.7815095572992,
62.779959971199,63.7784103850989,64.7768607989987,65.7753112128985,65.9734457253856),
 .UNSPECIFIED.);
#1774=B_SPLINE_CURVE_WITH_KNOTS('',3,(#14831,#14832,#14833,#14834,#14835,
#14836,#14837,#14838,#14839,#14840),.UNSPECIFIED.,.F.,.F.,(4,1,1,1,1,1,
1,4),(59.690260418206,60.3271191663639,61.3255695802637,62.3240199941636,
63.3224704080634,64.3209208219632,65.319371235863,65.9734457253856),
 .UNSPECIFIED.);
#1775=B_SPLINE_CURVE_WITH_KNOTS('',3,(#14845,#14846,#14847,#14848,#14849,
#14850,#14851,#14852,#14853,#14854),.UNSPECIFIED.,.F.,.F.,(4,1,1,1,1,1,
1,4),(53.4070751110264,53.7939062461006,54.7923566600004,55.7908070739002,
56.7892574878001,57.7877079016999,58.7861583155997,59.690260418206),
 .UNSPECIFIED.);
#1776=B_SPLINE_CURVE_WITH_KNOTS('',3,(#14855,#14856,#14857,#14858,#14859,
#14860,#14861,#14862,#14863,#14864),.UNSPECIFIED.,.F.,.F.,(4,1,1,1,1,1,
1,4),(53.4070751110264,54.3364166829649,55.3348670968648,56.3333175107646,
57.3317679246644,58.3302183385642,59.3286687524641,59.690260418206),
 .UNSPECIFIED.);
#1777=B_SPLINE_CURVE_WITH_KNOTS('',3,(#14869,#14870,#14871,#14872,#14873,
#14874,#14875,#14876,#14877,#14878),.UNSPECIFIED.,.F.,.F.,(4,1,1,1,1,1,
1,4),(47.1238898038468,47.8032037627016,48.8016541766014,49.8001045905012,
50.7985550044011,51.7970054183009,52.7954558322007,53.4070751110264),
 .UNSPECIFIED.);
#1778=B_SPLINE_CURVE_WITH_KNOTS('',3,(#14879,#14880,#14881,#14882,#14883,
#14884,#14885,#14886,#14887,#14888,#14889),.UNSPECIFIED.,.F.,.F.,(4,1,1,
1,1,1,1,1,4),(47.1238898038468,47.3472637856661,48.3457141995659,49.3441646134658,
50.3426150273656,51.3410654412654,52.3395158551653,53.3379662690651,53.4070751110264),
 .UNSPECIFIED.);
#1779=B_SPLINE_CURVE_WITH_KNOTS('',3,(#14894,#14895,#14896,#14897,#14898,
#14899,#14900,#14901,#14902,#14903),.UNSPECIFIED.,.F.,.F.,(4,1,1,1,1,1,
1,4),(40.8407044966672,41.8125012793026,42.8109516932024,43.8094021071023,
44.8078525210021,45.8063029349019,46.8047533488018,47.1238898038468),
 .UNSPECIFIED.);
#1780=B_SPLINE_CURVE_WITH_KNOTS('',3,(#14904,#14905,#14906,#14907,#14908,
#14909,#14910,#14911,#14912,#14913),.UNSPECIFIED.,.F.,.F.,(4,1,1,1,1,1,
1,4),(40.8407044966672,41.3565613022671,42.355011716167,43.3534621300668,
44.3519125439666,45.3503629578665,46.3488133717663,47.1238898038468),
 .UNSPECIFIED.);
#1781=B_SPLINE_CURVE_WITH_KNOTS('',3,(#14918,#14919,#14920,#14921,#14922,
#14923,#14924,#14925,#14926,#14927,#14928),.UNSPECIFIED.,.F.,.F.,(4,1,1,
1,1,1,1,1,4),(34.5575191894876,34.8233483820038,35.8217987959036,36.8202492098035,
37.8186996237033,38.8171500376031,39.8156004515029,40.8140508654028,40.8407044966672),
 .UNSPECIFIED.);
#1782=B_SPLINE_CURVE_WITH_KNOTS('',3,(#14929,#14930,#14931,#14932,#14933,
#14934,#14935,#14936,#14937,#14938),.UNSPECIFIED.,.F.,.F.,(4,1,1,1,1,1,
1,4),(34.5575191894876,35.3658588188682,36.364309232768,37.3627596466678,
38.3612100605677,39.3596604744675,40.3581108883673,40.8407044966672),
 .UNSPECIFIED.);
#1783=B_SPLINE_CURVE_WITH_KNOTS('',3,(#14943,#14944,#14945,#14946,#14947,
#14948,#14949,#14950,#14951,#14952),.UNSPECIFIED.,.F.,.F.,(4,1,1,1,1,1,
1,4),(28.274333882308,28.8326458986048,29.8310963125047,30.8295467264045,
31.8279971403043,32.8264475542041,33.824897968104,34.5575191894876),
 .UNSPECIFIED.);
#1784=B_SPLINE_CURVE_WITH_KNOTS('',3,(#14953,#14954,#14955,#14956,#14957,
#14958,#14959,#14960,#14961,#14962,#14963),.UNSPECIFIED.,.F.,.F.,(4,1,1,
1,1,1,1,1,4),(28.274333882308,28.3767059215694,29.3751563354692,30.373606749369,
31.3720571632688,32.3705075771687,33.3689579910685,34.3674084049683,34.5575191894876),
 .UNSPECIFIED.);
#1785=B_SPLINE_CURVE_WITH_KNOTS('',3,(#14968,#14969,#14970,#14971,#14972,
#14973,#14974,#14975,#14976,#14977),.UNSPECIFIED.,.F.,.F.,(4,1,1,1,1,1,
1,4),(21.9911485751285,22.8419434152058,23.8403938291057,24.8388442430055,
25.8372946569053,26.8357450708052,27.834195484705,28.274333882308),
 .UNSPECIFIED.);
#1786=B_SPLINE_CURVE_WITH_KNOTS('',3,(#14978,#14979,#14980,#14981,#14982,
#14983,#14984,#14985,#14986,#14987),.UNSPECIFIED.,.F.,.F.,(4,1,1,1,1,1,
1,4),(21.9911485751284,22.3860034381704,23.3844538520702,24.38290426597,
25.3813546798699,26.3798050937697,27.3782555076695,28.274333882308),
 .UNSPECIFIED.);
#1787=B_SPLINE_CURVE_WITH_KNOTS('',3,(#14993,#14994,#14995,#14996,#14997),
 .UNSPECIFIED.,.F.,.F.,(4,1,4),(14.3984001269718,15.3968505408716,15.7079632679489),
 .UNSPECIFIED.);
#1788=B_SPLINE_CURVE_WITH_KNOTS('',3,(#15000,#15001,#15002,#15003,#15004),
 .UNSPECIFIED.,.F.,.F.,(4,1,4),(13.8759337553362,14.8543401040072,15.7079632679489),
 .UNSPECIFIED.);
#1789=B_SPLINE_CURVE_WITH_KNOTS('',3,(#15010,#15011,#15012,#15013),
 .UNSPECIFIED.,.F.,.F.,(4,4),(108.12371336303,108.831095115081),
 .UNSPECIFIED.);
#1790=B_SPLINE_CURVE_WITH_KNOTS('',3,(#15021,#15022,#15023,#15024,#15025,
#15026,#15027,#15028,#15029,#15030),.UNSPECIFIED.,.F.,.F.,(4,3,3,4),(-106.814150222053,
-105.835743873382,-104.837293459482,-104.379939320515),.UNSPECIFIED.);
#1791=B_SPLINE_CURVE_WITH_KNOTS('',3,(#15035,#15036,#15037,#15038,#15039,
#15040,#15041,#15042,#15043,#15044,#15045,#15046,#15047,#15048,#15049,#15050,
#15051,#15052,#15053,#15054,#15055,#15056),.UNSPECIFIED.,.F.,.F.,(4,3,3,
3,3,3,3,4),(101.84052805585,102.840392631682,103.838843045582,104.837293459482,
105.835743873382,106.834194287282,107.832644701182,108.12371336303),
 .UNSPECIFIED.);
#1792=B_SPLINE_CURVE_WITH_KNOTS('',3,(#15057,#15058,#15059,#15060,#15061,
#15062,#15063,#15064,#15065,#15066,#15067,#15068,#15069,#15070,#15071,#15072,
#15073,#15074,#15075,#15076,#15077,#15078),.UNSPECIFIED.,.F.,.F.,(4,3,3,
3,3,3,3,4),(-104.379939320515,-103.838843045582,-102.840392631682,-101.841942217783,
-100.843491803883,-99.8450413899829,-98.8465909760831,-98.096754013335),
 .UNSPECIFIED.);
#1793=B_SPLINE_CURVE_WITH_KNOTS('',3,(#15083,#15084,#15085,#15086,#15087,
#15088,#15089,#15090,#15091,#15092,#15093,#15094,#15095,#15096,#15097,#15098,
#15099,#15100,#15101,#15102,#15103,#15104),.UNSPECIFIED.,.F.,.F.,(4,3,3,
3,3,3,3,4),(95.5573427486709,95.8512397343836,96.8496901482834,97.8481405621833,
98.8465909760831,99.8450413899829,100.843491803883,101.84052805585),
 .UNSPECIFIED.);
#1794=B_SPLINE_CURVE_WITH_KNOTS('',3,(#15105,#15106,#15107,#15108,#15109,
#15110,#15111,#15112,#15113,#15114,#15115,#15116,#15117,#15118,#15119,#15120,
#15121,#15122,#15123,#15124,#15125,#15126,#15127,#15128,#15129),
 .UNSPECIFIED.,.F.,.F.,(4,3,3,3,3,3,3,3,4),(-98.096754013335,-97.8481405621833,
-96.8496901482835,-95.8512397343836,-94.8527893204838,-93.854338906584,
-92.8558884926841,-91.8574380787843,-91.8135687061554),.UNSPECIFIED.);
#1795=B_SPLINE_CURVE_WITH_KNOTS('',3,(#15134,#15135,#15136,#15137,#15138,
#15139,#15140,#15141,#15142,#15143,#15144,#15145,#15146,#15147,#15148,#15149,
#15150,#15151,#15152,#15153,#15154,#15155),.UNSPECIFIED.,.F.,.F.,(4,3,3,
3,3,3,3,4),(89.2741574414913,89.8605372509846,90.8589876648845,91.8574380787843,
92.8558884926841,93.854338906584,94.8527893204838,95.5573427486709),
 .UNSPECIFIED.);
#1796=B_SPLINE_CURVE_WITH_KNOTS('',3,(#15156,#15157,#15158,#15159,#15160,
#15161,#15162,#15163,#15164,#15165,#15166,#15167,#15168,#15169,#15170,#15171,
#15172,#15173,#15174,#15175,#15176,#15177),.UNSPECIFIED.,.F.,.F.,(4,3,3,
3,3,3,3,4),(-91.8135687061554,-90.8589876648845,-89.8605372509847,-88.8620868370848,
-87.863636423185,-86.8651860092852,-85.8667355953854,-85.5303833989758),
 .UNSPECIFIED.);
#1797=B_SPLINE_CURVE_WITH_KNOTS('',3,(#15182,#15183,#15184,#15185,#15186,
#15187,#15188,#15189,#15190,#15191,#15192,#15193,#15194,#15195,#15196,#15197,
#15198,#15199,#15200,#15201,#15202,#15203),.UNSPECIFIED.,.F.,.F.,(4,3,3,
3,3,3,3,4),(82.9909721343117,83.8698347675857,84.8682851814855,85.8667355953853,
86.8651860092852,87.863636423185,88.8620868370848,89.2741574414913),
 .UNSPECIFIED.);
#1798=B_SPLINE_CURVE_WITH_KNOTS('',3,(#15204,#15205,#15206,#15207,#15208,
#15209,#15210,#15211,#15212,#15213,#15214,#15215,#15216,#15217,#15218,#15219,
#15220,#15221,#15222,#15223,#15224,#15225),.UNSPECIFIED.,.F.,.F.,(4,3,3,
3,3,3,3,4),(-85.5303833989758,-84.8682851814855,-83.8698347675857,-82.8713843536859,
-81.872933939786,-80.8744835258862,-79.8760331119864,-79.2471980917962),
 .UNSPECIFIED.);
#1799=B_SPLINE_CURVE_WITH_KNOTS('',3,(#15230,#15231,#15232,#15233,#15234,
#15235,#15236,#15237,#15238,#15239,#15240,#15241,#15242,#15243,#15244,#15245,
#15246,#15247,#15248,#15249,#15250,#15251,#15252,#15253,#15254),
 .UNSPECIFIED.,.F.,.F.,(4,3,3,3,3,3,3,3,4),(76.7077868271321,76.8806818702868,
77.8791322841867,78.8775826980865,79.8760331119864,80.8744835258862,81.872933939786,
82.8713843536859,82.9909721343117),.UNSPECIFIED.);
#1800=B_SPLINE_CURVE_WITH_KNOTS('',3,(#15255,#15256,#15257,#15258,#15259,
#15260,#15261,#15262,#15263,#15264,#15265,#15266,#15267,#15268,#15269,#15270,
#15271,#15272,#15273,#15274,#15275,#15276),.UNSPECIFIED.,.F.,.F.,(4,3,3,
3,3,3,3,4),(-79.2471980917962,-78.8775826980865,-77.8791322841867,-76.8806818702869,
-75.882231456387,-74.8837810424872,-73.8853306285874,-72.9640127846166),
 .UNSPECIFIED.);
#1801=B_SPLINE_CURVE_WITH_KNOTS('',3,(#15281,#15282,#15283,#15284,#15285,
#15286,#15287,#15288,#15289,#15290,#15291,#15292,#15293,#15294,#15295,#15296,
#15297,#15298,#15299,#15300,#15301,#15302),.UNSPECIFIED.,.F.,.F.,(4,3,3,
3,3,3,3,4),(70.4246015199525,70.8899793868879,71.8884298007877,72.8868802146875,
73.8853306285874,74.8837810424872,75.882231456387,76.7077868271321),
 .UNSPECIFIED.);
#1802=B_SPLINE_CURVE_WITH_KNOTS('',3,(#15303,#15304,#15305,#15306,#15307,
#15308,#15309,#15310,#15311,#15312,#15313,#15314,#15315,#15316,#15317,#15318,
#15319,#15320,#15321,#15322,#15323,#15324,#15325,#15326,#15327),
 .UNSPECIFIED.,.F.,.F.,(4,3,3,3,3,3,3,3,4),(-72.9640127846166,-72.8868802146875,
-71.8884298007877,-70.8899793868879,-69.891528972988,-68.8930785590882,
-67.8946281451884,-66.8961777312886,-66.680827477437),.UNSPECIFIED.);
#1803=B_SPLINE_CURVE_WITH_KNOTS('',3,(#15332,#15333,#15334,#15335,#15336,
#15337,#15338,#15339,#15340,#15341,#15342,#15343,#15344,#15345,#15346,#15347,
#15348,#15349,#15350,#15351,#15352,#15353),.UNSPECIFIED.,.F.,.F.,(4,3,3,
3,3,3,3,4),(64.1414162127729,64.8992769034889,65.8977273173887,66.8961777312886,
67.8946281451884,68.8930785590882,69.8915289729881,70.4246015199525),
 .UNSPECIFIED.);
#1804=B_SPLINE_CURVE_WITH_KNOTS('',3,(#15354,#15355,#15356,#15357,#15358,
#15359,#15360,#15361,#15362,#15363,#15364,#15365,#15366,#15367,#15368,#15369,
#15370,#15371,#15372,#15373,#15374,#15375),.UNSPECIFIED.,.F.,.F.,(4,3,3,
3,3,3,3,4),(-66.680827477437,-65.8977273173887,-64.8992769034889,-63.9008264895891,
-62.9023760756892,-61.9039256617894,-60.9054752478896,-60.3976421702575),
 .UNSPECIFIED.);
#1805=B_SPLINE_CURVE_WITH_KNOTS('',3,(#15380,#15381,#15382,#15383,#15384,
#15385,#15386,#15387,#15388,#15389,#15390,#15391,#15392,#15393,#15394,#15395,
#15396,#15397,#15398,#15399,#15400,#15401,#15402,#15403,#15404),
 .UNSPECIFIED.,.F.,.F.,(4,3,3,3,3,3,3,3,4),(57.8582309055933,57.9101240061901,
58.9085744200899,59.9070248339898,60.9054752478896,61.9039256617894,62.9023760756892,
63.9008264895891,64.1414162127729),.UNSPECIFIED.);
#1806=B_SPLINE_CURVE_WITH_KNOTS('',3,(#15405,#15406,#15407,#15408,#15409,
#15410,#15411,#15412,#15413,#15414,#15415,#15416,#15417,#15418,#15419,#15420,
#15421,#15422,#15423,#15424,#15425,#15426),.UNSPECIFIED.,.F.,.F.,(4,3,3,
3,3,3,3,4),(-60.3976421702575,-59.9070248339898,-58.9085744200899,-57.9101240061901,
-56.9116735922903,-55.9132231783904,-54.9147727644906,-54.1144568630779),
 .UNSPECIFIED.);
#1807=B_SPLINE_CURVE_WITH_KNOTS('',3,(#15431,#15432,#15433,#15434,#15435,
#15436,#15437,#15438,#15439,#15440,#15441,#15442,#15443,#15444,#15445,#15446,
#15447,#15448,#15449,#15450,#15451,#15452),.UNSPECIFIED.,.F.,.F.,(4,3,3,
3,3,3,3,4),(51.5750455984137,51.9194215227911,52.917871936691,53.9163223505908,
54.9147727644906,55.9132231783904,56.9116735922903,57.8582309055933),
 .UNSPECIFIED.);
#1808=B_SPLINE_CURVE_WITH_KNOTS('',3,(#15453,#15454,#15455,#15456,#15457,
#15458,#15459,#15460,#15461,#15462,#15463,#15464,#15465,#15466,#15467,#15468,
#15469,#15470,#15471,#15472,#15473,#15474,#15475,#15476,#15477),
 .UNSPECIFIED.,.F.,.F.,(4,3,3,3,3,3,3,3,4),(-54.1144568630779,-53.9163223505908,
-52.917871936691,-51.9194215227911,-50.9209711088913,-49.9225206949915,
-48.9240702810916,-47.9256198671918,-47.8312715558983),.UNSPECIFIED.);
#1809=B_SPLINE_CURVE_WITH_KNOTS('',3,(#15482,#15483,#15484,#15485,#15486,
#15487,#15488,#15489,#15490,#15491,#15492,#15493,#15494,#15495,#15496,#15497,
#15498,#15499,#15500,#15501,#15502,#15503),.UNSPECIFIED.,.F.,.F.,(4,3,3,
3,3,3,3,4),(45.2918602912341,45.9287190393921,46.927169453292,47.9256198671918,
48.9240702810916,49.9225206949915,50.9209711088913,51.5750455984137),
 .UNSPECIFIED.);
#1810=B_SPLINE_CURVE_WITH_KNOTS('',3,(#15504,#15505,#15506,#15507,#15508,
#15509,#15510,#15511,#15512,#15513,#15514,#15515,#15516,#15517,#15518,#15519,
#15520,#15521,#15522,#15523,#15524,#15525),.UNSPECIFIED.,.F.,.F.,(4,3,3,
3,3,3,3,4),(-47.8312715558983,-46.927169453292,-45.9287190393921,-44.9302686254923,
-43.9318182115925,-42.9333677976927,-41.9349173837928,-41.5480862487187),
 .UNSPECIFIED.);
#1811=B_SPLINE_CURVE_WITH_KNOTS('',3,(#15530,#15531,#15532,#15533,#15534,
#15535,#15536,#15537,#15538,#15539,#15540,#15541,#15542,#15543,#15544,#15545,
#15546,#15547,#15548,#15549,#15550,#15551),.UNSPECIFIED.,.F.,.F.,(4,3,3,
3,3,3,3,4),(39.0086749840546,39.9380165559932,40.936466969893,41.9349173837928,
42.9333677976927,43.9318182115925,44.9302686254923,45.2918602912341),
 .UNSPECIFIED.);
#1812=B_SPLINE_CURVE_WITH_KNOTS('',3,(#15552,#15553,#15554,#15555,#15556,
#15557,#15558,#15559,#15560,#15561,#15562,#15563,#15564,#15565,#15566,#15567,
#15568,#15569,#15570,#15571,#15572,#15573),.UNSPECIFIED.,.F.,.F.,(4,3,3,
3,3,3,3,4),(-41.5480862487187,-40.936466969893,-39.9380165559932,-38.9395661420933,
-37.9411157281935,-36.9426653142937,-35.9442149003939,-35.2649009415391),
 .UNSPECIFIED.);
#1813=B_SPLINE_CURVE_WITH_KNOTS('',3,(#15578,#15579,#15580,#15581,#15582,
#15583,#15584,#15585,#15586,#15587,#15588,#15589,#15590,#15591,#15592,#15593,
#15594,#15595,#15596,#15597,#15598,#15599,#15600,#15601,#15602),
 .UNSPECIFIED.,.F.,.F.,(4,3,3,3,3,3,3,3,4),(32.725489676875,32.9488636586944,
33.9473140725942,34.945764486494,35.9442149003939,36.9426653142937,37.9411157281935,
38.9395661420933,39.0086749840546),.UNSPECIFIED.);
#1814=B_SPLINE_CURVE_WITH_KNOTS('',3,(#15603,#15604,#15605,#15606,#15607,
#15608,#15609,#15610,#15611,#15612,#15613,#15614,#15615,#15616,#15617,#15618,
#15619,#15620,#15621,#15622,#15623,#15624),.UNSPECIFIED.,.F.,.F.,(4,3,3,
3,3,3,3,4),(-35.2649009415391,-34.945764486494,-33.9473140725942,-32.9488636586944,
-31.9504132447945,-30.9519628308947,-29.9535124169949,-28.9817156343595),
 .UNSPECIFIED.);
#1815=B_SPLINE_CURVE_WITH_KNOTS('',3,(#15629,#15630,#15631,#15632,#15633,
#15634,#15635,#15636,#15637,#15638,#15639,#15640,#15641,#15642,#15643,#15644,
#15645,#15646,#15647,#15648,#15649,#15650),.UNSPECIFIED.,.F.,.F.,(4,3,3,
3,3,3,3,4),(26.4423043696954,26.9581611752954,27.9566115891952,28.955062003095,
29.9535124169949,30.9519628308947,31.9504132447945,32.725489676875),
 .UNSPECIFIED.);
#1816=B_SPLINE_CURVE_WITH_KNOTS('',3,(#15651,#15652,#15653,#15654,#15655,
#15656,#15657,#15658,#15659,#15660,#15661,#15662,#15663,#15664,#15665,#15666,
#15667,#15668,#15669,#15670,#15671,#15672,#15673,#15674,#15675),
 .UNSPECIFIED.,.F.,.F.,(4,3,3,3,3,3,3,3,4),(-28.9817156343595,-28.955062003095,
-27.9566115891952,-26.9581611752954,-25.9597107613956,-24.9612603474957,
-23.9628099335959,-22.9643595196961,-22.6985303271799),.UNSPECIFIED.);
#1817=B_SPLINE_CURVE_WITH_KNOTS('',3,(#15680,#15681,#15682,#15683,#15684,
#15685,#15686,#15687,#15688,#15689,#15690,#15691,#15692,#15693,#15694,#15695,
#15696,#15697,#15698,#15699,#15700,#15701),.UNSPECIFIED.,.F.,.F.,(4,3,3,
3,3,3,3,4),(20.1591190625158,20.9674586918964,21.9659091057962,22.9643595196961,
23.9628099335959,24.9612603474957,25.9597107613956,26.4423043696954),
 .UNSPECIFIED.);
#1818=B_SPLINE_CURVE_WITH_KNOTS('',3,(#15702,#15703,#15704,#15705,#15706,
#15707,#15708,#15709,#15710,#15711,#15712,#15713,#15714,#15715,#15716,#15717,
#15718,#15719,#15720,#15721,#15722,#15723),.UNSPECIFIED.,.F.,.F.,(4,3,3,
3,3,3,3,4),(-22.6985303271799,-21.9659091057962,-20.9674586918964,-19.9690082779966,
-18.9705578640968,-17.9721074501969,-16.9736570362971,-16.4153450200003),
 .UNSPECIFIED.);
#1819=B_SPLINE_CURVE_WITH_KNOTS('',3,(#15728,#15729,#15730,#15731,#15732,
#15733,#15734,#15735,#15736,#15737,#15738,#15739,#15740,#15741,#15742,#15743,
#15744,#15745,#15746,#15747,#15748,#15749,#15750,#15751,#15752),
 .UNSPECIFIED.,.F.,.F.,(4,3,3,3,3,3,3,3,4),(13.8759337553362,13.9783057945976,
14.9767562084974,15.9752066223973,16.9736570362971,17.9721074501969,18.9705578640968,
19.9690082779966,20.1591190625158),.UNSPECIFIED.);
#1820=B_SPLINE_CURVE_WITH_KNOTS('',3,(#15753,#15754,#15755,#15756,#15757,
#15758,#15759,#15760,#15761,#15762,#15763,#15764,#15765,#15766,#15767,#15768,
#15769,#15770,#15771,#15772,#15773,#15774),.UNSPECIFIED.,.F.,.F.,(4,3,3,
3,3,3,3,4),(-16.4153450200003,-15.9752066223973,-14.9767562084974,-13.9783057945976,
-12.9798553806978,-11.9814049667979,-10.9829545528981,-10.1321597128207),
 .UNSPECIFIED.);
#1821=B_SPLINE_CURVE_WITH_KNOTS('',3,(#15780,#15781,#15782,#15783,#15784,
#15785,#15786,#15787,#15788,#15789,#15790,#15791,#15792),.UNSPECIFIED.,
 .F.,.F.,(4,3,3,3,4),(-3.84897440564114,-2.99535124169948,-1.99690082779965,
-0.99845041389982,0.),.UNSPECIFIED.);
#1822=B_SPLINE_CURVE_WITH_KNOTS('',3,(#15795,#15796,#15797,#15798,#15799,
#15800,#15801,#15802,#15803,#15804,#15805,#15806,#15807,#15808,#15809,#15810,
#15811,#15812,#15813),.UNSPECIFIED.,.F.,.F.,(4,3,3,3,3,3,4),(2.01694489302848,
2.99535124169948,3.99380165559931,4.99225206949914,5.99070248339897,6.9891528972988,
7.59274844815661),.UNSPECIFIED.);
#1823=B_SPLINE_CURVE_WITH_KNOTS('',3,(#15819,#15820,#15821,#15822,#15823,
#15824,#15825,#15826),.UNSPECIFIED.,.F.,.F.,(4,1,1,1,1,4),(116.238928182822,
116.69628232179,117.69473273569,118.693183149589,119.691633563489,120.690083977389),
 .UNSPECIFIED.);
#1824=B_SPLINE_CURVE_WITH_KNOTS('',3,(#15829,#15830,#15831,#15832,#15833,
#15834,#15835,#15836,#15837),.UNSPECIFIED.,.F.,.F.,(4,1,1,1,1,1,4),(116.238928182822,
116.240342344754,117.238792758654,118.237243172554,119.235693586454,120.234144000354,
121.212550349025),.UNSPECIFIED.);
#1825=B_SPLINE_CURVE_WITH_KNOTS('',3,(#15842,#15843,#15844,#15845,#15846,
#15847,#15848,#15849,#15850,#15851),.UNSPECIFIED.,.F.,.F.,(4,1,1,1,1,1,
1,4),(109.955742875643,110.705579838391,111.704030252291,112.70248066619,
113.70093108009,114.69938149399,115.69783190789,116.238928182822),
 .UNSPECIFIED.);
#1826=B_SPLINE_CURVE_WITH_KNOTS('',3,(#15852,#15853,#15854,#15855,#15856,
#15857,#15858,#15859,#15860,#15861),.UNSPECIFIED.,.F.,.F.,(4,1,1,1,1,1,
1,4),(109.955742875643,110.249639861355,111.248090275255,112.246540689155,
113.244991103055,114.243441516955,115.241891930855,116.238928182822),
 .UNSPECIFIED.);
#1827=B_SPLINE_CURVE_WITH_KNOTS('',3,(#15866,#15867,#15868,#15869,#15870,
#15871,#15872,#15873,#15874,#15875,#15876),.UNSPECIFIED.,.F.,.F.,(4,1,1,
1,1,1,1,1,4),(103.672557568463,103.716426941092,104.714877354992,105.713327768892,
106.711778182792,107.710228596691,108.708679010591,109.707129424491,109.955742875643),
 .UNSPECIFIED.);
#1828=B_SPLINE_CURVE_WITH_KNOTS('',3,(#15877,#15878,#15879,#15880,#15881,
#15882,#15883,#15884,#15885,#15886),.UNSPECIFIED.,.F.,.F.,(4,1,1,1,1,1,
1,4),(103.672557568463,104.258937377956,105.257387791856,106.255838205756,
107.254288619656,108.252739033556,109.251189447456,109.955742875643),
 .UNSPECIFIED.);
#1829=B_SPLINE_CURVE_WITH_KNOTS('',3,(#15891,#15892,#15893,#15894,#15895,
#15896,#15897,#15898,#15899,#15900),.UNSPECIFIED.,.F.,.F.,(4,1,1,1,1,1,
1,4),(97.3893722612835,97.7257244576931,98.7241748715929,99.7226252854927,
100.721075699393,101.719526113292,102.717976527192,103.672557568463),
 .UNSPECIFIED.);
#1830=B_SPLINE_CURVE_WITH_KNOTS('',3,(#15901,#15902,#15903,#15904,#15905,
#15906,#15907,#15908,#15909,#15910),.UNSPECIFIED.,.F.,.F.,(4,1,1,1,1,1,
1,4),(97.3893722612835,98.2682348945574,99.2666853084573,100.265135722357,
101.263586136257,102.262036550157,103.260486964057,103.672557568463),
 .UNSPECIFIED.);
#1831=B_SPLINE_CURVE_WITH_KNOTS('',3,(#15915,#15916,#15917,#15918,#15919,
#15920,#15921,#15922,#15923,#15924),.UNSPECIFIED.,.F.,.F.,(4,1,1,1,1,1,
1,4),(91.106186954104,91.7350219742941,92.7334723881939,93.7319228020937,
94.7303732159936,95.7288236298934,96.7272740437932,97.3893722612835),
 .UNSPECIFIED.);
#1832=B_SPLINE_CURVE_WITH_KNOTS('',3,(#15925,#15926,#15927,#15928,#15929,
#15930,#15931,#15932,#15933,#15934,#15935),.UNSPECIFIED.,.F.,.F.,(4,1,1,
1,1,1,1,1,4),(91.106186954104,91.2790819972586,92.2775324111584,93.2759828250583,
94.2744332389581,95.2728836528579,96.2713340667578,97.2697844806576,97.3893722612835),
 .UNSPECIFIED.);
#1833=B_SPLINE_CURVE_WITH_KNOTS('',3,(#15940,#15941,#15942,#15943,#15944,
#15945,#15946,#15947,#15948,#15949),.UNSPECIFIED.,.F.,.F.,(4,1,1,1,1,1,
1,4),(84.8230016469244,85.7443194908951,86.7427699047949,87.7412203186948,
88.7396707325946,89.7381211464944,90.7365715603943,91.106186954104),
 .UNSPECIFIED.);
#1834=B_SPLINE_CURVE_WITH_KNOTS('',3,(#15950,#15951,#15952,#15953,#15954,
#15955,#15956,#15957,#15958,#15959),.UNSPECIFIED.,.F.,.F.,(4,1,1,1,1,1,
1,4),(84.8230016469244,85.2883795138596,86.2868299277595,87.2852803416593,
88.2837307555591,89.282181169459,90.2806315833588,91.106186954104),
 .UNSPECIFIED.);
#1835=B_SPLINE_CURVE_WITH_KNOTS('',3,(#15964,#15965,#15966,#15967,#15968,
#15969,#15970,#15971,#15972,#15973,#15974),.UNSPECIFIED.,.F.,.F.,(4,1,1,
1,1,1,1,1,4),(78.5398163397448,78.7551665935963,79.7536170074961,80.7520674213959,
81.7505178352958,82.7489682491956,83.7474186630954,84.7458690769953,84.8230016469244),
 .UNSPECIFIED.);
#1836=B_SPLINE_CURVE_WITH_KNOTS('',3,(#15975,#15976,#15977,#15978,#15979,
#15980,#15981,#15982,#15983,#15984),.UNSPECIFIED.,.F.,.F.,(4,1,1,1,1,1,
1,4),(78.5398163397448,79.2976770304607,80.2961274443605,81.2945778582603,
82.2930282721602,83.29147868606,84.2899290999598,84.8230016469244),
 .UNSPECIFIED.);
#1837=B_SPLINE_CURVE_WITH_KNOTS('',3,(#15989,#15990,#15991,#15992,#15993,
#15994,#15995,#15996,#15997,#15998),.UNSPECIFIED.,.F.,.F.,(4,1,1,1,1,1,
1,4),(72.2566310325652,72.7644641101973,73.7629145240972,74.761364937997,
75.7598153518968,76.7582657657966,77.7567161796965,78.5398163397448),
 .UNSPECIFIED.);
#1838=B_SPLINE_CURVE_WITH_KNOTS('',3,(#15999,#16000,#16001,#16002,#16003,
#16004,#16005,#16006,#16007,#16008,#16009),.UNSPECIFIED.,.F.,.F.,(4,1,1,
1,1,1,1,1,4),(72.2566310325652,72.3085241331619,73.3069745470617,74.3054249609615,
75.3038753748613,76.3023257887612,77.300776202661,78.2992266165608,78.5398163397448),
 .UNSPECIFIED.);
#1839=B_SPLINE_CURVE_WITH_KNOTS('',3,(#16014,#16015,#16016,#16017,#16018,
#16019,#16020,#16021,#16022,#16023),.UNSPECIFIED.,.F.,.F.,(4,1,1,1,1,1,
1,4),(65.9734457253856,66.7737616267983,67.7722120406982,68.770662454598,
69.7691128684978,70.7675632823977,71.7660136962975,72.2566310325652),
 .UNSPECIFIED.);
#1840=B_SPLINE_CURVE_WITH_KNOTS('',3,(#16024,#16025,#16026,#16027,#16028,
#16029,#16030,#16031,#16032,#16033),.UNSPECIFIED.,.F.,.F.,(4,1,1,1,1,1,
1,4),(65.9734457253856,66.3178216497629,67.3162720636627,68.3147224775625,
69.3131728914624,70.3116233053622,71.310073719262,72.2566310325652),
 .UNSPECIFIED.);
#1841=B_SPLINE_CURVE_WITH_KNOTS('',3,(#16038,#16039,#16040,#16041,#16042,
#16043,#16044,#16045,#16046,#16047,#16048),.UNSPECIFIED.,.F.,.F.,(4,1,1,
1,1,1,1,1,4),(59.690260418206,59.7846087294995,60.7830591433994,61.7815095572992,
62.779959971199,63.7784103850989,64.7768607989987,65.7753112128985,65.9734457253856),
 .UNSPECIFIED.);
#1842=B_SPLINE_CURVE_WITH_KNOTS('',3,(#16049,#16050,#16051,#16052,#16053,
#16054,#16055,#16056,#16057,#16058),.UNSPECIFIED.,.F.,.F.,(4,1,1,1,1,1,
1,4),(59.690260418206,60.3271191663639,61.3255695802637,62.3240199941636,
63.3224704080634,64.3209208219632,65.3193712358631,65.9734457253856),
 .UNSPECIFIED.);
#1843=B_SPLINE_CURVE_WITH_KNOTS('',3,(#16063,#16064,#16065,#16066,#16067,
#16068,#16069,#16070,#16071,#16072),.UNSPECIFIED.,.F.,.F.,(4,1,1,1,1,1,
1,4),(53.4070751110264,53.7939062461006,54.7923566600004,55.7908070739002,
56.7892574878001,57.7877079016999,58.7861583155997,59.690260418206),
 .UNSPECIFIED.);
#1844=B_SPLINE_CURVE_WITH_KNOTS('',3,(#16073,#16074,#16075,#16076,#16077,
#16078,#16079,#16080,#16081,#16082),.UNSPECIFIED.,.F.,.F.,(4,1,1,1,1,1,
1,4),(53.4070751110264,54.3364166829649,55.3348670968648,56.3333175107646,
57.3317679246644,58.3302183385643,59.3286687524641,59.690260418206),
 .UNSPECIFIED.);
#1845=B_SPLINE_CURVE_WITH_KNOTS('',3,(#16087,#16088,#16089,#16090,#16091,
#16092,#16093,#16094,#16095,#16096),.UNSPECIFIED.,.F.,.F.,(4,1,1,1,1,1,
1,4),(47.1238898038468,47.8032037627016,48.8016541766014,49.8001045905012,
50.7985550044011,51.7970054183009,52.7954558322007,53.4070751110264),
 .UNSPECIFIED.);
#1846=B_SPLINE_CURVE_WITH_KNOTS('',3,(#16097,#16098,#16099,#16100,#16101,
#16102,#16103,#16104,#16105,#16106,#16107),.UNSPECIFIED.,.F.,.F.,(4,1,1,
1,1,1,1,1,4),(47.1238898038468,47.3472637856661,48.345714199566,49.3441646134658,
50.3426150273656,51.3410654412654,52.3395158551653,53.3379662690651,53.4070751110264),
 .UNSPECIFIED.);
#1847=B_SPLINE_CURVE_WITH_KNOTS('',3,(#16112,#16113,#16114,#16115,#16116,
#16117,#16118,#16119,#16120,#16121),.UNSPECIFIED.,.F.,.F.,(4,1,1,1,1,1,
1,4),(40.8407044966672,41.8125012793026,42.8109516932024,43.8094021071023,
44.8078525210021,45.8063029349019,46.8047533488018,47.1238898038468),
 .UNSPECIFIED.);
#1848=B_SPLINE_CURVE_WITH_KNOTS('',3,(#16122,#16123,#16124,#16125,#16126,
#16127,#16128,#16129,#16130,#16131),.UNSPECIFIED.,.F.,.F.,(4,1,1,1,1,1,
1,4),(40.8407044966672,41.3565613022672,42.355011716167,43.3534621300668,
44.3519125439666,45.3503629578665,46.3488133717663,47.1238898038468),
 .UNSPECIFIED.);
#1849=B_SPLINE_CURVE_WITH_KNOTS('',3,(#16136,#16137,#16138,#16139,#16140,
#16141,#16142,#16143,#16144,#16145,#16146),.UNSPECIFIED.,.F.,.F.,(4,1,1,
1,1,1,1,1,4),(34.5575191894876,34.8233483820038,35.8217987959036,36.8202492098035,
37.8186996237033,38.8171500376031,39.8156004515029,40.8140508654028,40.8407044966672),
 .UNSPECIFIED.);
#1850=B_SPLINE_CURVE_WITH_KNOTS('',3,(#16147,#16148,#16149,#16150,#16151,
#16152,#16153,#16154,#16155,#16156),.UNSPECIFIED.,.F.,.F.,(4,1,1,1,1,1,
1,4),(34.5575191894876,35.3658588188682,36.364309232768,37.3627596466678,
38.3612100605677,39.3596604744675,40.3581108883673,40.8407044966672),
 .UNSPECIFIED.);
#1851=B_SPLINE_CURVE_WITH_KNOTS('',3,(#16161,#16162,#16163,#16164,#16165,
#16166,#16167,#16168,#16169,#16170),.UNSPECIFIED.,.F.,.F.,(4,1,1,1,1,1,
1,4),(28.274333882308,28.8326458986048,29.8310963125046,30.8295467264045,
31.8279971403043,32.8264475542041,33.824897968104,34.5575191894876),
 .UNSPECIFIED.);
#1852=B_SPLINE_CURVE_WITH_KNOTS('',3,(#16171,#16172,#16173,#16174,#16175,
#16176,#16177,#16178,#16179,#16180,#16181),.UNSPECIFIED.,.F.,.F.,(4,1,1,
1,1,1,1,1,4),(28.274333882308,28.3767059215694,29.3751563354692,30.373606749369,
31.3720571632689,32.3705075771687,33.3689579910685,34.3674084049683,34.5575191894876),
 .UNSPECIFIED.);
#1853=B_SPLINE_CURVE_WITH_KNOTS('',3,(#16186,#16187,#16188,#16189,#16190,
#16191,#16192,#16193,#16194,#16195),.UNSPECIFIED.,.F.,.F.,(4,1,1,1,1,1,
1,4),(21.9911485751285,22.8419434152058,23.8403938291057,24.8388442430055,
25.8372946569053,26.8357450708052,27.834195484705,28.274333882308),
 .UNSPECIFIED.);
#1854=B_SPLINE_CURVE_WITH_KNOTS('',3,(#16196,#16197,#16198,#16199,#16200,
#16201,#16202,#16203,#16204,#16205),.UNSPECIFIED.,.F.,.F.,(4,1,1,1,1,1,
1,4),(21.9911485751284,22.3860034381704,23.3844538520702,24.3829042659701,
25.3813546798699,26.3798050937697,27.3782555076695,28.274333882308),
 .UNSPECIFIED.);
#1855=B_SPLINE_CURVE_WITH_KNOTS('',3,(#16211,#16212,#16213,#16214,#16215),
 .UNSPECIFIED.,.F.,.F.,(4,1,4),(14.3984001269718,15.3968505408716,15.7079632679489),
 .UNSPECIFIED.);
#1856=B_SPLINE_CURVE_WITH_KNOTS('',3,(#16218,#16219,#16220,#16221,#16222),
 .UNSPECIFIED.,.F.,.F.,(4,1,4),(13.8759337553362,14.8543401040072,15.7079632679489),
 .UNSPECIFIED.);
#1857=B_SPLINE_CURVE_WITH_KNOTS('',3,(#16224,#16225,#16226,#16227,#16228,
#16229,#16230,#16231,#16232,#16233,#16234,#16235,#16236,#16237,#16238,#16239,
#16240,#16241,#16242,#16243,#16244,#16245,#16246,#16247,#16248,#16249,#16250,
#16251,#16252,#16253,#16254,#16255,#16256,#16257,#16258,#16259,#16260,#16261,
#16262,#16263,#16264,#16265,#16266,#16267,#16268,#16269,#16270,#16271,#16272,
#16273,#16274,#16275,#16276,#16277,#16278,#16279,#16280,#16281,#16282,#16283,
#16284,#16285,#16286,#16287,#16288,#16289,#16290,#16291,#16292,#16293,#16294,
#16295,#16296,#16297,#16298,#16299,#16300,#16301,#16302,#16303,#16304,#16305,
#16306,#16307,#16308,#16309,#16310,#16311,#16312,#16313,#16314),
 .UNSPECIFIED.,.F.,.F.,(4,3,3,3,3,3,3,3,3,3,3,3,3,3,3,3,3,3,3,3,3,3,3,3,
3,3,3,3,3,3,4),(-0.569248610399407,-0.543578596463163,-0.517279330488097,
-0.510427274183678,-0.504800560895351,-0.477739172209543,-0.455689330734177,
-0.448366213390789,-0.442461660719966,-0.41472996294248,-0.386382582308514,
-0.358441367058857,-0.343970572338644,-0.337413249439412,-0.308477582949163,
-0.301340440406615,-0.273499497437324,-0.245035895034271,-0.233720105006401,
-0.228077781576704,-0.199099310593537,-0.169543243081912,-0.139741771809077,
-0.123046919548663,-0.118260996555259,-0.114011653396177,-0.08346298006925,
-0.0528795458366397,-0.0229338899610989,-0.00618295372576638,0.),
 .UNSPECIFIED.);
#1858=B_SPLINE_CURVE_WITH_KNOTS('',3,(#16315,#16316,#16317,#16318,#16319,
#16320,#16321,#16322,#16323,#16324,#16325,#16326,#16327,#16328,#16329,#16330,
#16331,#16332,#16333,#16334,#16335,#16336,#16337,#16338,#16339,#16340,#16341,
#16342,#16343,#16344,#16345,#16346,#16347,#16348,#16349,#16350,#16351,#16352,
#16353,#16354,#16355,#16356,#16357,#16358,#16359,#16360,#16361,#16362,#16363,
#16364,#16365,#16366,#16367,#16368,#16369,#16370,#16371,#16372,#16373,#16374,
#16375,#16376,#16377,#16378,#16379,#16380,#16381,#16382,#16383,#16384,#16385,
#16386,#16387,#16388,#16389,#16390,#16391,#16392,#16393,#16394,#16395,#16396,
#16397,#16398,#16399,#16400,#16401,#16402,#16403,#16404,#16405),
 .UNSPECIFIED.,.F.,.F.,(4,3,3,3,3,3,3,3,3,3,3,3,3,3,3,3,3,3,3,3,3,3,3,3,
3,3,3,3,3,3,4),(-0.566847306048068,-0.536667790777227,-0.506059605580284,
-0.497462088050579,-0.490486593578347,-0.460335737779737,-0.436884523306703,
-0.424130100459425,-0.418922747352239,-0.389496677338306,-0.360304013502597,
-0.332014662955751,-0.317192502715681,-0.312071570778799,-0.307326824244741,
-0.279357757008042,-0.27272602199547,-0.244230768419255,-0.21433741748379,
-0.205052770738313,-0.200811095462912,-0.172975232517528,-0.145198207857396,
-0.117889770880004,-0.103789044636945,-0.0993778831760535,-0.0726518756869364,
-0.0463552868969829,-0.0209007422778119,-0.00508396093552814,0.),
 .UNSPECIFIED.);
#1859=B_SPLINE_CURVE_WITH_KNOTS('',3,(#16407,#16408,#16409,#16410,#16411,
#16412,#16413,#16414,#16415,#16416,#16417),.UNSPECIFIED.,.F.,.F.,(4,1,1,
1,1,1,1,1,4),(15.7079632679489,15.852790517907,16.8512409318069,17.8496913457067,
18.8481417596065,19.8465921735064,20.8450425874062,21.843493001306,21.9911485751285),
 .UNSPECIFIED.);
#1860=B_SPLINE_CURVE_WITH_KNOTS('',3,(#16418,#16419,#16420,#16421,#16422,
#16423,#16424,#16425,#16426,#16427),.UNSPECIFIED.,.F.,.F.,(4,1,1,1,1,1,
1,4),(15.7079632679489,16.3953009547714,17.3937513686712,18.3922017825711,
19.3906521964709,20.3891026103707,21.3875530242706,21.9911485751284),
 .UNSPECIFIED.);
#1861=B_SPLINE_CURVE_WITH_KNOTS('',3,(#16876,#16877,#16878,#16879,#16880,
#16881,#16882,#16883,#16884,#16885,#16886,#16887,#16888,#16889,#16890,#16891,
#16892,#16893,#16894,#16895,#16896,#16897,#16898,#16899,#16900,#16901,#16902,
#16903,#16904,#16905,#16906,#16907,#16908,#16909,#16910,#16911,#16912,#16913,
#16914,#16915,#16916,#16917,#16918,#16919,#16920,#16921,#16922,#16923,#16924,
#16925,#16926,#16927,#16928,#16929,#16930,#16931,#16932,#16933,#16934,#16935,
#16936,#16937,#16938,#16939,#16940,#16941,#16942,#16943,#16944,#16945,#16946,
#16947,#16948,#16949,#16950,#16951,#16952,#16953,#16954,#16955,#16956,#16957,
#16958,#16959,#16960,#16961,#16962,#16963,#16964,#16965,#16966,#16967,#16968,
#16969,#16970,#16971,#16972),.UNSPECIFIED.,.F.,.F.,(4,3,3,3,3,3,3,3,3,3,
3,3,3,3,3,3,3,3,3,3,3,3,3,3,3,3,3,3,3,3,3,3,4),(0.,0.0253589562758107,0.0513899835108827,
0.0783515483041457,0.0901472329011983,0.0965516813294443,0.102699177545927,
0.130000868916647,0.157755246288974,0.185087060180977,0.195806070593553,
0.20210936686077,0.206420439750695,0.235022976376574,0.26352929739743,0.267082501856987,
0.294994868256452,0.306190141773776,0.311401074814444,0.315730762045215,
0.3438256131073,0.372960412553192,0.402414247073163,0.414012338023885,0.420579327404534,
0.426866604939584,0.456917898655282,0.482860587387028,0.492968514404809,
0.498516388426713,0.52960252100449,0.560688653582267,0.566847306048208),
 .UNSPECIFIED.);
#1862=B_SPLINE_CURVE_WITH_KNOTS('',3,(#16973,#16974,#16975,#16976,#16977,
#16978,#16979,#16980,#16981,#16982,#16983,#16984,#16985,#16986,#16987,#16988,
#16989,#16990,#16991,#16992,#16993,#16994,#16995,#16996,#16997),
 .UNSPECIFIED.,.F.,.F.,(4,3,3,3,3,3,3,3,4),(-10.1321597128207,-9.98450413899829,
-8.98605372509846,-7.98760331119862,-6.9891528972988,-5.99070248339897,
-4.99225206949914,-3.99380165559931,-3.84897440564114),.UNSPECIFIED.);
#1863=B_SPLINE_CURVE_WITH_KNOTS('',3,(#17446,#17447,#17448,#17449,#17450,
#17451,#17452,#17453,#17454,#17455,#17456,#17457,#17458,#17459,#17460,#17461,
#17462,#17463,#17464,#17465,#17466,#17467),.UNSPECIFIED.,.F.,.F.,(4,3,3,
3,3,3,3,4),(7.59274844815661,7.98760331119863,8.98605372509846,9.98450413899829,
10.9829545528981,11.981404966798,12.9798553806978,13.8759337553362),
 .UNSPECIFIED.);
#1864=B_SPLINE_CURVE_WITH_KNOTS('',3,(#17468,#17469,#17470,#17471,#17472,
#17473,#17474,#17475,#17476,#17477,#17478,#17479,#17480,#17481,#17482,#17483,
#17484,#17485,#17486,#17487,#17488,#17489,#17490,#17491,#17492,#17493,#17494,
#17495,#17496,#17497,#17498,#17499,#17500,#17501,#17502,#17503,#17504,#17505,
#17506,#17507,#17508,#17509,#17510,#17511,#17512,#17513,#17514,#17515,#17516,
#17517,#17518,#17519,#17520,#17521,#17522,#17523,#17524,#17525,#17526,#17527,
#17528,#17529,#17530,#17531,#17532,#17533,#17534,#17535,#17536,#17537,#17538,
#17539,#17540,#17541,#17542,#17543,#17544,#17545,#17546,#17547,#17548,#17549,
#17550,#17551,#17552,#17553,#17554,#17555,#17556,#17557,#17558,#17559,#17560,
#17561),.UNSPECIFIED.,.F.,.F.,(4,3,3,3,3,3,3,3,3,3,3,3,3,3,3,3,3,3,3,3,
3,3,3,3,3,3,3,3,3,3,3,4),(0.,0.0297203831394795,0.0601035467162832,0.0895497219052599,
0.115315125195615,0.120671839320256,0.150435254338286,0.180035115203003,
0.208944573459276,0.221427488552219,0.230458159732982,0.23471220724889,
0.263249756710517,0.291154363988279,0.295672948228097,0.324625445746226,
0.334643738865253,0.339478705934468,0.343237386322571,0.371326757387601,
0.39947478984986,0.427227777476084,0.438024540249258,0.443793094729609,
0.448942971696371,0.476234898938785,0.49821292729788,0.507328693746962,
0.512107928640037,0.538127470507601,0.564147012375166,0.569248610399473),
 .UNSPECIFIED.);
#1865=B_SPLINE_CURVE_WITH_KNOTS('',3,(#17564,#17565,#17566,#17567,#17568,
#17569,#17570,#17571,#17572,#17573,#17574,#17575,#17576,#17577,#17578,#17579,
#17580,#17581,#17582,#17583,#17584,#17585,#17586,#17587,#17588,#17589,#17590,
#17591,#17592,#17593,#17594,#17595,#17596,#17597,#17598,#17599,#17600,#17601,
#17602,#17603,#17604,#17605,#17606,#17607,#17608,#17609,#17610,#17611,#17612,
#17613,#17614,#17615,#17616,#17617,#17618,#17619,#17620,#17621,#17622,#17623,
#17624,#17625,#17626,#17627,#17628,#17629,#17630,#17631,#17632,#17633,#17634,
#17635,#17636,#17637,#17638,#17639,#17640,#17641,#17642,#17643,#17644,#17645,
#17646,#17647,#17648,#17649,#17650,#17651,#17652,#17653,#17654),
 .UNSPECIFIED.,.F.,.F.,(4,3,3,3,3,3,3,3,3,3,3,3,3,3,3,3,3,3,3,3,3,3,3,3,
3,3,3,3,3,3,4),(-0.569248610399443,-0.543578588652014,-0.517279316104031,
-0.510427238217388,-0.504800560499363,-0.477739166329021,-0.45568932558873,
-0.448366156831823,-0.442461645413569,-0.41472994217853,-0.386382566735571,
-0.358441354206424,-0.343970553035952,-0.337413258055178,-0.308477591793723,
-0.301340440406694,-0.273499502259986,-0.245035902856791,-0.233720101852398,
-0.228077781614374,-0.199099314524288,-0.169543248975156,-0.139741777996353,
-0.123046924962531,-0.11826102155782,-0.11401170878925,-0.083463036592537,
-0.0528796019523826,-0.0229339459431555,-0.0061829537257795,0.),
 .UNSPECIFIED.);
#1866=B_SPLINE_CURVE_WITH_KNOTS('',3,(#17655,#17656,#17657,#17658,#17659,
#17660,#17661,#17662,#17663,#17664,#17665,#17666,#17667,#17668,#17669,#17670,
#17671,#17672,#17673,#17674,#17675,#17676,#17677,#17678,#17679,#17680,#17681,
#17682,#17683,#17684,#17685,#17686,#17687,#17688,#17689,#17690,#17691,#17692,
#17693,#17694,#17695,#17696,#17697,#17698,#17699,#17700,#17701,#17702,#17703,
#17704,#17705,#17706,#17707,#17708,#17709,#17710,#17711,#17712,#17713,#17714,
#17715,#17716,#17717,#17718,#17719,#17720,#17721,#17722,#17723,#17724,#17725,
#17726,#17727,#17728,#17729,#17730,#17731,#17732,#17733,#17734,#17735,#17736,
#17737,#17738,#17739,#17740,#17741,#17742,#17743,#17744,#17745),
 .UNSPECIFIED.,.F.,.F.,(4,3,3,3,3,3,3,3,3,3,3,3,3,3,3,3,3,3,3,3,3,3,3,3,
3,3,3,3,3,3,4),(-0.566847306048142,-0.536667785913132,-0.50605959936329,
-0.497462080219576,-0.490486592168179,-0.460335736468636,-0.436884522159495,
-0.424130097594776,-0.418922746580067,-0.38949667718092,-0.360304013384567,
-0.332014664357047,-0.317192503766662,-0.312071575644096,-0.307326824831242,
-0.279357759469794,-0.272726021995507,-0.244230768475208,-0.214337417532747,
-0.20505277122677,-0.200811095853765,-0.172975232543609,-0.145198207986257,
-0.117889772593011,-0.103789046135826,-0.0993778841074578,-0.0726518774649773,
-0.0463552908642349,-0.020900750299918,-0.00508396093552477,0.),
 .UNSPECIFIED.);
#1867=B_SPLINE_CURVE_WITH_KNOTS('',3,(#17747,#17748,#17749,#17750,#17751,
#17752,#17753,#17754,#17755,#17756,#17757),.UNSPECIFIED.,.F.,.F.,(4,1,1,
1,1,1,1,1,4),(15.7079632679489,15.852790517907,16.8512409318069,17.8496913457067,
18.8481417596065,19.8465921735064,20.8450425874062,21.843493001306,21.9911485751285),
 .UNSPECIFIED.);
#1868=B_SPLINE_CURVE_WITH_KNOTS('',3,(#17758,#17759,#17760,#17761,#17762,
#17763,#17764,#17765,#17766,#17767),.UNSPECIFIED.,.F.,.F.,(4,1,1,1,1,1,
1,4),(15.7079632679489,16.3953009547714,17.3937513686712,18.3922017825711,
19.3906521964709,20.3891026103707,21.3875530242706,21.9911485751284),
 .UNSPECIFIED.);
#1869=B_SPLINE_CURVE_WITH_KNOTS('',3,(#18216,#18217,#18218,#18219,#18220,
#18221,#18222,#18223,#18224,#18225,#18226,#18227,#18228,#18229,#18230,#18231,
#18232,#18233,#18234,#18235,#18236,#18237,#18238,#18239,#18240,#18241,#18242,
#18243,#18244,#18245,#18246,#18247,#18248,#18249,#18250,#18251,#18252,#18253,
#18254,#18255,#18256,#18257,#18258,#18259,#18260,#18261,#18262,#18263,#18264,
#18265,#18266,#18267,#18268,#18269,#18270,#18271,#18272,#18273,#18274,#18275,
#18276,#18277,#18278,#18279,#18280,#18281,#18282,#18283,#18284,#18285,#18286,
#18287,#18288,#18289,#18290,#18291,#18292,#18293,#18294,#18295,#18296,#18297,
#18298,#18299,#18300,#18301,#18302,#18303,#18304,#18305,#18306,#18307,#18308,
#18309,#18310,#18311,#18312),.UNSPECIFIED.,.F.,.F.,(4,3,3,3,3,3,3,3,3,3,
3,3,3,3,3,3,3,3,3,3,3,3,3,3,3,3,3,3,3,3,3,3,4),(0.,0.0253589640191775,0.0513899982793661,
0.0783515612265618,0.0901472450159599,0.0965516873007117,0.102699175683727,
0.130000872479608,0.157755252595204,0.185087064910636,0.195806071974665,
0.202109368589621,0.206420440483056,0.235022978557914,0.263529297383441,
0.267082501856932,0.294994864743443,0.306190136087185,0.311401050641315,
0.315730756609606,0.343825602488203,0.372960399516403,0.402414233419896,
0.414012310566607,0.42057914219519,0.426866594758845,0.456917887218389,
0.48286057880933,0.492968489082692,0.498516363071224,0.529602508326689,
0.560688653582154,0.566847306048091),.UNSPECIFIED.);
#1870=B_SPLINE_CURVE_WITH_KNOTS('',3,(#18313,#18314,#18315,#18316,#18317,
#18318,#18319,#18320,#18321,#18322,#18323,#18324,#18325,#18326,#18327,#18328,
#18329,#18330,#18331,#18332,#18333,#18334,#18335,#18336,#18337),
 .UNSPECIFIED.,.F.,.F.,(4,3,3,3,3,3,3,3,4),(-10.1321597128207,-9.98450413899829,
-8.98605372509846,-7.98760331119863,-6.9891528972988,-5.99070248339897,
-4.99225206949914,-3.99380165559932,-3.84897440564114),.UNSPECIFIED.);
#1871=B_SPLINE_CURVE_WITH_KNOTS('',3,(#18786,#18787,#18788,#18789,#18790,
#18791,#18792,#18793,#18794,#18795,#18796,#18797,#18798,#18799,#18800,#18801,
#18802,#18803,#18804,#18805,#18806,#18807),.UNSPECIFIED.,.F.,.F.,(4,3,3,
3,3,3,3,4),(7.59274844815663,7.98760331119864,8.98605372509847,9.9845041389983,
10.9829545528981,11.981404966798,12.9798553806978,13.8759337553362),
 .UNSPECIFIED.);
#1872=B_SPLINE_CURVE_WITH_KNOTS('',3,(#18808,#18809,#18810,#18811,#18812,
#18813,#18814,#18815,#18816,#18817,#18818,#18819,#18820,#18821,#18822,#18823,
#18824,#18825,#18826,#18827,#18828,#18829,#18830,#18831,#18832,#18833,#18834,
#18835,#18836,#18837,#18838,#18839,#18840,#18841,#18842,#18843,#18844,#18845,
#18846,#18847,#18848,#18849,#18850,#18851,#18852,#18853,#18854,#18855,#18856,
#18857,#18858,#18859,#18860,#18861,#18862,#18863,#18864,#18865,#18866,#18867,
#18868,#18869,#18870,#18871,#18872,#18873,#18874,#18875,#18876,#18877,#18878,
#18879,#18880,#18881,#18882,#18883,#18884,#18885,#18886,#18887,#18888,#18889,
#18890,#18891,#18892,#18893,#18894,#18895,#18896,#18897,#18898,#18899,#18900,
#18901),.UNSPECIFIED.,.F.,.F.,(4,3,3,3,3,3,3,3,3,3,3,3,3,3,3,3,3,3,3,3,
3,3,3,3,3,3,3,3,3,3,3,4),(0.,0.0297203899945205,0.06010355702558,0.0895497309258828,
0.115315133088648,0.120671841145989,0.150435256327594,0.180035115425351,
0.208944573626014,0.221427487940053,0.230458155185264,0.234712201077947,
0.263249748593671,0.291154354340093,0.295672948228002,0.324625446145178,
0.334643737982065,0.339478702992735,0.343237383195306,0.371326754477909,
0.399474787132745,0.427227773598525,0.438024531377961,0.443793087224999,
0.448942972295281,0.476234898815801,0.498212927205595,0.507328692507987,
0.512107925785297,0.538127469080138,0.564147012374979,0.569248610399289),
 .UNSPECIFIED.);
#1873=B_SPLINE_CURVE_WITH_KNOTS('',3,(#18904,#18905,#18906,#18907,#18908,
#18909,#18910,#18911,#18912,#18913,#18914,#18915,#18916,#18917,#18918,#18919,
#18920,#18921,#18922,#18923,#18924,#18925,#18926,#18927,#18928,#18929,#18930,
#18931,#18932,#18933,#18934,#18935,#18936,#18937,#18938,#18939,#18940,#18941,
#18942,#18943,#18944,#18945,#18946,#18947,#18948,#18949,#18950,#18951,#18952,
#18953,#18954,#18955,#18956,#18957,#18958,#18959,#18960,#18961,#18962,#18963,
#18964,#18965,#18966,#18967,#18968,#18969,#18970,#18971,#18972,#18973,#18974,
#18975,#18976,#18977,#18978,#18979,#18980,#18981,#18982,#18983,#18984,#18985,
#18986,#18987,#18988,#18989,#18990,#18991,#18992,#18993,#18994),
 .UNSPECIFIED.,.F.,.F.,(4,3,3,3,3,3,3,3,3,3,3,3,3,3,3,3,3,3,3,3,3,3,3,3,
3,3,3,3,3,3,4),(-0.569248610399526,-0.543579431798118,-0.517280869422508,
-0.510431120482963,-0.504800591464605,-0.47773979012753,-0.455689871412427,
-0.448372136428178,-0.442463258694081,-0.414732144324734,-0.386384218345228,
-0.358442715127014,-0.3439725980329,-0.337412355992177,-0.308476667534375,
-0.301340440406708,-0.27349898470449,-0.24503506229541,-0.23372044216372,
-0.228077783746287,-0.199098898462337,-0.169542621789931,-0.139741118996361,
-0.123046348337536,-0.118258352302259,-0.114005782325404,-0.0834569890725602,
-0.0528735983342899,-0.0229279578859285,-0.00618295372576183,0.),
 .UNSPECIFIED.);
#1874=B_SPLINE_CURVE_WITH_KNOTS('',3,(#18995,#18996,#18997,#18998,#18999,
#19000,#19001,#19002,#19003,#19004,#19005,#19006,#19007,#19008,#19009,#19010,
#19011,#19012,#19013,#19014,#19015,#19016,#19017,#19018,#19019,#19020,#19021,
#19022,#19023,#19024,#19025,#19026,#19027,#19028,#19029,#19030,#19031,#19032,
#19033,#19034,#19035,#19036,#19037,#19038,#19039,#19040,#19041,#19042,#19043,
#19044,#19045,#19046,#19047,#19048,#19049,#19050,#19051,#19052,#19053,#19054,
#19055,#19056,#19057,#19058,#19059,#19060,#19061,#19062,#19063,#19064,#19065,
#19066,#19067,#19068,#19069,#19070,#19071,#19072,#19073,#19074,#19075,#19076,
#19077,#19078,#19079,#19080,#19081,#19082,#19083,#19084,#19085),
 .UNSPECIFIED.,.F.,.F.,(4,3,3,3,3,3,3,3,3,3,3,3,3,3,3,3,3,3,3,3,3,3,3,3,
3,3,3,3,3,3,4),(-0.566847306048112,-0.536668339194763,-0.506060306609139,
-0.497462971008878,-0.49048674636921,-0.460335880394182,-0.43688464809434,
-0.424130415052306,-0.418922833332638,-0.389496695041096,-0.360304026779685,
-0.332014506642465,-0.317192385480711,-0.312071032018094,-0.307326760176989,
-0.279357483073735,-0.27272602199545,-0.244230762652898,-0.214337412438226,
-0.205052717620921,-0.200811046971631,-0.172975225592022,-0.145198191377983,
-0.117889578720224,-0.103788876497136,-0.0993777838422393,-0.0726516837817966,
-0.0463548526568899,-0.0208998570126172,-0.00508396093552129,0.),
 .UNSPECIFIED.);
#1875=B_SPLINE_CURVE_WITH_KNOTS('',3,(#19087,#19088,#19089,#19090,#19091,
#19092,#19093,#19094,#19095,#19096,#19097),.UNSPECIFIED.,.F.,.F.,(4,1,1,
1,1,1,1,1,4),(15.7079632679489,15.852790517907,16.8512409318069,17.8496913457067,
18.8481417596065,19.8465921735064,20.8450425874062,21.843493001306,21.9911485751285),
 .UNSPECIFIED.);
#1876=B_SPLINE_CURVE_WITH_KNOTS('',3,(#19098,#19099,#19100,#19101,#19102,
#19103,#19104,#19105,#19106,#19107),.UNSPECIFIED.,.F.,.F.,(4,1,1,1,1,1,
1,4),(15.7079632679489,16.3953009547714,17.3937513686712,18.3922017825711,
19.3906521964709,20.3891026103707,21.3875530242705,21.9911485751285),
 .UNSPECIFIED.);
#1877=B_SPLINE_CURVE_WITH_KNOTS('',3,(#19556,#19557,#19558,#19559,#19560,
#19561,#19562,#19563,#19564,#19565,#19566,#19567,#19568,#19569,#19570,#19571,
#19572,#19573,#19574,#19575,#19576,#19577,#19578,#19579,#19580,#19581,#19582,
#19583,#19584,#19585,#19586,#19587,#19588,#19589,#19590,#19591,#19592,#19593,
#19594,#19595,#19596,#19597,#19598,#19599,#19600,#19601,#19602,#19603,#19604,
#19605,#19606,#19607,#19608,#19609,#19610,#19611,#19612,#19613,#19614,#19615,
#19616,#19617,#19618,#19619,#19620,#19621,#19622,#19623,#19624,#19625,#19626,
#19627,#19628,#19629,#19630,#19631,#19632,#19633,#19634,#19635,#19636,#19637,
#19638,#19639,#19640,#19641,#19642,#19643,#19644,#19645,#19646,#19647,#19648,
#19649,#19650,#19651,#19652),.UNSPECIFIED.,.F.,.F.,(4,3,3,3,3,3,3,3,3,3,
3,3,3,3,3,3,3,3,3,3,3,3,3,3,3,3,3,3,3,3,3,3,4),(0.,0.0253580839119621,0.0513883193661946,
0.0783500921775368,0.0901458677824991,0.0965510091518119,0.102699386274646,
0.130000465662217,0.157754532601719,0.185086524915523,0.19580591419694,
0.202109170553707,0.206420354259938,0.235022725853245,0.263529291896674,
0.267082501856933,0.294995261838824,0.306190778774865,0.311403784621555,
0.315731371826393,0.34382680331232,0.372961873868641,0.402415777646638,
0.414015416572459,0.420600208736835,0.426867850729504,0.456919286765161,
0.482861628469424,0.4929715795806,0.498519461182564,0.52960405738239,0.560688653582215,
0.566847306048152),.UNSPECIFIED.);
#1878=B_SPLINE_CURVE_WITH_KNOTS('',3,(#19653,#19654,#19655,#19656,#19657,
#19658,#19659,#19660,#19661,#19662,#19663,#19664,#19665,#19666,#19667,#19668,
#19669,#19670,#19671,#19672,#19673,#19674,#19675,#19676,#19677),
 .UNSPECIFIED.,.F.,.F.,(4,3,3,3,3,3,3,3,4),(-10.1321597128207,-9.98450413899828,
-8.98605372509846,-7.98760331119863,-6.9891528972988,-5.99070248339897,
-4.99225206949914,-3.99380165559931,-3.84897440564112),.UNSPECIFIED.);
#1879=B_SPLINE_CURVE_WITH_KNOTS('',3,(#20126,#20127,#20128,#20129,#20130,
#20131,#20132,#20133,#20134,#20135,#20136,#20137,#20138,#20139,#20140,#20141,
#20142,#20143,#20144,#20145,#20146,#20147),.UNSPECIFIED.,.F.,.F.,(4,3,3,
3,3,3,3,4),(7.59274844815663,7.98760331119864,8.98605372509847,9.9845041389983,
10.9829545528981,11.981404966798,12.9798553806978,13.8759337553362),
 .UNSPECIFIED.);
#1880=B_SPLINE_CURVE_WITH_KNOTS('',3,(#20148,#20149,#20150,#20151,#20152,
#20153,#20154,#20155,#20156,#20157,#20158,#20159,#20160,#20161,#20162,#20163,
#20164,#20165,#20166,#20167,#20168,#20169,#20170,#20171,#20172,#20173,#20174,
#20175,#20176,#20177,#20178,#20179,#20180,#20181,#20182,#20183,#20184,#20185,
#20186,#20187,#20188,#20189,#20190,#20191,#20192,#20193,#20194,#20195,#20196,
#20197,#20198,#20199,#20200,#20201,#20202,#20203,#20204,#20205,#20206,#20207,
#20208,#20209,#20210,#20211,#20212,#20213,#20214,#20215,#20216,#20217,#20218,
#20219,#20220,#20221,#20222,#20223,#20224,#20225,#20226,#20227,#20228,#20229,
#20230,#20231,#20232,#20233,#20234,#20235,#20236,#20237,#20238,#20239,#20240,
#20241),.UNSPECIFIED.,.F.,.F.,(4,3,3,3,3,3,3,3,3,3,3,3,3,3,3,3,3,3,3,3,
3,3,3,3,3,3,3,3,3,3,3,4),(0.,0.0297196497427133,0.0601024430505851,0.0895487561977697,
0.115314280201556,0.120671642680355,0.150435039105398,0.180035087607033,
0.20894455276229,0.221427550198096,0.230458612607052,0.234712819529639,
0.263250576278388,0.29115534663912,0.295672948228062,0.324625402415715,
0.334643829709069,0.339479004907797,0.343237704952895,0.371327052004073,
0.39947506248303,0.427228171302932,0.438025445099752,0.443793866239726,
0.448942908589349,0.476234910387191,0.498212935884146,0.507328822354416,
0.512108230143122,0.538127621259066,0.564147012375009,0.569248610399316),
 .UNSPECIFIED.);
#1881=B_SPLINE_CURVE_WITH_KNOTS('',3,(#20244,#20245,#20246,#20247,#20248,
#20249,#20250,#20251,#20252,#20253,#20254,#20255,#20256,#20257,#20258,#20259,
#20260,#20261,#20262,#20263,#20264,#20265,#20266,#20267,#20268,#20269,#20270,
#20271,#20272,#20273,#20274,#20275,#20276,#20277,#20278,#20279,#20280,#20281,
#20282,#20283,#20284,#20285,#20286,#20287,#20288,#20289,#20290,#20291,#20292,
#20293,#20294,#20295,#20296,#20297,#20298,#20299,#20300,#20301,#20302,#20303,
#20304,#20305,#20306,#20307,#20308,#20309,#20310,#20311,#20312,#20313,#20314,
#20315,#20316,#20317,#20318,#20319,#20320,#20321,#20322,#20323,#20324,#20325,
#20326,#20327,#20328,#20329,#20330,#20331,#20332,#20333,#20334),
 .UNSPECIFIED.,.F.,.F.,(4,3,3,3,3,3,3,3,3,3,3,3,3,3,3,3,3,3,3,3,3,3,3,3,
3,3,3,3,3,3,4),(-0.569248610399413,-0.543579424468409,-0.517280855913903,
-0.510431086725354,-0.504800591166774,-0.477739784666227,-0.455689866633776,
-0.448372084280305,-0.442463244683274,-0.414732125182678,-0.386384203988663,
-0.35844270327742,-0.343972580219404,-0.337412363788297,-0.308476675504046,
-0.301340440406619,-0.273498989180173,-0.245035069567214,-0.233720439206241,
-0.228077783767322,-0.199098902098819,-0.169542627253541,-0.139741124735967,
-0.123046353359691,-0.118258375487455,-0.114005833967889,-0.0834570417697634,
-0.0528736506474507,-0.0229280100403523,-0.00618295372576221,0.),
 .UNSPECIFIED.);
#1882=B_SPLINE_CURVE_WITH_KNOTS('',3,(#20335,#20336,#20337,#20338,#20339,
#20340,#20341,#20342,#20343,#20344,#20345,#20346,#20347,#20348,#20349,#20350,
#20351,#20352,#20353,#20354,#20355,#20356,#20357,#20358,#20359,#20360,#20361,
#20362,#20363,#20364,#20365,#20366,#20367,#20368,#20369,#20370,#20371,#20372,
#20373,#20374,#20375,#20376,#20377,#20378,#20379,#20380,#20381,#20382,#20383,
#20384,#20385,#20386,#20387,#20388,#20389,#20390,#20391,#20392,#20393,#20394,
#20395,#20396,#20397,#20398,#20399,#20400,#20401,#20402,#20403,#20404,#20405,
#20406,#20407,#20408,#20409,#20410,#20411,#20412,#20413,#20414,#20415,#20416,
#20417,#20418,#20419,#20420,#20421,#20422,#20423,#20424,#20425),
 .UNSPECIFIED.,.F.,.F.,(4,3,3,3,3,3,3,3,3,3,3,3,3,3,3,3,3,3,3,3,3,3,3,3,
3,3,3,3,3,3,4),(-0.566847306047958,-0.536668334620797,-0.506060300747489,
-0.49746296362483,-0.490486745065209,-0.460335879165694,-0.436884647019413,
-0.424130412363237,-0.418922832603944,-0.389496694866531,-0.360304026648761,
-0.332014507914833,-0.317192386434988,-0.312071036440509,-0.307326760696969,
-0.279357485335346,-0.272726021995452,-0.244230762694646,-0.214337412474756,
-0.205052718047108,-0.200811047279563,-0.172975225547944,-0.145198191396071,
-0.117889580168519,-0.103788877764395,-0.0993777847284473,-0.0726516854150365,
-0.046354856269949,-0.0208998643347332,-0.00508396093552485,0.),
 .UNSPECIFIED.);
#1883=B_SPLINE_CURVE_WITH_KNOTS('',3,(#20427,#20428,#20429,#20430,#20431,
#20432,#20433,#20434,#20435,#20436,#20437),.UNSPECIFIED.,.F.,.F.,(4,1,1,
1,1,1,1,1,4),(15.7079632679489,15.852790517907,16.8512409318069,17.8496913457067,
18.8481417596065,19.8465921735064,20.8450425874062,21.843493001306,21.9911485751285),
 .UNSPECIFIED.);
#1884=B_SPLINE_CURVE_WITH_KNOTS('',3,(#20438,#20439,#20440,#20441,#20442,
#20443,#20444,#20445,#20446,#20447),.UNSPECIFIED.,.F.,.F.,(4,1,1,1,1,1,
1,4),(15.7079632679489,16.3953009547714,17.3937513686712,18.3922017825711,
19.3906521964709,20.3891026103707,21.3875530242706,21.9911485751285),
 .UNSPECIFIED.);
#1885=B_SPLINE_CURVE_WITH_KNOTS('',3,(#20896,#20897,#20898,#20899,#20900,
#20901,#20902,#20903,#20904,#20905,#20906,#20907,#20908,#20909,#20910,#20911,
#20912,#20913,#20914,#20915,#20916,#20917,#20918,#20919,#20920,#20921,#20922,
#20923,#20924,#20925,#20926,#20927,#20928,#20929,#20930,#20931,#20932,#20933,
#20934,#20935,#20936,#20937,#20938,#20939,#20940,#20941,#20942,#20943,#20944,
#20945,#20946,#20947,#20948,#20949,#20950,#20951,#20952,#20953,#20954,#20955,
#20956,#20957,#20958,#20959,#20960,#20961,#20962,#20963,#20964,#20965,#20966,
#20967,#20968,#20969,#20970,#20971,#20972,#20973,#20974,#20975,#20976,#20977,
#20978,#20979,#20980,#20981,#20982,#20983,#20984,#20985,#20986,#20987,#20988,
#20989,#20990,#20991,#20992),.UNSPECIFIED.,.F.,.F.,(4,3,3,3,3,3,3,3,3,3,
3,3,3,3,3,3,3,3,3,3,3,3,3,3,3,3,3,3,3,3,3,3,4),(0.,0.0253580911802079,0.0513883332338855,
0.0783501043117711,0.0901458791583461,0.0965510147472824,0.102699384553703,
0.130000469046477,0.157754538584699,0.185086529402767,0.195805915508858,
0.202109172202035,0.206420354971663,0.23502272795396,0.263529291975222,
0.26708250185697,0.294995258577133,0.306190773496798,0.311403762156505,
0.315731366767556,0.343826793446803,0.372961861754818,0.402415764957967,
0.414015391046657,0.420600034660242,0.426867839516936,0.456919274359249,
0.482861619164976,0.492971552248951,0.498519433722844,0.5296040436525,0.560688653582156,
0.566847306048094),.UNSPECIFIED.);
#1886=B_SPLINE_CURVE_WITH_KNOTS('',3,(#20993,#20994,#20995,#20996,#20997,
#20998,#20999,#21000,#21001,#21002,#21003,#21004,#21005,#21006,#21007,#21008,
#21009,#21010,#21011,#21012,#21013,#21014,#21015,#21016,#21017),
 .UNSPECIFIED.,.F.,.F.,(4,3,3,3,3,3,3,3,4),(-10.1321597128207,-9.98450413899829,
-8.98605372509846,-7.98760331119863,-6.9891528972988,-5.99070248339897,
-4.99225206949914,-3.99380165559931,-3.84897440564113),.UNSPECIFIED.);
#1887=B_SPLINE_CURVE_WITH_KNOTS('',3,(#21466,#21467,#21468,#21469,#21470,
#21471,#21472,#21473,#21474,#21475,#21476,#21477,#21478,#21479,#21480,#21481,
#21482,#21483,#21484,#21485,#21486,#21487),.UNSPECIFIED.,.F.,.F.,(4,3,3,
3,3,3,3,4),(7.59274844815663,7.98760331119864,8.98605372509847,9.9845041389983,
10.9829545528981,11.981404966798,12.9798553806978,13.8759337553362),
 .UNSPECIFIED.);
#1888=B_SPLINE_CURVE_WITH_KNOTS('',3,(#21488,#21489,#21490,#21491,#21492,
#21493,#21494,#21495,#21496,#21497,#21498,#21499,#21500,#21501,#21502,#21503,
#21504,#21505,#21506,#21507,#21508,#21509,#21510,#21511,#21512,#21513,#21514,
#21515,#21516,#21517,#21518,#21519,#21520,#21521,#21522,#21523,#21524,#21525,
#21526,#21527,#21528,#21529,#21530,#21531,#21532,#21533,#21534,#21535,#21536,
#21537,#21538,#21539,#21540,#21541,#21542,#21543,#21544,#21545,#21546,#21547,
#21548,#21549,#21550,#21551,#21552,#21553,#21554,#21555,#21556,#21557,#21558,
#21559,#21560,#21561,#21562,#21563,#21564,#21565,#21566,#21567,#21568,#21569,
#21570,#21571,#21572,#21573,#21574,#21575,#21576,#21577,#21578,#21579,#21580,
#21581),.UNSPECIFIED.,.F.,.F.,(4,3,3,3,3,3,3,3,3,3,3,3,3,3,3,3,3,3,3,3,
3,3,3,3,3,3,3,3,3,3,3,4),(0.,0.0297196561791004,0.0601024527423554,0.0895487646780782,
0.115314287621836,0.120671644407955,0.15043504100573,0.180035087872894,
0.208944552961705,0.221427549682809,0.230458608873444,0.234712814484028,
0.263250569423067,0.29115533835926,0.295672948228138,0.324625402802554,
0.334643828946165,0.339479002351001,0.343237702251031,0.371327049518733,
0.399475060202899,0.427228167985078,0.438025437450442,0.443793859675948,
0.448942909106405,0.476234910274104,0.498212935799389,0.507328821201627,
0.5121082275177,0.538127619946472,0.564147012375243,0.569248610399555),
 .UNSPECIFIED.);
#2175=LINE('',#11354,#2721);
#2176=LINE('',#11363,#2722);
#2177=LINE('',#11380,#2723);
#2178=LINE('',#11428,#2724);
#2179=LINE('',#11479,#2725);
#2180=LINE('',#11527,#2726);
#2181=LINE('',#11575,#2727);
#2182=LINE('',#11626,#2728);
#2183=LINE('',#11677,#2729);
#2184=LINE('',#11725,#2730);
#2185=LINE('',#11776,#2731);
#2186=LINE('',#11827,#2732);
#2187=LINE('',#11875,#2733);
#2188=LINE('',#11923,#2734);
#2189=LINE('',#11974,#2735);
#2190=LINE('',#12025,#2736);
#2191=LINE('',#12073,#2737);
#2192=LINE('',#12124,#2738);
#2193=LINE('',#12163,#2739);
#2194=LINE('',#12187,#2740);
#2195=LINE('',#12211,#2741);
#2196=LINE('',#12236,#2742);
#2197=LINE('',#12260,#2743);
#2198=LINE('',#12285,#2744);
#2199=LINE('',#12309,#2745);
#2200=LINE('',#12334,#2746);
#2201=LINE('',#12359,#2747);
#2202=LINE('',#12383,#2748);
#2203=LINE('',#12408,#2749);
#2204=LINE('',#12432,#2750);
#2205=LINE('',#12457,#2751);
#2206=LINE('',#12481,#2752);
#2207=LINE('',#12506,#2753);
#2208=LINE('',#12531,#2754);
#2209=LINE('',#12555,#2755);
#2210=LINE('',#12572,#2756);
#2211=LINE('',#12581,#2757);
#2212=LINE('',#12598,#2758);
#2213=LINE('',#12646,#2759);
#2214=LINE('',#12697,#2760);
#2215=LINE('',#12745,#2761);
#2216=LINE('',#12793,#2762);
#2217=LINE('',#12844,#2763);
#2218=LINE('',#12895,#2764);
#2219=LINE('',#12943,#2765);
#2220=LINE('',#12994,#2766);
#2221=LINE('',#13045,#2767);
#2222=LINE('',#13093,#2768);
#2223=LINE('',#13141,#2769);
#2224=LINE('',#13192,#2770);
#2225=LINE('',#13243,#2771);
#2226=LINE('',#13291,#2772);
#2227=LINE('',#13342,#2773);
#2228=LINE('',#13381,#2774);
#2229=LINE('',#13405,#2775);
#2230=LINE('',#13429,#2776);
#2231=LINE('',#13454,#2777);
#2232=LINE('',#13478,#2778);
#2233=LINE('',#13503,#2779);
#2234=LINE('',#13527,#2780);
#2235=LINE('',#13552,#2781);
#2236=LINE('',#13577,#2782);
#2237=LINE('',#13601,#2783);
#2238=LINE('',#13626,#2784);
#2239=LINE('',#13650,#2785);
#2240=LINE('',#13675,#2786);
#2241=LINE('',#13699,#2787);
#2242=LINE('',#13724,#2788);
#2243=LINE('',#13749,#2789);
#2244=LINE('',#13773,#2790);
#2245=LINE('',#13790,#2791);
#2246=LINE('',#13799,#2792);
#2247=LINE('',#13816,#2793);
#2248=LINE('',#13864,#2794);
#2249=LINE('',#13915,#2795);
#2250=LINE('',#13963,#2796);
#2251=LINE('',#14011,#2797);
#2252=LINE('',#14062,#2798);
#2253=LINE('',#14113,#2799);
#2254=LINE('',#14161,#2800);
#2255=LINE('',#14212,#2801);
#2256=LINE('',#14263,#2802);
#2257=LINE('',#14311,#2803);
#2258=LINE('',#14359,#2804);
#2259=LINE('',#14410,#2805);
#2260=LINE('',#14461,#2806);
#2261=LINE('',#14509,#2807);
#2262=LINE('',#14560,#2808);
#2263=LINE('',#14599,#2809);
#2264=LINE('',#14623,#2810);
#2265=LINE('',#14647,#2811);
#2266=LINE('',#14672,#2812);
#2267=LINE('',#14696,#2813);
#2268=LINE('',#14721,#2814);
#2269=LINE('',#14745,#2815);
#2270=LINE('',#14770,#2816);
#2271=LINE('',#14795,#2817);
#2272=LINE('',#14819,#2818);
#2273=LINE('',#14844,#2819);
#2274=LINE('',#14868,#2820);
#2275=LINE('',#14893,#2821);
#2276=LINE('',#14917,#2822);
#2277=LINE('',#14942,#2823);
#2278=LINE('',#14967,#2824);
#2279=LINE('',#14991,#2825);
#2280=LINE('',#15008,#2826);
#2281=LINE('',#15017,#2827);
#2282=LINE('',#15034,#2828);
#2283=LINE('',#15082,#2829);
#2284=LINE('',#15133,#2830);
#2285=LINE('',#15181,#2831);
#2286=LINE('',#15229,#2832);
#2287=LINE('',#15280,#2833);
#2288=LINE('',#15331,#2834);
#2289=LINE('',#15379,#2835);
#2290=LINE('',#15430,#2836);
#2291=LINE('',#15481,#2837);
#2292=LINE('',#15529,#2838);
#2293=LINE('',#15577,#2839);
#2294=LINE('',#15628,#2840);
#2295=LINE('',#15679,#2841);
#2296=LINE('',#15727,#2842);
#2297=LINE('',#15778,#2843);
#2298=LINE('',#15817,#2844);
#2299=LINE('',#15841,#2845);
#2300=LINE('',#15865,#2846);
#2301=LINE('',#15890,#2847);
#2302=LINE('',#15914,#2848);
#2303=LINE('',#15939,#2849);
#2304=LINE('',#15963,#2850);
#2305=LINE('',#15988,#2851);
#2306=LINE('',#16013,#2852);
#2307=LINE('',#16037,#2853);
#2308=LINE('',#16062,#2854);
#2309=LINE('',#16086,#2855);
#2310=LINE('',#16111,#2856);
#2311=LINE('',#16135,#2857);
#2312=LINE('',#16160,#2858);
#2313=LINE('',#16185,#2859);
#2314=LINE('',#16209,#2860);
#2315=LINE('',#21590,#2861);
#2316=LINE('',#21592,#2862);
#2317=LINE('',#21594,#2863);
#2318=LINE('',#21595,#2864);
#2319=LINE('',#21598,#2865);
#2320=LINE('',#21600,#2866);
#2321=LINE('',#21601,#2867);
#2322=LINE('',#21604,#2868);
#2323=LINE('',#21606,#2869);
#2324=LINE('',#21607,#2870);
#2325=LINE('',#21609,#2871);
#2326=LINE('',#21610,#2872);
#2327=LINE('',#21614,#2873);
#2328=LINE('',#21616,#2874);
#2329=LINE('',#21618,#2875);
#2330=LINE('',#21619,#2876);
#2331=LINE('',#21622,#2877);
#2332=LINE('',#21624,#2878);
#2333=LINE('',#21625,#2879);
#2334=LINE('',#21628,#2880);
#2335=LINE('',#21630,#2881);
#2336=LINE('',#21631,#2882);
#2337=LINE('',#21633,#2883);
#2338=LINE('',#21634,#2884);
#2721=VECTOR('',#9535,3.);
#2722=VECTOR('',#9538,3.);
#2723=VECTOR('',#9545,3.);
#2724=VECTOR('',#9548,3.);
#2725=VECTOR('',#9551,3.);
#2726=VECTOR('',#9554,3.);
#2727=VECTOR('',#9557,3.);
#2728=VECTOR('',#9560,3.);
#2729=VECTOR('',#9563,3.);
#2730=VECTOR('',#9566,3.);
#2731=VECTOR('',#9569,3.);
#2732=VECTOR('',#9572,3.);
#2733=VECTOR('',#9575,3.);
#2734=VECTOR('',#9578,3.);
#2735=VECTOR('',#9581,3.);
#2736=VECTOR('',#9584,3.);
#2737=VECTOR('',#9587,3.);
#2738=VECTOR('',#9590,3.);
#2739=VECTOR('',#9595,3.0735);
#2740=VECTOR('',#9600,3.0735);
#2741=VECTOR('',#9603,3.0735);
#2742=VECTOR('',#9606,3.0735);
#2743=VECTOR('',#9609,3.0735);
#2744=VECTOR('',#9612,3.0735);
#2745=VECTOR('',#9615,3.0735);
#2746=VECTOR('',#9618,3.0735);
#2747=VECTOR('',#9621,3.0735);
#2748=VECTOR('',#9624,3.0735);
#2749=VECTOR('',#9627,3.0735);
#2750=VECTOR('',#9630,3.0735);
#2751=VECTOR('',#9633,3.0735);
#2752=VECTOR('',#9636,3.0735);
#2753=VECTOR('',#9639,3.0735);
#2754=VECTOR('',#9642,3.0735);
#2755=VECTOR('',#9645,3.0735);
#2756=VECTOR('',#9650,3.);
#2757=VECTOR('',#9653,3.);
#2758=VECTOR('',#9660,3.);
#2759=VECTOR('',#9663,3.);
#2760=VECTOR('',#9666,3.);
#2761=VECTOR('',#9669,3.);
#2762=VECTOR('',#9672,3.);
#2763=VECTOR('',#9675,3.);
#2764=VECTOR('',#9678,3.);
#2765=VECTOR('',#9681,3.);
#2766=VECTOR('',#9684,3.);
#2767=VECTOR('',#9687,3.);
#2768=VECTOR('',#9690,3.);
#2769=VECTOR('',#9693,3.);
#2770=VECTOR('',#9696,3.);
#2771=VECTOR('',#9699,3.);
#2772=VECTOR('',#9702,3.);
#2773=VECTOR('',#9705,3.);
#2774=VECTOR('',#9710,3.0735);
#2775=VECTOR('',#9715,3.0735);
#2776=VECTOR('',#9718,3.0735);
#2777=VECTOR('',#9721,3.0735);
#2778=VECTOR('',#9724,3.0735);
#2779=VECTOR('',#9727,3.0735);
#2780=VECTOR('',#9730,3.0735);
#2781=VECTOR('',#9733,3.0735);
#2782=VECTOR('',#9736,3.0735);
#2783=VECTOR('',#9739,3.0735);
#2784=VECTOR('',#9742,3.0735);
#2785=VECTOR('',#9745,3.0735);
#2786=VECTOR('',#9748,3.0735);
#2787=VECTOR('',#9751,3.0735);
#2788=VECTOR('',#9754,3.0735);
#2789=VECTOR('',#9757,3.0735);
#2790=VECTOR('',#9760,3.0735);
#2791=VECTOR('',#9765,3.);
#2792=VECTOR('',#9768,3.);
#2793=VECTOR('',#9775,3.);
#2794=VECTOR('',#9778,3.);
#2795=VECTOR('',#9781,3.);
#2796=VECTOR('',#9784,3.);
#2797=VECTOR('',#9787,3.);
#2798=VECTOR('',#9790,3.);
#2799=VECTOR('',#9793,3.);
#2800=VECTOR('',#9796,3.);
#2801=VECTOR('',#9799,3.);
#2802=VECTOR('',#9802,3.);
#2803=VECTOR('',#9805,3.);
#2804=VECTOR('',#9808,3.);
#2805=VECTOR('',#9811,3.);
#2806=VECTOR('',#9814,3.);
#2807=VECTOR('',#9817,3.);
#2808=VECTOR('',#9820,3.);
#2809=VECTOR('',#9825,3.07349999999996);
#2810=VECTOR('',#9830,3.07349999999996);
#2811=VECTOR('',#9833,3.07349999999996);
#2812=VECTOR('',#9836,3.07349999999996);
#2813=VECTOR('',#9839,3.07349999999996);
#2814=VECTOR('',#9842,3.07349999999996);
#2815=VECTOR('',#9845,3.07349999999996);
#2816=VECTOR('',#9848,3.07349999999996);
#2817=VECTOR('',#9851,3.07349999999996);
#2818=VECTOR('',#9854,3.07349999999996);
#2819=VECTOR('',#9857,3.07349999999996);
#2820=VECTOR('',#9860,3.07349999999996);
#2821=VECTOR('',#9863,3.07349999999996);
#2822=VECTOR('',#9866,3.07349999999996);
#2823=VECTOR('',#9869,3.07349999999996);
#2824=VECTOR('',#9872,3.07349999999996);
#2825=VECTOR('',#9875,3.07349999999996);
#2826=VECTOR('',#9880,3.);
#2827=VECTOR('',#9883,3.);
#2828=VECTOR('',#9890,3.);
#2829=VECTOR('',#9893,3.);
#2830=VECTOR('',#9896,3.);
#2831=VECTOR('',#9899,3.);
#2832=VECTOR('',#9902,3.);
#2833=VECTOR('',#9905,3.);
#2834=VECTOR('',#9908,3.);
#2835=VECTOR('',#9911,3.);
#2836=VECTOR('',#9914,3.);
#2837=VECTOR('',#9917,3.);
#2838=VECTOR('',#9920,3.);
#2839=VECTOR('',#9923,3.);
#2840=VECTOR('',#9926,3.);
#2841=VECTOR('',#9929,3.);
#2842=VECTOR('',#9932,3.);
#2843=VECTOR('',#9935,3.);
#2844=VECTOR('',#9940,3.07350000000003);
#2845=VECTOR('',#9945,3.07350000000003);
#2846=VECTOR('',#9948,3.07350000000003);
#2847=VECTOR('',#9951,3.07350000000003);
#2848=VECTOR('',#9954,3.07350000000003);
#2849=VECTOR('',#9957,3.07350000000003);
#2850=VECTOR('',#9960,3.07350000000003);
#2851=VECTOR('',#9963,3.07350000000003);
#2852=VECTOR('',#9966,3.07350000000003);
#2853=VECTOR('',#9969,3.07350000000003);
#2854=VECTOR('',#9972,3.07350000000003);
#2855=VECTOR('',#9975,3.07350000000003);
#2856=VECTOR('',#9978,3.07350000000003);
#2857=VECTOR('',#9981,3.07350000000003);
#2858=VECTOR('',#9984,3.07350000000003);
#2859=VECTOR('',#9987,3.07350000000003);
#2860=VECTOR('',#9990,3.07350000000003);
#2861=VECTOR('',#10027,10.);
#2862=VECTOR('',#10028,10.);
#2863=VECTOR('',#10029,10.);
#2864=VECTOR('',#10030,10.);
#2865=VECTOR('',#10033,10.);
#2866=VECTOR('',#10034,10.);
#2867=VECTOR('',#10035,10.);
#2868=VECTOR('',#10038,10.);
#2869=VECTOR('',#10039,10.);
#2870=VECTOR('',#10040,10.);
#2871=VECTOR('',#10043,10.);
#2872=VECTOR('',#10044,10.);
#2873=VECTOR('',#10047,10.);
#2874=VECTOR('',#10048,10.);
#2875=VECTOR('',#10049,10.);
#2876=VECTOR('',#10050,10.);
#2877=VECTOR('',#10053,10.);
#2878=VECTOR('',#10054,10.);
#2879=VECTOR('',#10055,10.);
#2880=VECTOR('',#10058,10.);
#2881=VECTOR('',#10059,10.);
#2882=VECTOR('',#10060,10.);
#2883=VECTOR('',#10063,10.);
#2884=VECTOR('',#10064,10.);
#3267=VERTEX_POINT('',#11352);
#3268=VERTEX_POINT('',#11353);
#3269=VERTEX_POINT('',#11355);
#3270=VERTEX_POINT('',#11360);
#3271=VERTEX_POINT('',#11362);
#3272=VERTEX_POINT('',#11365);
#3273=VERTEX_POINT('',#11378);
#3274=VERTEX_POINT('',#11379);
#3275=VERTEX_POINT('',#11426);
#3276=VERTEX_POINT('',#11427);
#3277=VERTEX_POINT('',#11477);
#3278=VERTEX_POINT('',#11478);
#3279=VERTEX_POINT('',#11525);
#3280=VERTEX_POINT('',#11526);
#3281=VERTEX_POINT('',#11573);
#3282=VERTEX_POINT('',#11574);
#3283=VERTEX_POINT('',#11624);
#3284=VERTEX_POINT('',#11625);
#3285=VERTEX_POINT('',#11675);
#3286=VERTEX_POINT('',#11676);
#3287=VERTEX_POINT('',#11723);
#3288=VERTEX_POINT('',#11724);
#3289=VERTEX_POINT('',#11774);
#3290=VERTEX_POINT('',#11775);
#3291=VERTEX_POINT('',#11825);
#3292=VERTEX_POINT('',#11826);
#3293=VERTEX_POINT('',#11873);
#3294=VERTEX_POINT('',#11874);
#3295=VERTEX_POINT('',#11921);
#3296=VERTEX_POINT('',#11922);
#3297=VERTEX_POINT('',#11972);
#3298=VERTEX_POINT('',#11973);
#3299=VERTEX_POINT('',#12023);
#3300=VERTEX_POINT('',#12024);
#3301=VERTEX_POINT('',#12071);
#3302=VERTEX_POINT('',#12072);
#3303=VERTEX_POINT('',#12122);
#3304=VERTEX_POINT('',#12123);
#3305=VERTEX_POINT('',#12125);
#3306=VERTEX_POINT('',#12139);
#3307=VERTEX_POINT('',#12161);
#3308=VERTEX_POINT('',#12162);
#3309=VERTEX_POINT('',#12164);
#3310=VERTEX_POINT('',#12173);
#3311=VERTEX_POINT('',#12185);
#3312=VERTEX_POINT('',#12186);
#3313=VERTEX_POINT('',#12209);
#3314=VERTEX_POINT('',#12210);
#3315=VERTEX_POINT('',#12234);
#3316=VERTEX_POINT('',#12235);
#3317=VERTEX_POINT('',#12258);
#3318=VERTEX_POINT('',#12259);
#3319=VERTEX_POINT('',#12283);
#3320=VERTEX_POINT('',#12284);
#3321=VERTEX_POINT('',#12307);
#3322=VERTEX_POINT('',#12308);
#3323=VERTEX_POINT('',#12332);
#3324=VERTEX_POINT('',#12333);
#3325=VERTEX_POINT('',#12357);
#3326=VERTEX_POINT('',#12358);
#3327=VERTEX_POINT('',#12381);
#3328=VERTEX_POINT('',#12382);
#3329=VERTEX_POINT('',#12406);
#3330=VERTEX_POINT('',#12407);
#3331=VERTEX_POINT('',#12430);
#3332=VERTEX_POINT('',#12431);
#3333=VERTEX_POINT('',#12455);
#3334=VERTEX_POINT('',#12456);
#3335=VERTEX_POINT('',#12479);
#3336=VERTEX_POINT('',#12480);
#3337=VERTEX_POINT('',#12504);
#3338=VERTEX_POINT('',#12505);
#3339=VERTEX_POINT('',#12529);
#3340=VERTEX_POINT('',#12530);
#3341=VERTEX_POINT('',#12553);
#3342=VERTEX_POINT('',#12554);
#3343=VERTEX_POINT('',#12556);
#3344=VERTEX_POINT('',#12562);
#3345=VERTEX_POINT('',#12570);
#3346=VERTEX_POINT('',#12571);
#3347=VERTEX_POINT('',#12573);
#3348=VERTEX_POINT('',#12578);
#3349=VERTEX_POINT('',#12580);
#3350=VERTEX_POINT('',#12583);
#3351=VERTEX_POINT('',#12596);
#3352=VERTEX_POINT('',#12597);
#3353=VERTEX_POINT('',#12644);
#3354=VERTEX_POINT('',#12645);
#3355=VERTEX_POINT('',#12695);
#3356=VERTEX_POINT('',#12696);
#3357=VERTEX_POINT('',#12743);
#3358=VERTEX_POINT('',#12744);
#3359=VERTEX_POINT('',#12791);
#3360=VERTEX_POINT('',#12792);
#3361=VERTEX_POINT('',#12842);
#3362=VERTEX_POINT('',#12843);
#3363=VERTEX_POINT('',#12893);
#3364=VERTEX_POINT('',#12894);
#3365=VERTEX_POINT('',#12941);
#3366=VERTEX_POINT('',#12942);
#3367=VERTEX_POINT('',#12992);
#3368=VERTEX_POINT('',#12993);
#3369=VERTEX_POINT('',#13043);
#3370=VERTEX_POINT('',#13044);
#3371=VERTEX_POINT('',#13091);
#3372=VERTEX_POINT('',#13092);
#3373=VERTEX_POINT('',#13139);
#3374=VERTEX_POINT('',#13140);
#3375=VERTEX_POINT('',#13190);
#3376=VERTEX_POINT('',#13191);
#3377=VERTEX_POINT('',#13241);
#3378=VERTEX_POINT('',#13242);
#3379=VERTEX_POINT('',#13289);
#3380=VERTEX_POINT('',#13290);
#3381=VERTEX_POINT('',#13340);
#3382=VERTEX_POINT('',#13341);
#3383=VERTEX_POINT('',#13343);
#3384=VERTEX_POINT('',#13357);
#3385=VERTEX_POINT('',#13379);
#3386=VERTEX_POINT('',#13380);
#3387=VERTEX_POINT('',#13382);
#3388=VERTEX_POINT('',#13391);
#3389=VERTEX_POINT('',#13403);
#3390=VERTEX_POINT('',#13404);
#3391=VERTEX_POINT('',#13427);
#3392=VERTEX_POINT('',#13428);
#3393=VERTEX_POINT('',#13452);
#3394=VERTEX_POINT('',#13453);
#3395=VERTEX_POINT('',#13476);
#3396=VERTEX_POINT('',#13477);
#3397=VERTEX_POINT('',#13501);
#3398=VERTEX_POINT('',#13502);
#3399=VERTEX_POINT('',#13525);
#3400=VERTEX_POINT('',#13526);
#3401=VERTEX_POINT('',#13550);
#3402=VERTEX_POINT('',#13551);
#3403=VERTEX_POINT('',#13575);
#3404=VERTEX_POINT('',#13576);
#3405=VERTEX_POINT('',#13599);
#3406=VERTEX_POINT('',#13600);
#3407=VERTEX_POINT('',#13624);
#3408=VERTEX_POINT('',#13625);
#3409=VERTEX_POINT('',#13648);
#3410=VERTEX_POINT('',#13649);
#3411=VERTEX_POINT('',#13673);
#3412=VERTEX_POINT('',#13674);
#3413=VERTEX_POINT('',#13697);
#3414=VERTEX_POINT('',#13698);
#3415=VERTEX_POINT('',#13722);
#3416=VERTEX_POINT('',#13723);
#3417=VERTEX_POINT('',#13747);
#3418=VERTEX_POINT('',#13748);
#3419=VERTEX_POINT('',#13771);
#3420=VERTEX_POINT('',#13772);
#3421=VERTEX_POINT('',#13774);
#3422=VERTEX_POINT('',#13780);
#3423=VERTEX_POINT('',#13788);
#3424=VERTEX_POINT('',#13789);
#3425=VERTEX_POINT('',#13791);
#3426=VERTEX_POINT('',#13796);
#3427=VERTEX_POINT('',#13798);
#3428=VERTEX_POINT('',#13801);
#3429=VERTEX_POINT('',#13814);
#3430=VERTEX_POINT('',#13815);
#3431=VERTEX_POINT('',#13862);
#3432=VERTEX_POINT('',#13863);
#3433=VERTEX_POINT('',#13913);
#3434=VERTEX_POINT('',#13914);
#3435=VERTEX_POINT('',#13961);
#3436=VERTEX_POINT('',#13962);
#3437=VERTEX_POINT('',#14009);
#3438=VERTEX_POINT('',#14010);
#3439=VERTEX_POINT('',#14060);
#3440=VERTEX_POINT('',#14061);
#3441=VERTEX_POINT('',#14111);
#3442=VERTEX_POINT('',#14112);
#3443=VERTEX_POINT('',#14159);
#3444=VERTEX_POINT('',#14160);
#3445=VERTEX_POINT('',#14210);
#3446=VERTEX_POINT('',#14211);
#3447=VERTEX_POINT('',#14261);
#3448=VERTEX_POINT('',#14262);
#3449=VERTEX_POINT('',#14309);
#3450=VERTEX_POINT('',#14310);
#3451=VERTEX_POINT('',#14357);
#3452=VERTEX_POINT('',#14358);
#3453=VERTEX_POINT('',#14408);
#3454=VERTEX_POINT('',#14409);
#3455=VERTEX_POINT('',#14459);
#3456=VERTEX_POINT('',#14460);
#3457=VERTEX_POINT('',#14507);
#3458=VERTEX_POINT('',#14508);
#3459=VERTEX_POINT('',#14558);
#3460=VERTEX_POINT('',#14559);
#3461=VERTEX_POINT('',#14561);
#3462=VERTEX_POINT('',#14575);
#3463=VERTEX_POINT('',#14597);
#3464=VERTEX_POINT('',#14598);
#3465=VERTEX_POINT('',#14600);
#3466=VERTEX_POINT('',#14609);
#3467=VERTEX_POINT('',#14621);
#3468=VERTEX_POINT('',#14622);
#3469=VERTEX_POINT('',#14645);
#3470=VERTEX_POINT('',#14646);
#3471=VERTEX_POINT('',#14670);
#3472=VERTEX_POINT('',#14671);
#3473=VERTEX_POINT('',#14694);
#3474=VERTEX_POINT('',#14695);
#3475=VERTEX_POINT('',#14719);
#3476=VERTEX_POINT('',#14720);
#3477=VERTEX_POINT('',#14743);
#3478=VERTEX_POINT('',#14744);
#3479=VERTEX_POINT('',#14768);
#3480=VERTEX_POINT('',#14769);
#3481=VERTEX_POINT('',#14793);
#3482=VERTEX_POINT('',#14794);
#3483=VERTEX_POINT('',#14817);
#3484=VERTEX_POINT('',#14818);
#3485=VERTEX_POINT('',#14842);
#3486=VERTEX_POINT('',#14843);
#3487=VERTEX_POINT('',#14866);
#3488=VERTEX_POINT('',#14867);
#3489=VERTEX_POINT('',#14891);
#3490=VERTEX_POINT('',#14892);
#3491=VERTEX_POINT('',#14915);
#3492=VERTEX_POINT('',#14916);
#3493=VERTEX_POINT('',#14940);
#3494=VERTEX_POINT('',#14941);
#3495=VERTEX_POINT('',#14965);
#3496=VERTEX_POINT('',#14966);
#3497=VERTEX_POINT('',#14989);
#3498=VERTEX_POINT('',#14990);
#3499=VERTEX_POINT('',#14992);
#3500=VERTEX_POINT('',#14998);
#3501=VERTEX_POINT('',#15006);
#3502=VERTEX_POINT('',#15007);
#3503=VERTEX_POINT('',#15009);
#3504=VERTEX_POINT('',#15014);
#3505=VERTEX_POINT('',#15016);
#3506=VERTEX_POINT('',#15019);
#3507=VERTEX_POINT('',#15032);
#3508=VERTEX_POINT('',#15033);
#3509=VERTEX_POINT('',#15080);
#3510=VERTEX_POINT('',#15081);
#3511=VERTEX_POINT('',#15131);
#3512=VERTEX_POINT('',#15132);
#3513=VERTEX_POINT('',#15179);
#3514=VERTEX_POINT('',#15180);
#3515=VERTEX_POINT('',#15227);
#3516=VERTEX_POINT('',#15228);
#3517=VERTEX_POINT('',#15278);
#3518=VERTEX_POINT('',#15279);
#3519=VERTEX_POINT('',#15329);
#3520=VERTEX_POINT('',#15330);
#3521=VERTEX_POINT('',#15377);
#3522=VERTEX_POINT('',#15378);
#3523=VERTEX_POINT('',#15428);
#3524=VERTEX_POINT('',#15429);
#3525=VERTEX_POINT('',#15479);
#3526=VERTEX_POINT('',#15480);
#3527=VERTEX_POINT('',#15527);
#3528=VERTEX_POINT('',#15528);
#3529=VERTEX_POINT('',#15575);
#3530=VERTEX_POINT('',#15576);
#3531=VERTEX_POINT('',#15626);
#3532=VERTEX_POINT('',#15627);
#3533=VERTEX_POINT('',#15677);
#3534=VERTEX_POINT('',#15678);
#3535=VERTEX_POINT('',#15725);
#3536=VERTEX_POINT('',#15726);
#3537=VERTEX_POINT('',#15776);
#3538=VERTEX_POINT('',#15777);
#3539=VERTEX_POINT('',#15779);
#3540=VERTEX_POINT('',#15793);
#3541=VERTEX_POINT('',#15815);
#3542=VERTEX_POINT('',#15816);
#3543=VERTEX_POINT('',#15818);
#3544=VERTEX_POINT('',#15827);
#3545=VERTEX_POINT('',#15839);
#3546=VERTEX_POINT('',#15840);
#3547=VERTEX_POINT('',#15863);
#3548=VERTEX_POINT('',#15864);
#3549=VERTEX_POINT('',#15888);
#3550=VERTEX_POINT('',#15889);
#3551=VERTEX_POINT('',#15912);
#3552=VERTEX_POINT('',#15913);
#3553=VERTEX_POINT('',#15937);
#3554=VERTEX_POINT('',#15938);
#3555=VERTEX_POINT('',#15961);
#3556=VERTEX_POINT('',#15962);
#3557=VERTEX_POINT('',#15986);
#3558=VERTEX_POINT('',#15987);
#3559=VERTEX_POINT('',#16011);
#3560=VERTEX_POINT('',#16012);
#3561=VERTEX_POINT('',#16035);
#3562=VERTEX_POINT('',#16036);
#3563=VERTEX_POINT('',#16060);
#3564=VERTEX_POINT('',#16061);
#3565=VERTEX_POINT('',#16084);
#3566=VERTEX_POINT('',#16085);
#3567=VERTEX_POINT('',#16109);
#3568=VERTEX_POINT('',#16110);
#3569=VERTEX_POINT('',#16133);
#3570=VERTEX_POINT('',#16134);
#3571=VERTEX_POINT('',#16158);
#3572=VERTEX_POINT('',#16159);
#3573=VERTEX_POINT('',#16183);
#3574=VERTEX_POINT('',#16184);
#3575=VERTEX_POINT('',#16207);
#3576=VERTEX_POINT('',#16208);
#3577=VERTEX_POINT('',#16210);
#3578=VERTEX_POINT('',#16216);
#3579=VERTEX_POINT('',#21588);
#3580=VERTEX_POINT('',#21589);
#3581=VERTEX_POINT('',#21591);
#3582=VERTEX_POINT('',#21593);
#3583=VERTEX_POINT('',#21597);
#3584=VERTEX_POINT('',#21599);
#3585=VERTEX_POINT('',#21603);
#3586=VERTEX_POINT('',#21605);
#3587=VERTEX_POINT('',#21612);
#3588=VERTEX_POINT('',#21613);
#3589=VERTEX_POINT('',#21615);
#3590=VERTEX_POINT('',#21617);
#3591=VERTEX_POINT('',#21621);
#3592=VERTEX_POINT('',#21623);
#3593=VERTEX_POINT('',#21627);
#3594=VERTEX_POINT('',#21629);
#4107=EDGE_CURVE('',#3267,#3268,#2175,.T.);
#4108=EDGE_CURVE('',#3268,#3269,#1585,.T.);
#4109=EDGE_CURVE('',#3269,#3270,#1461,.T.);
#4110=EDGE_CURVE('',#3270,#3271,#2176,.T.);
#4111=EDGE_CURVE('',#3271,#3271,#1462,.F.);
#4112=EDGE_CURVE('',#3270,#3272,#1463,.T.);
#4113=EDGE_CURVE('',#3272,#3267,#1586,.T.);
#4114=EDGE_CURVE('',#3273,#3274,#2177,.T.);
#4115=EDGE_CURVE('',#3274,#3268,#1587,.T.);
#4116=EDGE_CURVE('',#3267,#3273,#1588,.T.);
#4117=EDGE_CURVE('',#3275,#3276,#2178,.T.);
#4118=EDGE_CURVE('',#3276,#3274,#1589,.T.);
#4119=EDGE_CURVE('',#3273,#3275,#1590,.T.);
#4120=EDGE_CURVE('',#3277,#3278,#2179,.T.);
#4121=EDGE_CURVE('',#3278,#3276,#1591,.T.);
#4122=EDGE_CURVE('',#3275,#3277,#1592,.T.);
#4123=EDGE_CURVE('',#3279,#3280,#2180,.T.);
#4124=EDGE_CURVE('',#3280,#3278,#1593,.T.);
#4125=EDGE_CURVE('',#3277,#3279,#1594,.T.);
#4126=EDGE_CURVE('',#3281,#3282,#2181,.T.);
#4127=EDGE_CURVE('',#3282,#3280,#1595,.T.);
#4128=EDGE_CURVE('',#3279,#3281,#1596,.T.);
#4129=EDGE_CURVE('',#3283,#3284,#2182,.T.);
#4130=EDGE_CURVE('',#3284,#3282,#1597,.T.);
#4131=EDGE_CURVE('',#3281,#3283,#1598,.T.);
#4132=EDGE_CURVE('',#3285,#3286,#2183,.T.);
#4133=EDGE_CURVE('',#3286,#3284,#1599,.T.);
#4134=EDGE_CURVE('',#3283,#3285,#1600,.T.);
#4135=EDGE_CURVE('',#3287,#3288,#2184,.T.);
#4136=EDGE_CURVE('',#3288,#3286,#1601,.T.);
#4137=EDGE_CURVE('',#3285,#3287,#1602,.T.);
#4138=EDGE_CURVE('',#3289,#3290,#2185,.T.);
#4139=EDGE_CURVE('',#3290,#3288,#1603,.T.);
#4140=EDGE_CURVE('',#3287,#3289,#1604,.T.);
#4141=EDGE_CURVE('',#3291,#3292,#2186,.T.);
#4142=EDGE_CURVE('',#3292,#3290,#1605,.T.);
#4143=EDGE_CURVE('',#3289,#3291,#1606,.T.);
#4144=EDGE_CURVE('',#3293,#3294,#2187,.T.);
#4145=EDGE_CURVE('',#3294,#3292,#1607,.T.);
#4146=EDGE_CURVE('',#3291,#3293,#1608,.T.);
#4147=EDGE_CURVE('',#3295,#3296,#2188,.T.);
#4148=EDGE_CURVE('',#3296,#3294,#1609,.T.);
#4149=EDGE_CURVE('',#3293,#3295,#1610,.T.);
#4150=EDGE_CURVE('',#3297,#3298,#2189,.T.);
#4151=EDGE_CURVE('',#3298,#3296,#1611,.T.);
#4152=EDGE_CURVE('',#3295,#3297,#1612,.T.);
#4153=EDGE_CURVE('',#3299,#3300,#2190,.T.);
#4154=EDGE_CURVE('',#3300,#3298,#1613,.T.);
#4155=EDGE_CURVE('',#3297,#3299,#1614,.T.);
#4156=EDGE_CURVE('',#3301,#3302,#2191,.T.);
#4157=EDGE_CURVE('',#3302,#3300,#1615,.T.);
#4158=EDGE_CURVE('',#3299,#3301,#1616,.T.);
#4159=EDGE_CURVE('',#3303,#3304,#2192,.T.);
#4160=EDGE_CURVE('',#3303,#3305,#1617,.T.);
#4161=EDGE_CURVE('',#3306,#3305,#1464,.F.);
#4162=EDGE_CURVE('',#3306,#3304,#1618,.T.);
#4163=EDGE_CURVE('',#3307,#3308,#2193,.T.);
#4164=EDGE_CURVE('',#3308,#3309,#1619,.T.);
#4165=EDGE_CURVE('',#3310,#3309,#1465,.T.);
#4166=EDGE_CURVE('',#3307,#3310,#1620,.T.);
#4167=EDGE_CURVE('',#3311,#3312,#2194,.T.);
#4168=EDGE_CURVE('',#3312,#3308,#1621,.T.);
#4169=EDGE_CURVE('',#3311,#3307,#1622,.T.);
#4170=EDGE_CURVE('',#3313,#3314,#2195,.T.);
#4171=EDGE_CURVE('',#3314,#3312,#1623,.T.);
#4172=EDGE_CURVE('',#3313,#3311,#1624,.T.);
#4173=EDGE_CURVE('',#3315,#3316,#2196,.T.);
#4174=EDGE_CURVE('',#3316,#3314,#1625,.T.);
#4175=EDGE_CURVE('',#3315,#3313,#1626,.T.);
#4176=EDGE_CURVE('',#3317,#3318,#2197,.T.);
#4177=EDGE_CURVE('',#3318,#3316,#1627,.T.);
#4178=EDGE_CURVE('',#3317,#3315,#1628,.T.);
#4179=EDGE_CURVE('',#3319,#3320,#2198,.T.);
#4180=EDGE_CURVE('',#3320,#3318,#1629,.T.);
#4181=EDGE_CURVE('',#3319,#3317,#1630,.T.);
#4182=EDGE_CURVE('',#3321,#3322,#2199,.T.);
#4183=EDGE_CURVE('',#3322,#3320,#1631,.T.);
#4184=EDGE_CURVE('',#3321,#3319,#1632,.T.);
#4185=EDGE_CURVE('',#3323,#3324,#2200,.T.);
#4186=EDGE_CURVE('',#3324,#3322,#1633,.T.);
#4187=EDGE_CURVE('',#3323,#3321,#1634,.T.);
#4188=EDGE_CURVE('',#3325,#3326,#2201,.T.);
#4189=EDGE_CURVE('',#3326,#3324,#1635,.T.);
#4190=EDGE_CURVE('',#3325,#3323,#1636,.T.);
#4191=EDGE_CURVE('',#3327,#3328,#2202,.T.);
#4192=EDGE_CURVE('',#3328,#3326,#1637,.T.);
#4193=EDGE_CURVE('',#3327,#3325,#1638,.T.);
#4194=EDGE_CURVE('',#3329,#3330,#2203,.T.);
#4195=EDGE_CURVE('',#3330,#3328,#1639,.T.);
#4196=EDGE_CURVE('',#3329,#3327,#1640,.T.);
#4197=EDGE_CURVE('',#3331,#3332,#2204,.T.);
#4198=EDGE_CURVE('',#3332,#3330,#1641,.T.);
#4199=EDGE_CURVE('',#3331,#3329,#1642,.T.);
#4200=EDGE_CURVE('',#3333,#3334,#2205,.T.);
#4201=EDGE_CURVE('',#3334,#3332,#1643,.T.);
#4202=EDGE_CURVE('',#3333,#3331,#1644,.T.);
#4203=EDGE_CURVE('',#3335,#3336,#2206,.T.);
#4204=EDGE_CURVE('',#3336,#3334,#1645,.T.);
#4205=EDGE_CURVE('',#3335,#3333,#1646,.T.);
#4206=EDGE_CURVE('',#3337,#3338,#2207,.T.);
#4207=EDGE_CURVE('',#3338,#3336,#1647,.T.);
#4208=EDGE_CURVE('',#3337,#3335,#1648,.T.);
#4209=EDGE_CURVE('',#3339,#3340,#2208,.T.);
#4210=EDGE_CURVE('',#3340,#3338,#1649,.T.);
#4211=EDGE_CURVE('',#3339,#3337,#1650,.T.);
#4212=EDGE_CURVE('',#3341,#3342,#2209,.T.);
#4213=EDGE_CURVE('',#3343,#3341,#1651,.T.);
#4214=EDGE_CURVE('',#3344,#3343,#1466,.T.);
#4215=EDGE_CURVE('',#3344,#3342,#1652,.T.);
#4216=EDGE_CURVE('',#3345,#3346,#2210,.T.);
#4217=EDGE_CURVE('',#3346,#3347,#1653,.T.);
#4218=EDGE_CURVE('',#3347,#3348,#1467,.T.);
#4219=EDGE_CURVE('',#3348,#3349,#2211,.T.);
#4220=EDGE_CURVE('',#3349,#3349,#1468,.F.);
#4221=EDGE_CURVE('',#3348,#3350,#1469,.T.);
#4222=EDGE_CURVE('',#3350,#3345,#1654,.T.);
#4223=EDGE_CURVE('',#3351,#3352,#2212,.T.);
#4224=EDGE_CURVE('',#3352,#3346,#1655,.T.);
#4225=EDGE_CURVE('',#3345,#3351,#1656,.T.);
#4226=EDGE_CURVE('',#3353,#3354,#2213,.T.);
#4227=EDGE_CURVE('',#3354,#3352,#1657,.T.);
#4228=EDGE_CURVE('',#3351,#3353,#1658,.T.);
#4229=EDGE_CURVE('',#3355,#3356,#2214,.T.);
#4230=EDGE_CURVE('',#3356,#3354,#1659,.T.);
#4231=EDGE_CURVE('',#3353,#3355,#1660,.T.);
#4232=EDGE_CURVE('',#3357,#3358,#2215,.T.);
#4233=EDGE_CURVE('',#3358,#3356,#1661,.T.);
#4234=EDGE_CURVE('',#3355,#3357,#1662,.T.);
#4235=EDGE_CURVE('',#3359,#3360,#2216,.T.);
#4236=EDGE_CURVE('',#3360,#3358,#1663,.T.);
#4237=EDGE_CURVE('',#3357,#3359,#1664,.T.);
#4238=EDGE_CURVE('',#3361,#3362,#2217,.T.);
#4239=EDGE_CURVE('',#3362,#3360,#1665,.T.);
#4240=EDGE_CURVE('',#3359,#3361,#1666,.T.);
#4241=EDGE_CURVE('',#3363,#3364,#2218,.T.);
#4242=EDGE_CURVE('',#3364,#3362,#1667,.T.);
#4243=EDGE_CURVE('',#3361,#3363,#1668,.T.);
#4244=EDGE_CURVE('',#3365,#3366,#2219,.T.);
#4245=EDGE_CURVE('',#3366,#3364,#1669,.T.);
#4246=EDGE_CURVE('',#3363,#3365,#1670,.T.);
#4247=EDGE_CURVE('',#3367,#3368,#2220,.T.);
#4248=EDGE_CURVE('',#3368,#3366,#1671,.T.);
#4249=EDGE_CURVE('',#3365,#3367,#1672,.T.);
#4250=EDGE_CURVE('',#3369,#3370,#2221,.T.);
#4251=EDGE_CURVE('',#3370,#3368,#1673,.T.);
#4252=EDGE_CURVE('',#3367,#3369,#1674,.T.);
#4253=EDGE_CURVE('',#3371,#3372,#2222,.T.);
#4254=EDGE_CURVE('',#3372,#3370,#1675,.T.);
#4255=EDGE_CURVE('',#3369,#3371,#1676,.T.);
#4256=EDGE_CURVE('',#3373,#3374,#2223,.T.);
#4257=EDGE_CURVE('',#3374,#3372,#1677,.T.);
#4258=EDGE_CURVE('',#3371,#3373,#1678,.T.);
#4259=EDGE_CURVE('',#3375,#3376,#2224,.T.);
#4260=EDGE_CURVE('',#3376,#3374,#1679,.T.);
#4261=EDGE_CURVE('',#3373,#3375,#1680,.T.);
#4262=EDGE_CURVE('',#3377,#3378,#2225,.T.);
#4263=EDGE_CURVE('',#3378,#3376,#1681,.T.);
#4264=EDGE_CURVE('',#3375,#3377,#1682,.T.);
#4265=EDGE_CURVE('',#3379,#3380,#2226,.T.);
#4266=EDGE_CURVE('',#3380,#3378,#1683,.T.);
#4267=EDGE_CURVE('',#3377,#3379,#1684,.T.);
#4268=EDGE_CURVE('',#3381,#3382,#2227,.T.);
#4269=EDGE_CURVE('',#3381,#3383,#1685,.T.);
#4270=EDGE_CURVE('',#3384,#3383,#1470,.F.);
#4271=EDGE_CURVE('',#3384,#3382,#1686,.T.);
#4272=EDGE_CURVE('',#3385,#3386,#2228,.T.);
#4273=EDGE_CURVE('',#3386,#3387,#1687,.T.);
#4274=EDGE_CURVE('',#3388,#3387,#1471,.T.);
#4275=EDGE_CURVE('',#3385,#3388,#1688,.T.);
#4276=EDGE_CURVE('',#3389,#3390,#2229,.T.);
#4277=EDGE_CURVE('',#3390,#3386,#1689,.T.);
#4278=EDGE_CURVE('',#3389,#3385,#1690,.T.);
#4279=EDGE_CURVE('',#3391,#3392,#2230,.T.);
#4280=EDGE_CURVE('',#3392,#3390,#1691,.T.);
#4281=EDGE_CURVE('',#3391,#3389,#1692,.T.);
#4282=EDGE_CURVE('',#3393,#3394,#2231,.T.);
#4283=EDGE_CURVE('',#3394,#3392,#1693,.T.);
#4284=EDGE_CURVE('',#3393,#3391,#1694,.T.);
#4285=EDGE_CURVE('',#3395,#3396,#2232,.T.);
#4286=EDGE_CURVE('',#3396,#3394,#1695,.T.);
#4287=EDGE_CURVE('',#3395,#3393,#1696,.T.);
#4288=EDGE_CURVE('',#3397,#3398,#2233,.T.);
#4289=EDGE_CURVE('',#3398,#3396,#1697,.T.);
#4290=EDGE_CURVE('',#3397,#3395,#1698,.T.);
#4291=EDGE_CURVE('',#3399,#3400,#2234,.T.);
#4292=EDGE_CURVE('',#3400,#3398,#1699,.T.);
#4293=EDGE_CURVE('',#3399,#3397,#1700,.T.);
#4294=EDGE_CURVE('',#3401,#3402,#2235,.T.);
#4295=EDGE_CURVE('',#3402,#3400,#1701,.T.);
#4296=EDGE_CURVE('',#3401,#3399,#1702,.T.);
#4297=EDGE_CURVE('',#3403,#3404,#2236,.T.);
#4298=EDGE_CURVE('',#3404,#3402,#1703,.T.);
#4299=EDGE_CURVE('',#3403,#3401,#1704,.T.);
#4300=EDGE_CURVE('',#3405,#3406,#2237,.T.);
#4301=EDGE_CURVE('',#3406,#3404,#1705,.T.);
#4302=EDGE_CURVE('',#3405,#3403,#1706,.T.);
#4303=EDGE_CURVE('',#3407,#3408,#2238,.T.);
#4304=EDGE_CURVE('',#3408,#3406,#1707,.T.);
#4305=EDGE_CURVE('',#3407,#3405,#1708,.T.);
#4306=EDGE_CURVE('',#3409,#3410,#2239,.T.);
#4307=EDGE_CURVE('',#3410,#3408,#1709,.T.);
#4308=EDGE_CURVE('',#3409,#3407,#1710,.T.);
#4309=EDGE_CURVE('',#3411,#3412,#2240,.T.);
#4310=EDGE_CURVE('',#3412,#3410,#1711,.T.);
#4311=EDGE_CURVE('',#3411,#3409,#1712,.T.);
#4312=EDGE_CURVE('',#3413,#3414,#2241,.T.);
#4313=EDGE_CURVE('',#3414,#3412,#1713,.T.);
#4314=EDGE_CURVE('',#3413,#3411,#1714,.T.);
#4315=EDGE_CURVE('',#3415,#3416,#2242,.T.);
#4316=EDGE_CURVE('',#3416,#3414,#1715,.T.);
#4317=EDGE_CURVE('',#3415,#3413,#1716,.T.);
#4318=EDGE_CURVE('',#3417,#3418,#2243,.T.);
#4319=EDGE_CURVE('',#3418,#3416,#1717,.T.);
#4320=EDGE_CURVE('',#3417,#3415,#1718,.T.);
#4321=EDGE_CURVE('',#3419,#3420,#2244,.T.);
#4322=EDGE_CURVE('',#3421,#3419,#1719,.T.);
#4323=EDGE_CURVE('',#3422,#3421,#1472,.T.);
#4324=EDGE_CURVE('',#3422,#3420,#1720,.T.);
#4325=EDGE_CURVE('',#3423,#3424,#2245,.T.);
#4326=EDGE_CURVE('',#3424,#3425,#1721,.T.);
#4327=EDGE_CURVE('',#3425,#3426,#1473,.T.);
#4328=EDGE_CURVE('',#3426,#3427,#2246,.T.);
#4329=EDGE_CURVE('',#3427,#3427,#1474,.F.);
#4330=EDGE_CURVE('',#3426,#3428,#1475,.T.);
#4331=EDGE_CURVE('',#3428,#3423,#1722,.T.);
#4332=EDGE_CURVE('',#3429,#3430,#2247,.T.);
#4333=EDGE_CURVE('',#3430,#3424,#1723,.T.);
#4334=EDGE_CURVE('',#3423,#3429,#1724,.T.);
#4335=EDGE_CURVE('',#3431,#3432,#2248,.T.);
#4336=EDGE_CURVE('',#3432,#3430,#1725,.T.);
#4337=EDGE_CURVE('',#3429,#3431,#1726,.T.);
#4338=EDGE_CURVE('',#3433,#3434,#2249,.T.);
#4339=EDGE_CURVE('',#3434,#3432,#1727,.T.);
#4340=EDGE_CURVE('',#3431,#3433,#1728,.T.);
#4341=EDGE_CURVE('',#3435,#3436,#2250,.T.);
#4342=EDGE_CURVE('',#3436,#3434,#1729,.T.);
#4343=EDGE_CURVE('',#3433,#3435,#1730,.T.);
#4344=EDGE_CURVE('',#3437,#3438,#2251,.T.);
#4345=EDGE_CURVE('',#3438,#3436,#1731,.T.);
#4346=EDGE_CURVE('',#3435,#3437,#1732,.T.);
#4347=EDGE_CURVE('',#3439,#3440,#2252,.T.);
#4348=EDGE_CURVE('',#3440,#3438,#1733,.T.);
#4349=EDGE_CURVE('',#3437,#3439,#1734,.T.);
#4350=EDGE_CURVE('',#3441,#3442,#2253,.T.);
#4351=EDGE_CURVE('',#3442,#3440,#1735,.T.);
#4352=EDGE_CURVE('',#3439,#3441,#1736,.T.);
#4353=EDGE_CURVE('',#3443,#3444,#2254,.T.);
#4354=EDGE_CURVE('',#3444,#3442,#1737,.T.);
#4355=EDGE_CURVE('',#3441,#3443,#1738,.T.);
#4356=EDGE_CURVE('',#3445,#3446,#2255,.T.);
#4357=EDGE_CURVE('',#3446,#3444,#1739,.T.);
#4358=EDGE_CURVE('',#3443,#3445,#1740,.T.);
#4359=EDGE_CURVE('',#3447,#3448,#2256,.T.);
#4360=EDGE_CURVE('',#3448,#3446,#1741,.T.);
#4361=EDGE_CURVE('',#3445,#3447,#1742,.T.);
#4362=EDGE_CURVE('',#3449,#3450,#2257,.T.);
#4363=EDGE_CURVE('',#3450,#3448,#1743,.T.);
#4364=EDGE_CURVE('',#3447,#3449,#1744,.T.);
#4365=EDGE_CURVE('',#3451,#3452,#2258,.T.);
#4366=EDGE_CURVE('',#3452,#3450,#1745,.T.);
#4367=EDGE_CURVE('',#3449,#3451,#1746,.T.);
#4368=EDGE_CURVE('',#3453,#3454,#2259,.T.);
#4369=EDGE_CURVE('',#3454,#3452,#1747,.T.);
#4370=EDGE_CURVE('',#3451,#3453,#1748,.T.);
#4371=EDGE_CURVE('',#3455,#3456,#2260,.T.);
#4372=EDGE_CURVE('',#3456,#3454,#1749,.T.);
#4373=EDGE_CURVE('',#3453,#3455,#1750,.T.);
#4374=EDGE_CURVE('',#3457,#3458,#2261,.T.);
#4375=EDGE_CURVE('',#3458,#3456,#1751,.T.);
#4376=EDGE_CURVE('',#3455,#3457,#1752,.T.);
#4377=EDGE_CURVE('',#3459,#3460,#2262,.T.);
#4378=EDGE_CURVE('',#3459,#3461,#1753,.T.);
#4379=EDGE_CURVE('',#3462,#3461,#1476,.F.);
#4380=EDGE_CURVE('',#3462,#3460,#1754,.T.);
#4381=EDGE_CURVE('',#3463,#3464,#2263,.T.);
#4382=EDGE_CURVE('',#3464,#3465,#1755,.T.);
#4383=EDGE_CURVE('',#3466,#3465,#1477,.T.);
#4384=EDGE_CURVE('',#3463,#3466,#1756,.T.);
#4385=EDGE_CURVE('',#3467,#3468,#2264,.T.);
#4386=EDGE_CURVE('',#3468,#3464,#1757,.T.);
#4387=EDGE_CURVE('',#3467,#3463,#1758,.T.);
#4388=EDGE_CURVE('',#3469,#3470,#2265,.T.);
#4389=EDGE_CURVE('',#3470,#3468,#1759,.T.);
#4390=EDGE_CURVE('',#3469,#3467,#1760,.T.);
#4391=EDGE_CURVE('',#3471,#3472,#2266,.T.);
#4392=EDGE_CURVE('',#3472,#3470,#1761,.T.);
#4393=EDGE_CURVE('',#3471,#3469,#1762,.T.);
#4394=EDGE_CURVE('',#3473,#3474,#2267,.T.);
#4395=EDGE_CURVE('',#3474,#3472,#1763,.T.);
#4396=EDGE_CURVE('',#3473,#3471,#1764,.T.);
#4397=EDGE_CURVE('',#3475,#3476,#2268,.T.);
#4398=EDGE_CURVE('',#3476,#3474,#1765,.T.);
#4399=EDGE_CURVE('',#3475,#3473,#1766,.T.);
#4400=EDGE_CURVE('',#3477,#3478,#2269,.T.);
#4401=EDGE_CURVE('',#3478,#3476,#1767,.T.);
#4402=EDGE_CURVE('',#3477,#3475,#1768,.T.);
#4403=EDGE_CURVE('',#3479,#3480,#2270,.T.);
#4404=EDGE_CURVE('',#3480,#3478,#1769,.T.);
#4405=EDGE_CURVE('',#3479,#3477,#1770,.T.);
#4406=EDGE_CURVE('',#3481,#3482,#2271,.T.);
#4407=EDGE_CURVE('',#3482,#3480,#1771,.T.);
#4408=EDGE_CURVE('',#3481,#3479,#1772,.T.);
#4409=EDGE_CURVE('',#3483,#3484,#2272,.T.);
#4410=EDGE_CURVE('',#3484,#3482,#1773,.T.);
#4411=EDGE_CURVE('',#3483,#3481,#1774,.T.);
#4412=EDGE_CURVE('',#3485,#3486,#2273,.T.);
#4413=EDGE_CURVE('',#3486,#3484,#1775,.T.);
#4414=EDGE_CURVE('',#3485,#3483,#1776,.T.);
#4415=EDGE_CURVE('',#3487,#3488,#2274,.T.);
#4416=EDGE_CURVE('',#3488,#3486,#1777,.T.);
#4417=EDGE_CURVE('',#3487,#3485,#1778,.T.);
#4418=EDGE_CURVE('',#3489,#3490,#2275,.T.);
#4419=EDGE_CURVE('',#3490,#3488,#1779,.T.);
#4420=EDGE_CURVE('',#3489,#3487,#1780,.T.);
#4421=EDGE_CURVE('',#3491,#3492,#2276,.T.);
#4422=EDGE_CURVE('',#3492,#3490,#1781,.T.);
#4423=EDGE_CURVE('',#3491,#3489,#1782,.T.);
#4424=EDGE_CURVE('',#3493,#3494,#2277,.T.);
#4425=EDGE_CURVE('',#3494,#3492,#1783,.T.);
#4426=EDGE_CURVE('',#3493,#3491,#1784,.T.);
#4427=EDGE_CURVE('',#3495,#3496,#2278,.T.);
#4428=EDGE_CURVE('',#3496,#3494,#1785,.T.);
#4429=EDGE_CURVE('',#3495,#3493,#1786,.T.);
#4430=EDGE_CURVE('',#3497,#3498,#2279,.T.);
#4431=EDGE_CURVE('',#3499,#3497,#1787,.T.);
#4432=EDGE_CURVE('',#3500,#3499,#1478,.T.);
#4433=EDGE_CURVE('',#3500,#3498,#1788,.T.);
#4434=EDGE_CURVE('',#3501,#3502,#2280,.T.);
#4435=EDGE_CURVE('',#3502,#3503,#1789,.T.);
#4436=EDGE_CURVE('',#3503,#3504,#1479,.T.);
#4437=EDGE_CURVE('',#3504,#3505,#2281,.T.);
#4438=EDGE_CURVE('',#3505,#3505,#1480,.F.);
#4439=EDGE_CURVE('',#3504,#3506,#1481,.T.);
#4440=EDGE_CURVE('',#3506,#3501,#1790,.T.);
#4441=EDGE_CURVE('',#3507,#3508,#2282,.T.);
#4442=EDGE_CURVE('',#3508,#3502,#1791,.T.);
#4443=EDGE_CURVE('',#3501,#3507,#1792,.T.);
#4444=EDGE_CURVE('',#3509,#3510,#2283,.T.);
#4445=EDGE_CURVE('',#3510,#3508,#1793,.T.);
#4446=EDGE_CURVE('',#3507,#3509,#1794,.T.);
#4447=EDGE_CURVE('',#3511,#3512,#2284,.T.);
#4448=EDGE_CURVE('',#3512,#3510,#1795,.T.);
#4449=EDGE_CURVE('',#3509,#3511,#1796,.T.);
#4450=EDGE_CURVE('',#3513,#3514,#2285,.T.);
#4451=EDGE_CURVE('',#3514,#3512,#1797,.T.);
#4452=EDGE_CURVE('',#3511,#3513,#1798,.T.);
#4453=EDGE_CURVE('',#3515,#3516,#2286,.T.);
#4454=EDGE_CURVE('',#3516,#3514,#1799,.T.);
#4455=EDGE_CURVE('',#3513,#3515,#1800,.T.);
#4456=EDGE_CURVE('',#3517,#3518,#2287,.T.);
#4457=EDGE_CURVE('',#3518,#3516,#1801,.T.);
#4458=EDGE_CURVE('',#3515,#3517,#1802,.T.);
#4459=EDGE_CURVE('',#3519,#3520,#2288,.T.);
#4460=EDGE_CURVE('',#3520,#3518,#1803,.T.);
#4461=EDGE_CURVE('',#3517,#3519,#1804,.T.);
#4462=EDGE_CURVE('',#3521,#3522,#2289,.T.);
#4463=EDGE_CURVE('',#3522,#3520,#1805,.T.);
#4464=EDGE_CURVE('',#3519,#3521,#1806,.T.);
#4465=EDGE_CURVE('',#3523,#3524,#2290,.T.);
#4466=EDGE_CURVE('',#3524,#3522,#1807,.T.);
#4467=EDGE_CURVE('',#3521,#3523,#1808,.T.);
#4468=EDGE_CURVE('',#3525,#3526,#2291,.T.);
#4469=EDGE_CURVE('',#3526,#3524,#1809,.T.);
#4470=EDGE_CURVE('',#3523,#3525,#1810,.T.);
#4471=EDGE_CURVE('',#3527,#3528,#2292,.T.);
#4472=EDGE_CURVE('',#3528,#3526,#1811,.T.);
#4473=EDGE_CURVE('',#3525,#3527,#1812,.T.);
#4474=EDGE_CURVE('',#3529,#3530,#2293,.T.);
#4475=EDGE_CURVE('',#3530,#3528,#1813,.T.);
#4476=EDGE_CURVE('',#3527,#3529,#1814,.T.);
#4477=EDGE_CURVE('',#3531,#3532,#2294,.T.);
#4478=EDGE_CURVE('',#3532,#3530,#1815,.T.);
#4479=EDGE_CURVE('',#3529,#3531,#1816,.T.);
#4480=EDGE_CURVE('',#3533,#3534,#2295,.T.);
#4481=EDGE_CURVE('',#3534,#3532,#1817,.T.);
#4482=EDGE_CURVE('',#3531,#3533,#1818,.T.);
#4483=EDGE_CURVE('',#3535,#3536,#2296,.T.);
#4484=EDGE_CURVE('',#3536,#3534,#1819,.T.);
#4485=EDGE_CURVE('',#3533,#3535,#1820,.T.);
#4486=EDGE_CURVE('',#3537,#3538,#2297,.T.);
#4487=EDGE_CURVE('',#3537,#3539,#1821,.T.);
#4488=EDGE_CURVE('',#3540,#3539,#1482,.F.);
#4489=EDGE_CURVE('',#3540,#3538,#1822,.T.);
#4490=EDGE_CURVE('',#3541,#3542,#2298,.T.);
#4491=EDGE_CURVE('',#3542,#3543,#1823,.T.);
#4492=EDGE_CURVE('',#3544,#3543,#1483,.T.);
#4493=EDGE_CURVE('',#3541,#3544,#1824,.T.);
#4494=EDGE_CURVE('',#3545,#3546,#2299,.T.);
#4495=EDGE_CURVE('',#3546,#3542,#1825,.T.);
#4496=EDGE_CURVE('',#3545,#3541,#1826,.T.);
#4497=EDGE_CURVE('',#3547,#3548,#2300,.T.);
#4498=EDGE_CURVE('',#3548,#3546,#1827,.T.);
#4499=EDGE_CURVE('',#3547,#3545,#1828,.T.);
#4500=EDGE_CURVE('',#3549,#3550,#2301,.T.);
#4501=EDGE_CURVE('',#3550,#3548,#1829,.T.);
#4502=EDGE_CURVE('',#3549,#3547,#1830,.T.);
#4503=EDGE_CURVE('',#3551,#3552,#2302,.T.);
#4504=EDGE_CURVE('',#3552,#3550,#1831,.T.);
#4505=EDGE_CURVE('',#3551,#3549,#1832,.T.);
#4506=EDGE_CURVE('',#3553,#3554,#2303,.T.);
#4507=EDGE_CURVE('',#3554,#3552,#1833,.T.);
#4508=EDGE_CURVE('',#3553,#3551,#1834,.T.);
#4509=EDGE_CURVE('',#3555,#3556,#2304,.T.);
#4510=EDGE_CURVE('',#3556,#3554,#1835,.T.);
#4511=EDGE_CURVE('',#3555,#3553,#1836,.T.);
#4512=EDGE_CURVE('',#3557,#3558,#2305,.T.);
#4513=EDGE_CURVE('',#3558,#3556,#1837,.T.);
#4514=EDGE_CURVE('',#3557,#3555,#1838,.T.);
#4515=EDGE_CURVE('',#3559,#3560,#2306,.T.);
#4516=EDGE_CURVE('',#3560,#3558,#1839,.T.);
#4517=EDGE_CURVE('',#3559,#3557,#1840,.T.);
#4518=EDGE_CURVE('',#3561,#3562,#2307,.T.);
#4519=EDGE_CURVE('',#3562,#3560,#1841,.T.);
#4520=EDGE_CURVE('',#3561,#3559,#1842,.T.);
#4521=EDGE_CURVE('',#3563,#3564,#2308,.T.);
#4522=EDGE_CURVE('',#3564,#3562,#1843,.T.);
#4523=EDGE_CURVE('',#3563,#3561,#1844,.T.);
#4524=EDGE_CURVE('',#3565,#3566,#2309,.T.);
#4525=EDGE_CURVE('',#3566,#3564,#1845,.T.);
#4526=EDGE_CURVE('',#3565,#3563,#1846,.T.);
#4527=EDGE_CURVE('',#3567,#3568,#2310,.T.);
#4528=EDGE_CURVE('',#3568,#3566,#1847,.T.);
#4529=EDGE_CURVE('',#3567,#3565,#1848,.T.);
#4530=EDGE_CURVE('',#3569,#3570,#2311,.T.);
#4531=EDGE_CURVE('',#3570,#3568,#1849,.T.);
#4532=EDGE_CURVE('',#3569,#3567,#1850,.T.);
#4533=EDGE_CURVE('',#3571,#3572,#2312,.T.);
#4534=EDGE_CURVE('',#3572,#3570,#1851,.T.);
#4535=EDGE_CURVE('',#3571,#3569,#1852,.T.);
#4536=EDGE_CURVE('',#3573,#3574,#2313,.T.);
#4537=EDGE_CURVE('',#3574,#3572,#1853,.T.);
#4538=EDGE_CURVE('',#3573,#3571,#1854,.T.);
#4539=EDGE_CURVE('',#3575,#3576,#2314,.T.);
#4540=EDGE_CURVE('',#3577,#3575,#1855,.T.);
#4541=EDGE_CURVE('',#3578,#3577,#1484,.T.);
#4542=EDGE_CURVE('',#3578,#3576,#1856,.T.);
#4543=EDGE_CURVE('',#3503,#3544,#1857,.T.);
#4544=EDGE_CURVE('',#3543,#3506,#1858,.T.);
#4545=EDGE_CURVE('',#3576,#3574,#1859,.T.);
#4546=EDGE_CURVE('',#3575,#3573,#1860,.T.);
#4547=EDGE_CURVE('',#3539,#3578,#1861,.T.);
#4548=EDGE_CURVE('',#3535,#3537,#1862,.T.);
#4549=EDGE_CURVE('',#3538,#3536,#1863,.T.);
#4550=EDGE_CURVE('',#3577,#3540,#1864,.T.);
#4551=EDGE_CURVE('',#3425,#3466,#1865,.T.);
#4552=EDGE_CURVE('',#3465,#3428,#1866,.T.);
#4553=EDGE_CURVE('',#3498,#3496,#1867,.T.);
#4554=EDGE_CURVE('',#3497,#3495,#1868,.T.);
#4555=EDGE_CURVE('',#3461,#3500,#1869,.T.);
#4556=EDGE_CURVE('',#3457,#3459,#1870,.T.);
#4557=EDGE_CURVE('',#3460,#3458,#1871,.T.);
#4558=EDGE_CURVE('',#3499,#3462,#1872,.T.);
#4559=EDGE_CURVE('',#3347,#3388,#1873,.T.);
#4560=EDGE_CURVE('',#3387,#3350,#1874,.T.);
#4561=EDGE_CURVE('',#3420,#3418,#1875,.T.);
#4562=EDGE_CURVE('',#3419,#3417,#1876,.T.);
#4563=EDGE_CURVE('',#3383,#3422,#1877,.T.);
#4564=EDGE_CURVE('',#3379,#3381,#1878,.T.);
#4565=EDGE_CURVE('',#3382,#3380,#1879,.T.);
#4566=EDGE_CURVE('',#3421,#3384,#1880,.T.);
#4567=EDGE_CURVE('',#3269,#3310,#1881,.T.);
#4568=EDGE_CURVE('',#3309,#3272,#1882,.T.);
#4569=EDGE_CURVE('',#3342,#3340,#1883,.T.);
#4570=EDGE_CURVE('',#3341,#3339,#1884,.T.);
#4571=EDGE_CURVE('',#3305,#3344,#1885,.T.);
#4572=EDGE_CURVE('',#3301,#3303,#1886,.T.);
#4573=EDGE_CURVE('',#3304,#3302,#1887,.T.);
#4574=EDGE_CURVE('',#3343,#3306,#1888,.T.);
#4575=EDGE_CURVE('',#3579,#3580,#2315,.T.);
#4576=EDGE_CURVE('',#3580,#3581,#2316,.T.);
#4577=EDGE_CURVE('',#3582,#3581,#2317,.T.);
#4578=EDGE_CURVE('',#3579,#3582,#2318,.T.);
#4579=EDGE_CURVE('',#3583,#3579,#2319,.T.);
#4580=EDGE_CURVE('',#3584,#3582,#2320,.T.);
#4581=EDGE_CURVE('',#3583,#3584,#2321,.T.);
#4582=EDGE_CURVE('',#3585,#3583,#2322,.T.);
#4583=EDGE_CURVE('',#3586,#3584,#2323,.T.);
#4584=EDGE_CURVE('',#3585,#3586,#2324,.T.);
#4585=EDGE_CURVE('',#3580,#3585,#2325,.T.);
#4586=EDGE_CURVE('',#3581,#3586,#2326,.T.);
#4587=EDGE_CURVE('',#3587,#3588,#2327,.F.);
#4588=EDGE_CURVE('',#3588,#3589,#2328,.T.);
#4589=EDGE_CURVE('',#3590,#3589,#2329,.F.);
#4590=EDGE_CURVE('',#3587,#3590,#2330,.F.);
#4591=EDGE_CURVE('',#3591,#3587,#2331,.F.);
#4592=EDGE_CURVE('',#3592,#3590,#2332,.F.);
#4593=EDGE_CURVE('',#3591,#3592,#2333,.F.);
#4594=EDGE_CURVE('',#3593,#3591,#2334,.F.);
#4595=EDGE_CURVE('',#3594,#3592,#2335,.F.);
#4596=EDGE_CURVE('',#3593,#3594,#2336,.T.);
#4597=EDGE_CURVE('',#3588,#3593,#2337,.F.);
#4598=EDGE_CURVE('',#3589,#3594,#2338,.F.);
#5367=ORIENTED_EDGE('',*,*,#4107,.T.);
#5368=ORIENTED_EDGE('',*,*,#4108,.T.);
#5369=ORIENTED_EDGE('',*,*,#4109,.T.);
#5370=ORIENTED_EDGE('',*,*,#4110,.T.);
#5371=ORIENTED_EDGE('',*,*,#4111,.T.);
#5372=ORIENTED_EDGE('',*,*,#4110,.F.);
#5373=ORIENTED_EDGE('',*,*,#4112,.T.);
#5374=ORIENTED_EDGE('',*,*,#4113,.T.);
#5375=ORIENTED_EDGE('',*,*,#4114,.T.);
#5376=ORIENTED_EDGE('',*,*,#4115,.T.);
#5377=ORIENTED_EDGE('',*,*,#4107,.F.);
#5378=ORIENTED_EDGE('',*,*,#4116,.T.);
#5379=ORIENTED_EDGE('',*,*,#4117,.T.);
#5380=ORIENTED_EDGE('',*,*,#4118,.T.);
#5381=ORIENTED_EDGE('',*,*,#4114,.F.);
#5382=ORIENTED_EDGE('',*,*,#4119,.T.);
#5383=ORIENTED_EDGE('',*,*,#4120,.T.);
#5384=ORIENTED_EDGE('',*,*,#4121,.T.);
#5385=ORIENTED_EDGE('',*,*,#4117,.F.);
#5386=ORIENTED_EDGE('',*,*,#4122,.T.);
#5387=ORIENTED_EDGE('',*,*,#4123,.T.);
#5388=ORIENTED_EDGE('',*,*,#4124,.T.);
#5389=ORIENTED_EDGE('',*,*,#4120,.F.);
#5390=ORIENTED_EDGE('',*,*,#4125,.T.);
#5391=ORIENTED_EDGE('',*,*,#4126,.T.);
#5392=ORIENTED_EDGE('',*,*,#4127,.T.);
#5393=ORIENTED_EDGE('',*,*,#4123,.F.);
#5394=ORIENTED_EDGE('',*,*,#4128,.T.);
#5395=ORIENTED_EDGE('',*,*,#4129,.T.);
#5396=ORIENTED_EDGE('',*,*,#4130,.T.);
#5397=ORIENTED_EDGE('',*,*,#4126,.F.);
#5398=ORIENTED_EDGE('',*,*,#4131,.T.);
#5399=ORIENTED_EDGE('',*,*,#4132,.T.);
#5400=ORIENTED_EDGE('',*,*,#4133,.T.);
#5401=ORIENTED_EDGE('',*,*,#4129,.F.);
#5402=ORIENTED_EDGE('',*,*,#4134,.T.);
#5403=ORIENTED_EDGE('',*,*,#4135,.T.);
#5404=ORIENTED_EDGE('',*,*,#4136,.T.);
#5405=ORIENTED_EDGE('',*,*,#4132,.F.);
#5406=ORIENTED_EDGE('',*,*,#4137,.T.);
#5407=ORIENTED_EDGE('',*,*,#4138,.T.);
#5408=ORIENTED_EDGE('',*,*,#4139,.T.);
#5409=ORIENTED_EDGE('',*,*,#4135,.F.);
#5410=ORIENTED_EDGE('',*,*,#4140,.T.);
#5411=ORIENTED_EDGE('',*,*,#4141,.T.);
#5412=ORIENTED_EDGE('',*,*,#4142,.T.);
#5413=ORIENTED_EDGE('',*,*,#4138,.F.);
#5414=ORIENTED_EDGE('',*,*,#4143,.T.);
#5415=ORIENTED_EDGE('',*,*,#4144,.T.);
#5416=ORIENTED_EDGE('',*,*,#4145,.T.);
#5417=ORIENTED_EDGE('',*,*,#4141,.F.);
#5418=ORIENTED_EDGE('',*,*,#4146,.T.);
#5419=ORIENTED_EDGE('',*,*,#4147,.T.);
#5420=ORIENTED_EDGE('',*,*,#4148,.T.);
#5421=ORIENTED_EDGE('',*,*,#4144,.F.);
#5422=ORIENTED_EDGE('',*,*,#4149,.T.);
#5423=ORIENTED_EDGE('',*,*,#4150,.T.);
#5424=ORIENTED_EDGE('',*,*,#4151,.T.);
#5425=ORIENTED_EDGE('',*,*,#4147,.F.);
#5426=ORIENTED_EDGE('',*,*,#4152,.T.);
#5427=ORIENTED_EDGE('',*,*,#4153,.T.);
#5428=ORIENTED_EDGE('',*,*,#4154,.T.);
#5429=ORIENTED_EDGE('',*,*,#4150,.F.);
#5430=ORIENTED_EDGE('',*,*,#4155,.T.);
#5431=ORIENTED_EDGE('',*,*,#4156,.T.);
#5432=ORIENTED_EDGE('',*,*,#4157,.T.);
#5433=ORIENTED_EDGE('',*,*,#4153,.F.);
#5434=ORIENTED_EDGE('',*,*,#4158,.T.);
#5435=ORIENTED_EDGE('',*,*,#4159,.F.);
#5436=ORIENTED_EDGE('',*,*,#4160,.T.);
#5437=ORIENTED_EDGE('',*,*,#4161,.F.);
#5438=ORIENTED_EDGE('',*,*,#4162,.T.);
#5439=ORIENTED_EDGE('',*,*,#4163,.T.);
#5440=ORIENTED_EDGE('',*,*,#4164,.T.);
#5441=ORIENTED_EDGE('',*,*,#4165,.F.);
#5442=ORIENTED_EDGE('',*,*,#4166,.F.);
#5443=ORIENTED_EDGE('',*,*,#4167,.T.);
#5444=ORIENTED_EDGE('',*,*,#4168,.T.);
#5445=ORIENTED_EDGE('',*,*,#4163,.F.);
#5446=ORIENTED_EDGE('',*,*,#4169,.F.);
#5447=ORIENTED_EDGE('',*,*,#4170,.T.);
#5448=ORIENTED_EDGE('',*,*,#4171,.T.);
#5449=ORIENTED_EDGE('',*,*,#4167,.F.);
#5450=ORIENTED_EDGE('',*,*,#4172,.F.);
#5451=ORIENTED_EDGE('',*,*,#4173,.T.);
#5452=ORIENTED_EDGE('',*,*,#4174,.T.);
#5453=ORIENTED_EDGE('',*,*,#4170,.F.);
#5454=ORIENTED_EDGE('',*,*,#4175,.F.);
#5455=ORIENTED_EDGE('',*,*,#4176,.T.);
#5456=ORIENTED_EDGE('',*,*,#4177,.T.);
#5457=ORIENTED_EDGE('',*,*,#4173,.F.);
#5458=ORIENTED_EDGE('',*,*,#4178,.F.);
#5459=ORIENTED_EDGE('',*,*,#4179,.T.);
#5460=ORIENTED_EDGE('',*,*,#4180,.T.);
#5461=ORIENTED_EDGE('',*,*,#4176,.F.);
#5462=ORIENTED_EDGE('',*,*,#4181,.F.);
#5463=ORIENTED_EDGE('',*,*,#4182,.T.);
#5464=ORIENTED_EDGE('',*,*,#4183,.T.);
#5465=ORIENTED_EDGE('',*,*,#4179,.F.);
#5466=ORIENTED_EDGE('',*,*,#4184,.F.);
#5467=ORIENTED_EDGE('',*,*,#4185,.T.);
#5468=ORIENTED_EDGE('',*,*,#4186,.T.);
#5469=ORIENTED_EDGE('',*,*,#4182,.F.);
#5470=ORIENTED_EDGE('',*,*,#4187,.F.);
#5471=ORIENTED_EDGE('',*,*,#4188,.T.);
#5472=ORIENTED_EDGE('',*,*,#4189,.T.);
#5473=ORIENTED_EDGE('',*,*,#4185,.F.);
#5474=ORIENTED_EDGE('',*,*,#4190,.F.);
#5475=ORIENTED_EDGE('',*,*,#4191,.T.);
#5476=ORIENTED_EDGE('',*,*,#4192,.T.);
#5477=ORIENTED_EDGE('',*,*,#4188,.F.);
#5478=ORIENTED_EDGE('',*,*,#4193,.F.);
#5479=ORIENTED_EDGE('',*,*,#4194,.T.);
#5480=ORIENTED_EDGE('',*,*,#4195,.T.);
#5481=ORIENTED_EDGE('',*,*,#4191,.F.);
#5482=ORIENTED_EDGE('',*,*,#4196,.F.);
#5483=ORIENTED_EDGE('',*,*,#4197,.T.);
#5484=ORIENTED_EDGE('',*,*,#4198,.T.);
#5485=ORIENTED_EDGE('',*,*,#4194,.F.);
#5486=ORIENTED_EDGE('',*,*,#4199,.F.);
#5487=ORIENTED_EDGE('',*,*,#4200,.T.);
#5488=ORIENTED_EDGE('',*,*,#4201,.T.);
#5489=ORIENTED_EDGE('',*,*,#4197,.F.);
#5490=ORIENTED_EDGE('',*,*,#4202,.F.);
#5491=ORIENTED_EDGE('',*,*,#4203,.T.);
#5492=ORIENTED_EDGE('',*,*,#4204,.T.);
#5493=ORIENTED_EDGE('',*,*,#4200,.F.);
#5494=ORIENTED_EDGE('',*,*,#4205,.F.);
#5495=ORIENTED_EDGE('',*,*,#4206,.T.);
#5496=ORIENTED_EDGE('',*,*,#4207,.T.);
#5497=ORIENTED_EDGE('',*,*,#4203,.F.);
#5498=ORIENTED_EDGE('',*,*,#4208,.F.);
#5499=ORIENTED_EDGE('',*,*,#4209,.T.);
#5500=ORIENTED_EDGE('',*,*,#4210,.T.);
#5501=ORIENTED_EDGE('',*,*,#4206,.F.);
#5502=ORIENTED_EDGE('',*,*,#4211,.F.);
#5503=ORIENTED_EDGE('',*,*,#4212,.F.);
#5504=ORIENTED_EDGE('',*,*,#4213,.F.);
#5505=ORIENTED_EDGE('',*,*,#4214,.F.);
#5506=ORIENTED_EDGE('',*,*,#4215,.T.);
#5507=ORIENTED_EDGE('',*,*,#4216,.T.);
#5508=ORIENTED_EDGE('',*,*,#4217,.T.);
#5509=ORIENTED_EDGE('',*,*,#4218,.T.);
#5510=ORIENTED_EDGE('',*,*,#4219,.T.);
#5511=ORIENTED_EDGE('',*,*,#4220,.T.);
#5512=ORIENTED_EDGE('',*,*,#4219,.F.);
#5513=ORIENTED_EDGE('',*,*,#4221,.T.);
#5514=ORIENTED_EDGE('',*,*,#4222,.T.);
#5515=ORIENTED_EDGE('',*,*,#4223,.T.);
#5516=ORIENTED_EDGE('',*,*,#4224,.T.);
#5517=ORIENTED_EDGE('',*,*,#4216,.F.);
#5518=ORIENTED_EDGE('',*,*,#4225,.T.);
#5519=ORIENTED_EDGE('',*,*,#4226,.T.);
#5520=ORIENTED_EDGE('',*,*,#4227,.T.);
#5521=ORIENTED_EDGE('',*,*,#4223,.F.);
#5522=ORIENTED_EDGE('',*,*,#4228,.T.);
#5523=ORIENTED_EDGE('',*,*,#4229,.T.);
#5524=ORIENTED_EDGE('',*,*,#4230,.T.);
#5525=ORIENTED_EDGE('',*,*,#4226,.F.);
#5526=ORIENTED_EDGE('',*,*,#4231,.T.);
#5527=ORIENTED_EDGE('',*,*,#4232,.T.);
#5528=ORIENTED_EDGE('',*,*,#4233,.T.);
#5529=ORIENTED_EDGE('',*,*,#4229,.F.);
#5530=ORIENTED_EDGE('',*,*,#4234,.T.);
#5531=ORIENTED_EDGE('',*,*,#4235,.T.);
#5532=ORIENTED_EDGE('',*,*,#4236,.T.);
#5533=ORIENTED_EDGE('',*,*,#4232,.F.);
#5534=ORIENTED_EDGE('',*,*,#4237,.T.);
#5535=ORIENTED_EDGE('',*,*,#4238,.T.);
#5536=ORIENTED_EDGE('',*,*,#4239,.T.);
#5537=ORIENTED_EDGE('',*,*,#4235,.F.);
#5538=ORIENTED_EDGE('',*,*,#4240,.T.);
#5539=ORIENTED_EDGE('',*,*,#4241,.T.);
#5540=ORIENTED_EDGE('',*,*,#4242,.T.);
#5541=ORIENTED_EDGE('',*,*,#4238,.F.);
#5542=ORIENTED_EDGE('',*,*,#4243,.T.);
#5543=ORIENTED_EDGE('',*,*,#4244,.T.);
#5544=ORIENTED_EDGE('',*,*,#4245,.T.);
#5545=ORIENTED_EDGE('',*,*,#4241,.F.);
#5546=ORIENTED_EDGE('',*,*,#4246,.T.);
#5547=ORIENTED_EDGE('',*,*,#4247,.T.);
#5548=ORIENTED_EDGE('',*,*,#4248,.T.);
#5549=ORIENTED_EDGE('',*,*,#4244,.F.);
#5550=ORIENTED_EDGE('',*,*,#4249,.T.);
#5551=ORIENTED_EDGE('',*,*,#4250,.T.);
#5552=ORIENTED_EDGE('',*,*,#4251,.T.);
#5553=ORIENTED_EDGE('',*,*,#4247,.F.);
#5554=ORIENTED_EDGE('',*,*,#4252,.T.);
#5555=ORIENTED_EDGE('',*,*,#4253,.T.);
#5556=ORIENTED_EDGE('',*,*,#4254,.T.);
#5557=ORIENTED_EDGE('',*,*,#4250,.F.);
#5558=ORIENTED_EDGE('',*,*,#4255,.T.);
#5559=ORIENTED_EDGE('',*,*,#4256,.T.);
#5560=ORIENTED_EDGE('',*,*,#4257,.T.);
#5561=ORIENTED_EDGE('',*,*,#4253,.F.);
#5562=ORIENTED_EDGE('',*,*,#4258,.T.);
#5563=ORIENTED_EDGE('',*,*,#4259,.T.);
#5564=ORIENTED_EDGE('',*,*,#4260,.T.);
#5565=ORIENTED_EDGE('',*,*,#4256,.F.);
#5566=ORIENTED_EDGE('',*,*,#4261,.T.);
#5567=ORIENTED_EDGE('',*,*,#4262,.T.);
#5568=ORIENTED_EDGE('',*,*,#4263,.T.);
#5569=ORIENTED_EDGE('',*,*,#4259,.F.);
#5570=ORIENTED_EDGE('',*,*,#4264,.T.);
#5571=ORIENTED_EDGE('',*,*,#4265,.T.);
#5572=ORIENTED_EDGE('',*,*,#4266,.T.);
#5573=ORIENTED_EDGE('',*,*,#4262,.F.);
#5574=ORIENTED_EDGE('',*,*,#4267,.T.);
#5575=ORIENTED_EDGE('',*,*,#4268,.F.);
#5576=ORIENTED_EDGE('',*,*,#4269,.T.);
#5577=ORIENTED_EDGE('',*,*,#4270,.F.);
#5578=ORIENTED_EDGE('',*,*,#4271,.T.);
#5579=ORIENTED_EDGE('',*,*,#4272,.T.);
#5580=ORIENTED_EDGE('',*,*,#4273,.T.);
#5581=ORIENTED_EDGE('',*,*,#4274,.F.);
#5582=ORIENTED_EDGE('',*,*,#4275,.F.);
#5583=ORIENTED_EDGE('',*,*,#4276,.T.);
#5584=ORIENTED_EDGE('',*,*,#4277,.T.);
#5585=ORIENTED_EDGE('',*,*,#4272,.F.);
#5586=ORIENTED_EDGE('',*,*,#4278,.F.);
#5587=ORIENTED_EDGE('',*,*,#4279,.T.);
#5588=ORIENTED_EDGE('',*,*,#4280,.T.);
#5589=ORIENTED_EDGE('',*,*,#4276,.F.);
#5590=ORIENTED_EDGE('',*,*,#4281,.F.);
#5591=ORIENTED_EDGE('',*,*,#4282,.T.);
#5592=ORIENTED_EDGE('',*,*,#4283,.T.);
#5593=ORIENTED_EDGE('',*,*,#4279,.F.);
#5594=ORIENTED_EDGE('',*,*,#4284,.F.);
#5595=ORIENTED_EDGE('',*,*,#4285,.T.);
#5596=ORIENTED_EDGE('',*,*,#4286,.T.);
#5597=ORIENTED_EDGE('',*,*,#4282,.F.);
#5598=ORIENTED_EDGE('',*,*,#4287,.F.);
#5599=ORIENTED_EDGE('',*,*,#4288,.T.);
#5600=ORIENTED_EDGE('',*,*,#4289,.T.);
#5601=ORIENTED_EDGE('',*,*,#4285,.F.);
#5602=ORIENTED_EDGE('',*,*,#4290,.F.);
#5603=ORIENTED_EDGE('',*,*,#4291,.T.);
#5604=ORIENTED_EDGE('',*,*,#4292,.T.);
#5605=ORIENTED_EDGE('',*,*,#4288,.F.);
#5606=ORIENTED_EDGE('',*,*,#4293,.F.);
#5607=ORIENTED_EDGE('',*,*,#4294,.T.);
#5608=ORIENTED_EDGE('',*,*,#4295,.T.);
#5609=ORIENTED_EDGE('',*,*,#4291,.F.);
#5610=ORIENTED_EDGE('',*,*,#4296,.F.);
#5611=ORIENTED_EDGE('',*,*,#4297,.T.);
#5612=ORIENTED_EDGE('',*,*,#4298,.T.);
#5613=ORIENTED_EDGE('',*,*,#4294,.F.);
#5614=ORIENTED_EDGE('',*,*,#4299,.F.);
#5615=ORIENTED_EDGE('',*,*,#4300,.T.);
#5616=ORIENTED_EDGE('',*,*,#4301,.T.);
#5617=ORIENTED_EDGE('',*,*,#4297,.F.);
#5618=ORIENTED_EDGE('',*,*,#4302,.F.);
#5619=ORIENTED_EDGE('',*,*,#4303,.T.);
#5620=ORIENTED_EDGE('',*,*,#4304,.T.);
#5621=ORIENTED_EDGE('',*,*,#4300,.F.);
#5622=ORIENTED_EDGE('',*,*,#4305,.F.);
#5623=ORIENTED_EDGE('',*,*,#4306,.T.);
#5624=ORIENTED_EDGE('',*,*,#4307,.T.);
#5625=ORIENTED_EDGE('',*,*,#4303,.F.);
#5626=ORIENTED_EDGE('',*,*,#4308,.F.);
#5627=ORIENTED_EDGE('',*,*,#4309,.T.);
#5628=ORIENTED_EDGE('',*,*,#4310,.T.);
#5629=ORIENTED_EDGE('',*,*,#4306,.F.);
#5630=ORIENTED_EDGE('',*,*,#4311,.F.);
#5631=ORIENTED_EDGE('',*,*,#4312,.T.);
#5632=ORIENTED_EDGE('',*,*,#4313,.T.);
#5633=ORIENTED_EDGE('',*,*,#4309,.F.);
#5634=ORIENTED_EDGE('',*,*,#4314,.F.);
#5635=ORIENTED_EDGE('',*,*,#4315,.T.);
#5636=ORIENTED_EDGE('',*,*,#4316,.T.);
#5637=ORIENTED_EDGE('',*,*,#4312,.F.);
#5638=ORIENTED_EDGE('',*,*,#4317,.F.);
#5639=ORIENTED_EDGE('',*,*,#4318,.T.);
#5640=ORIENTED_EDGE('',*,*,#4319,.T.);
#5641=ORIENTED_EDGE('',*,*,#4315,.F.);
#5642=ORIENTED_EDGE('',*,*,#4320,.F.);
#5643=ORIENTED_EDGE('',*,*,#4321,.F.);
#5644=ORIENTED_EDGE('',*,*,#4322,.F.);
#5645=ORIENTED_EDGE('',*,*,#4323,.F.);
#5646=ORIENTED_EDGE('',*,*,#4324,.T.);
#5647=ORIENTED_EDGE('',*,*,#4325,.T.);
#5648=ORIENTED_EDGE('',*,*,#4326,.T.);
#5649=ORIENTED_EDGE('',*,*,#4327,.T.);
#5650=ORIENTED_EDGE('',*,*,#4328,.T.);
#5651=ORIENTED_EDGE('',*,*,#4329,.T.);
#5652=ORIENTED_EDGE('',*,*,#4328,.F.);
#5653=ORIENTED_EDGE('',*,*,#4330,.T.);
#5654=ORIENTED_EDGE('',*,*,#4331,.T.);
#5655=ORIENTED_EDGE('',*,*,#4332,.T.);
#5656=ORIENTED_EDGE('',*,*,#4333,.T.);
#5657=ORIENTED_EDGE('',*,*,#4325,.F.);
#5658=ORIENTED_EDGE('',*,*,#4334,.T.);
#5659=ORIENTED_EDGE('',*,*,#4335,.T.);
#5660=ORIENTED_EDGE('',*,*,#4336,.T.);
#5661=ORIENTED_EDGE('',*,*,#4332,.F.);
#5662=ORIENTED_EDGE('',*,*,#4337,.T.);
#5663=ORIENTED_EDGE('',*,*,#4338,.T.);
#5664=ORIENTED_EDGE('',*,*,#4339,.T.);
#5665=ORIENTED_EDGE('',*,*,#4335,.F.);
#5666=ORIENTED_EDGE('',*,*,#4340,.T.);
#5667=ORIENTED_EDGE('',*,*,#4341,.T.);
#5668=ORIENTED_EDGE('',*,*,#4342,.T.);
#5669=ORIENTED_EDGE('',*,*,#4338,.F.);
#5670=ORIENTED_EDGE('',*,*,#4343,.T.);
#5671=ORIENTED_EDGE('',*,*,#4344,.T.);
#5672=ORIENTED_EDGE('',*,*,#4345,.T.);
#5673=ORIENTED_EDGE('',*,*,#4341,.F.);
#5674=ORIENTED_EDGE('',*,*,#4346,.T.);
#5675=ORIENTED_EDGE('',*,*,#4347,.T.);
#5676=ORIENTED_EDGE('',*,*,#4348,.T.);
#5677=ORIENTED_EDGE('',*,*,#4344,.F.);
#5678=ORIENTED_EDGE('',*,*,#4349,.T.);
#5679=ORIENTED_EDGE('',*,*,#4350,.T.);
#5680=ORIENTED_EDGE('',*,*,#4351,.T.);
#5681=ORIENTED_EDGE('',*,*,#4347,.F.);
#5682=ORIENTED_EDGE('',*,*,#4352,.T.);
#5683=ORIENTED_EDGE('',*,*,#4353,.T.);
#5684=ORIENTED_EDGE('',*,*,#4354,.T.);
#5685=ORIENTED_EDGE('',*,*,#4350,.F.);
#5686=ORIENTED_EDGE('',*,*,#4355,.T.);
#5687=ORIENTED_EDGE('',*,*,#4356,.T.);
#5688=ORIENTED_EDGE('',*,*,#4357,.T.);
#5689=ORIENTED_EDGE('',*,*,#4353,.F.);
#5690=ORIENTED_EDGE('',*,*,#4358,.T.);
#5691=ORIENTED_EDGE('',*,*,#4359,.T.);
#5692=ORIENTED_EDGE('',*,*,#4360,.T.);
#5693=ORIENTED_EDGE('',*,*,#4356,.F.);
#5694=ORIENTED_EDGE('',*,*,#4361,.T.);
#5695=ORIENTED_EDGE('',*,*,#4362,.T.);
#5696=ORIENTED_EDGE('',*,*,#4363,.T.);
#5697=ORIENTED_EDGE('',*,*,#4359,.F.);
#5698=ORIENTED_EDGE('',*,*,#4364,.T.);
#5699=ORIENTED_EDGE('',*,*,#4365,.T.);
#5700=ORIENTED_EDGE('',*,*,#4366,.T.);
#5701=ORIENTED_EDGE('',*,*,#4362,.F.);
#5702=ORIENTED_EDGE('',*,*,#4367,.T.);
#5703=ORIENTED_EDGE('',*,*,#4368,.T.);
#5704=ORIENTED_EDGE('',*,*,#4369,.T.);
#5705=ORIENTED_EDGE('',*,*,#4365,.F.);
#5706=ORIENTED_EDGE('',*,*,#4370,.T.);
#5707=ORIENTED_EDGE('',*,*,#4371,.T.);
#5708=ORIENTED_EDGE('',*,*,#4372,.T.);
#5709=ORIENTED_EDGE('',*,*,#4368,.F.);
#5710=ORIENTED_EDGE('',*,*,#4373,.T.);
#5711=ORIENTED_EDGE('',*,*,#4374,.T.);
#5712=ORIENTED_EDGE('',*,*,#4375,.T.);
#5713=ORIENTED_EDGE('',*,*,#4371,.F.);
#5714=ORIENTED_EDGE('',*,*,#4376,.T.);
#5715=ORIENTED_EDGE('',*,*,#4377,.F.);
#5716=ORIENTED_EDGE('',*,*,#4378,.T.);
#5717=ORIENTED_EDGE('',*,*,#4379,.F.);
#5718=ORIENTED_EDGE('',*,*,#4380,.T.);
#5719=ORIENTED_EDGE('',*,*,#4381,.T.);
#5720=ORIENTED_EDGE('',*,*,#4382,.T.);
#5721=ORIENTED_EDGE('',*,*,#4383,.F.);
#5722=ORIENTED_EDGE('',*,*,#4384,.F.);
#5723=ORIENTED_EDGE('',*,*,#4385,.T.);
#5724=ORIENTED_EDGE('',*,*,#4386,.T.);
#5725=ORIENTED_EDGE('',*,*,#4381,.F.);
#5726=ORIENTED_EDGE('',*,*,#4387,.F.);
#5727=ORIENTED_EDGE('',*,*,#4388,.T.);
#5728=ORIENTED_EDGE('',*,*,#4389,.T.);
#5729=ORIENTED_EDGE('',*,*,#4385,.F.);
#5730=ORIENTED_EDGE('',*,*,#4390,.F.);
#5731=ORIENTED_EDGE('',*,*,#4391,.T.);
#5732=ORIENTED_EDGE('',*,*,#4392,.T.);
#5733=ORIENTED_EDGE('',*,*,#4388,.F.);
#5734=ORIENTED_EDGE('',*,*,#4393,.F.);
#5735=ORIENTED_EDGE('',*,*,#4394,.T.);
#5736=ORIENTED_EDGE('',*,*,#4395,.T.);
#5737=ORIENTED_EDGE('',*,*,#4391,.F.);
#5738=ORIENTED_EDGE('',*,*,#4396,.F.);
#5739=ORIENTED_EDGE('',*,*,#4397,.T.);
#5740=ORIENTED_EDGE('',*,*,#4398,.T.);
#5741=ORIENTED_EDGE('',*,*,#4394,.F.);
#5742=ORIENTED_EDGE('',*,*,#4399,.F.);
#5743=ORIENTED_EDGE('',*,*,#4400,.T.);
#5744=ORIENTED_EDGE('',*,*,#4401,.T.);
#5745=ORIENTED_EDGE('',*,*,#4397,.F.);
#5746=ORIENTED_EDGE('',*,*,#4402,.F.);
#5747=ORIENTED_EDGE('',*,*,#4403,.T.);
#5748=ORIENTED_EDGE('',*,*,#4404,.T.);
#5749=ORIENTED_EDGE('',*,*,#4400,.F.);
#5750=ORIENTED_EDGE('',*,*,#4405,.F.);
#5751=ORIENTED_EDGE('',*,*,#4406,.T.);
#5752=ORIENTED_EDGE('',*,*,#4407,.T.);
#5753=ORIENTED_EDGE('',*,*,#4403,.F.);
#5754=ORIENTED_EDGE('',*,*,#4408,.F.);
#5755=ORIENTED_EDGE('',*,*,#4409,.T.);
#5756=ORIENTED_EDGE('',*,*,#4410,.T.);
#5757=ORIENTED_EDGE('',*,*,#4406,.F.);
#5758=ORIENTED_EDGE('',*,*,#4411,.F.);
#5759=ORIENTED_EDGE('',*,*,#4412,.T.);
#5760=ORIENTED_EDGE('',*,*,#4413,.T.);
#5761=ORIENTED_EDGE('',*,*,#4409,.F.);
#5762=ORIENTED_EDGE('',*,*,#4414,.F.);
#5763=ORIENTED_EDGE('',*,*,#4415,.T.);
#5764=ORIENTED_EDGE('',*,*,#4416,.T.);
#5765=ORIENTED_EDGE('',*,*,#4412,.F.);
#5766=ORIENTED_EDGE('',*,*,#4417,.F.);
#5767=ORIENTED_EDGE('',*,*,#4418,.T.);
#5768=ORIENTED_EDGE('',*,*,#4419,.T.);
#5769=ORIENTED_EDGE('',*,*,#4415,.F.);
#5770=ORIENTED_EDGE('',*,*,#4420,.F.);
#5771=ORIENTED_EDGE('',*,*,#4421,.T.);
#5772=ORIENTED_EDGE('',*,*,#4422,.T.);
#5773=ORIENTED_EDGE('',*,*,#4418,.F.);
#5774=ORIENTED_EDGE('',*,*,#4423,.F.);
#5775=ORIENTED_EDGE('',*,*,#4424,.T.);
#5776=ORIENTED_EDGE('',*,*,#4425,.T.);
#5777=ORIENTED_EDGE('',*,*,#4421,.F.);
#5778=ORIENTED_EDGE('',*,*,#4426,.F.);
#5779=ORIENTED_EDGE('',*,*,#4427,.T.);
#5780=ORIENTED_EDGE('',*,*,#4428,.T.);
#5781=ORIENTED_EDGE('',*,*,#4424,.F.);
#5782=ORIENTED_EDGE('',*,*,#4429,.F.);
#5783=ORIENTED_EDGE('',*,*,#4430,.F.);
#5784=ORIENTED_EDGE('',*,*,#4431,.F.);
#5785=ORIENTED_EDGE('',*,*,#4432,.F.);
#5786=ORIENTED_EDGE('',*,*,#4433,.T.);
#5787=ORIENTED_EDGE('',*,*,#4434,.T.);
#5788=ORIENTED_EDGE('',*,*,#4435,.T.);
#5789=ORIENTED_EDGE('',*,*,#4436,.T.);
#5790=ORIENTED_EDGE('',*,*,#4437,.T.);
#5791=ORIENTED_EDGE('',*,*,#4438,.T.);
#5792=ORIENTED_EDGE('',*,*,#4437,.F.);
#5793=ORIENTED_EDGE('',*,*,#4439,.T.);
#5794=ORIENTED_EDGE('',*,*,#4440,.T.);
#5795=ORIENTED_EDGE('',*,*,#4441,.T.);
#5796=ORIENTED_EDGE('',*,*,#4442,.T.);
#5797=ORIENTED_EDGE('',*,*,#4434,.F.);
#5798=ORIENTED_EDGE('',*,*,#4443,.T.);
#5799=ORIENTED_EDGE('',*,*,#4444,.T.);
#5800=ORIENTED_EDGE('',*,*,#4445,.T.);
#5801=ORIENTED_EDGE('',*,*,#4441,.F.);
#5802=ORIENTED_EDGE('',*,*,#4446,.T.);
#5803=ORIENTED_EDGE('',*,*,#4447,.T.);
#5804=ORIENTED_EDGE('',*,*,#4448,.T.);
#5805=ORIENTED_EDGE('',*,*,#4444,.F.);
#5806=ORIENTED_EDGE('',*,*,#4449,.T.);
#5807=ORIENTED_EDGE('',*,*,#4450,.T.);
#5808=ORIENTED_EDGE('',*,*,#4451,.T.);
#5809=ORIENTED_EDGE('',*,*,#4447,.F.);
#5810=ORIENTED_EDGE('',*,*,#4452,.T.);
#5811=ORIENTED_EDGE('',*,*,#4453,.T.);
#5812=ORIENTED_EDGE('',*,*,#4454,.T.);
#5813=ORIENTED_EDGE('',*,*,#4450,.F.);
#5814=ORIENTED_EDGE('',*,*,#4455,.T.);
#5815=ORIENTED_EDGE('',*,*,#4456,.T.);
#5816=ORIENTED_EDGE('',*,*,#4457,.T.);
#5817=ORIENTED_EDGE('',*,*,#4453,.F.);
#5818=ORIENTED_EDGE('',*,*,#4458,.T.);
#5819=ORIENTED_EDGE('',*,*,#4459,.T.);
#5820=ORIENTED_EDGE('',*,*,#4460,.T.);
#5821=ORIENTED_EDGE('',*,*,#4456,.F.);
#5822=ORIENTED_EDGE('',*,*,#4461,.T.);
#5823=ORIENTED_EDGE('',*,*,#4462,.T.);
#5824=ORIENTED_EDGE('',*,*,#4463,.T.);
#5825=ORIENTED_EDGE('',*,*,#4459,.F.);
#5826=ORIENTED_EDGE('',*,*,#4464,.T.);
#5827=ORIENTED_EDGE('',*,*,#4465,.T.);
#5828=ORIENTED_EDGE('',*,*,#4466,.T.);
#5829=ORIENTED_EDGE('',*,*,#4462,.F.);
#5830=ORIENTED_EDGE('',*,*,#4467,.T.);
#5831=ORIENTED_EDGE('',*,*,#4468,.T.);
#5832=ORIENTED_EDGE('',*,*,#4469,.T.);
#5833=ORIENTED_EDGE('',*,*,#4465,.F.);
#5834=ORIENTED_EDGE('',*,*,#4470,.T.);
#5835=ORIENTED_EDGE('',*,*,#4471,.T.);
#5836=ORIENTED_EDGE('',*,*,#4472,.T.);
#5837=ORIENTED_EDGE('',*,*,#4468,.F.);
#5838=ORIENTED_EDGE('',*,*,#4473,.T.);
#5839=ORIENTED_EDGE('',*,*,#4474,.T.);
#5840=ORIENTED_EDGE('',*,*,#4475,.T.);
#5841=ORIENTED_EDGE('',*,*,#4471,.F.);
#5842=ORIENTED_EDGE('',*,*,#4476,.T.);
#5843=ORIENTED_EDGE('',*,*,#4477,.T.);
#5844=ORIENTED_EDGE('',*,*,#4478,.T.);
#5845=ORIENTED_EDGE('',*,*,#4474,.F.);
#5846=ORIENTED_EDGE('',*,*,#4479,.T.);
#5847=ORIENTED_EDGE('',*,*,#4480,.T.);
#5848=ORIENTED_EDGE('',*,*,#4481,.T.);
#5849=ORIENTED_EDGE('',*,*,#4477,.F.);
#5850=ORIENTED_EDGE('',*,*,#4482,.T.);
#5851=ORIENTED_EDGE('',*,*,#4483,.T.);
#5852=ORIENTED_EDGE('',*,*,#4484,.T.);
#5853=ORIENTED_EDGE('',*,*,#4480,.F.);
#5854=ORIENTED_EDGE('',*,*,#4485,.T.);
#5855=ORIENTED_EDGE('',*,*,#4486,.F.);
#5856=ORIENTED_EDGE('',*,*,#4487,.T.);
#5857=ORIENTED_EDGE('',*,*,#4488,.F.);
#5858=ORIENTED_EDGE('',*,*,#4489,.T.);
#5859=ORIENTED_EDGE('',*,*,#4490,.T.);
#5860=ORIENTED_EDGE('',*,*,#4491,.T.);
#5861=ORIENTED_EDGE('',*,*,#4492,.F.);
#5862=ORIENTED_EDGE('',*,*,#4493,.F.);
#5863=ORIENTED_EDGE('',*,*,#4494,.T.);
#5864=ORIENTED_EDGE('',*,*,#4495,.T.);
#5865=ORIENTED_EDGE('',*,*,#4490,.F.);
#5866=ORIENTED_EDGE('',*,*,#4496,.F.);
#5867=ORIENTED_EDGE('',*,*,#4497,.T.);
#5868=ORIENTED_EDGE('',*,*,#4498,.T.);
#5869=ORIENTED_EDGE('',*,*,#4494,.F.);
#5870=ORIENTED_EDGE('',*,*,#4499,.F.);
#5871=ORIENTED_EDGE('',*,*,#4500,.T.);
#5872=ORIENTED_EDGE('',*,*,#4501,.T.);
#5873=ORIENTED_EDGE('',*,*,#4497,.F.);
#5874=ORIENTED_EDGE('',*,*,#4502,.F.);
#5875=ORIENTED_EDGE('',*,*,#4503,.T.);
#5876=ORIENTED_EDGE('',*,*,#4504,.T.);
#5877=ORIENTED_EDGE('',*,*,#4500,.F.);
#5878=ORIENTED_EDGE('',*,*,#4505,.F.);
#5879=ORIENTED_EDGE('',*,*,#4506,.T.);
#5880=ORIENTED_EDGE('',*,*,#4507,.T.);
#5881=ORIENTED_EDGE('',*,*,#4503,.F.);
#5882=ORIENTED_EDGE('',*,*,#4508,.F.);
#5883=ORIENTED_EDGE('',*,*,#4509,.T.);
#5884=ORIENTED_EDGE('',*,*,#4510,.T.);
#5885=ORIENTED_EDGE('',*,*,#4506,.F.);
#5886=ORIENTED_EDGE('',*,*,#4511,.F.);
#5887=ORIENTED_EDGE('',*,*,#4512,.T.);
#5888=ORIENTED_EDGE('',*,*,#4513,.T.);
#5889=ORIENTED_EDGE('',*,*,#4509,.F.);
#5890=ORIENTED_EDGE('',*,*,#4514,.F.);
#5891=ORIENTED_EDGE('',*,*,#4515,.T.);
#5892=ORIENTED_EDGE('',*,*,#4516,.T.);
#5893=ORIENTED_EDGE('',*,*,#4512,.F.);
#5894=ORIENTED_EDGE('',*,*,#4517,.F.);
#5895=ORIENTED_EDGE('',*,*,#4518,.T.);
#5896=ORIENTED_EDGE('',*,*,#4519,.T.);
#5897=ORIENTED_EDGE('',*,*,#4515,.F.);
#5898=ORIENTED_EDGE('',*,*,#4520,.F.);
#5899=ORIENTED_EDGE('',*,*,#4521,.T.);
#5900=ORIENTED_EDGE('',*,*,#4522,.T.);
#5901=ORIENTED_EDGE('',*,*,#4518,.F.);
#5902=ORIENTED_EDGE('',*,*,#4523,.F.);
#5903=ORIENTED_EDGE('',*,*,#4524,.T.);
#5904=ORIENTED_EDGE('',*,*,#4525,.T.);
#5905=ORIENTED_EDGE('',*,*,#4521,.F.);
#5906=ORIENTED_EDGE('',*,*,#4526,.F.);
#5907=ORIENTED_EDGE('',*,*,#4527,.T.);
#5908=ORIENTED_EDGE('',*,*,#4528,.T.);
#5909=ORIENTED_EDGE('',*,*,#4524,.F.);
#5910=ORIENTED_EDGE('',*,*,#4529,.F.);
#5911=ORIENTED_EDGE('',*,*,#4530,.T.);
#5912=ORIENTED_EDGE('',*,*,#4531,.T.);
#5913=ORIENTED_EDGE('',*,*,#4527,.F.);
#5914=ORIENTED_EDGE('',*,*,#4532,.F.);
#5915=ORIENTED_EDGE('',*,*,#4533,.T.);
#5916=ORIENTED_EDGE('',*,*,#4534,.T.);
#5917=ORIENTED_EDGE('',*,*,#4530,.F.);
#5918=ORIENTED_EDGE('',*,*,#4535,.F.);
#5919=ORIENTED_EDGE('',*,*,#4536,.T.);
#5920=ORIENTED_EDGE('',*,*,#4537,.T.);
#5921=ORIENTED_EDGE('',*,*,#4533,.F.);
#5922=ORIENTED_EDGE('',*,*,#4538,.F.);
#5923=ORIENTED_EDGE('',*,*,#4539,.F.);
#5924=ORIENTED_EDGE('',*,*,#4540,.F.);
#5925=ORIENTED_EDGE('',*,*,#4541,.F.);
#5926=ORIENTED_EDGE('',*,*,#4542,.T.);
#5927=ORIENTED_EDGE('',*,*,#4436,.F.);
#5928=ORIENTED_EDGE('',*,*,#4543,.T.);
#5929=ORIENTED_EDGE('',*,*,#4492,.T.);
#5930=ORIENTED_EDGE('',*,*,#4544,.T.);
#5931=ORIENTED_EDGE('',*,*,#4439,.F.);
#5932=ORIENTED_EDGE('',*,*,#4539,.T.);
#5933=ORIENTED_EDGE('',*,*,#4545,.T.);
#5934=ORIENTED_EDGE('',*,*,#4536,.F.);
#5935=ORIENTED_EDGE('',*,*,#4546,.F.);
#5936=ORIENTED_EDGE('',*,*,#4544,.F.);
#5937=ORIENTED_EDGE('',*,*,#4491,.F.);
#5938=ORIENTED_EDGE('',*,*,#4495,.F.);
#5939=ORIENTED_EDGE('',*,*,#4498,.F.);
#5940=ORIENTED_EDGE('',*,*,#4501,.F.);
#5941=ORIENTED_EDGE('',*,*,#4504,.F.);
#5942=ORIENTED_EDGE('',*,*,#4507,.F.);
#5943=ORIENTED_EDGE('',*,*,#4510,.F.);
#5944=ORIENTED_EDGE('',*,*,#4513,.F.);
#5945=ORIENTED_EDGE('',*,*,#4516,.F.);
#5946=ORIENTED_EDGE('',*,*,#4519,.F.);
#5947=ORIENTED_EDGE('',*,*,#4522,.F.);
#5948=ORIENTED_EDGE('',*,*,#4525,.F.);
#5949=ORIENTED_EDGE('',*,*,#4528,.F.);
#5950=ORIENTED_EDGE('',*,*,#4531,.F.);
#5951=ORIENTED_EDGE('',*,*,#4534,.F.);
#5952=ORIENTED_EDGE('',*,*,#4537,.F.);
#5953=ORIENTED_EDGE('',*,*,#4545,.F.);
#5954=ORIENTED_EDGE('',*,*,#4542,.F.);
#5955=ORIENTED_EDGE('',*,*,#4547,.F.);
#5956=ORIENTED_EDGE('',*,*,#4487,.F.);
#5957=ORIENTED_EDGE('',*,*,#4548,.F.);
#5958=ORIENTED_EDGE('',*,*,#4485,.F.);
#5959=ORIENTED_EDGE('',*,*,#4482,.F.);
#5960=ORIENTED_EDGE('',*,*,#4479,.F.);
#5961=ORIENTED_EDGE('',*,*,#4476,.F.);
#5962=ORIENTED_EDGE('',*,*,#4473,.F.);
#5963=ORIENTED_EDGE('',*,*,#4470,.F.);
#5964=ORIENTED_EDGE('',*,*,#4467,.F.);
#5965=ORIENTED_EDGE('',*,*,#4464,.F.);
#5966=ORIENTED_EDGE('',*,*,#4461,.F.);
#5967=ORIENTED_EDGE('',*,*,#4458,.F.);
#5968=ORIENTED_EDGE('',*,*,#4455,.F.);
#5969=ORIENTED_EDGE('',*,*,#4452,.F.);
#5970=ORIENTED_EDGE('',*,*,#4449,.F.);
#5971=ORIENTED_EDGE('',*,*,#4446,.F.);
#5972=ORIENTED_EDGE('',*,*,#4443,.F.);
#5973=ORIENTED_EDGE('',*,*,#4440,.F.);
#5974=ORIENTED_EDGE('',*,*,#4543,.F.);
#5975=ORIENTED_EDGE('',*,*,#4435,.F.);
#5976=ORIENTED_EDGE('',*,*,#4442,.F.);
#5977=ORIENTED_EDGE('',*,*,#4445,.F.);
#5978=ORIENTED_EDGE('',*,*,#4448,.F.);
#5979=ORIENTED_EDGE('',*,*,#4451,.F.);
#5980=ORIENTED_EDGE('',*,*,#4454,.F.);
#5981=ORIENTED_EDGE('',*,*,#4457,.F.);
#5982=ORIENTED_EDGE('',*,*,#4460,.F.);
#5983=ORIENTED_EDGE('',*,*,#4463,.F.);
#5984=ORIENTED_EDGE('',*,*,#4466,.F.);
#5985=ORIENTED_EDGE('',*,*,#4469,.F.);
#5986=ORIENTED_EDGE('',*,*,#4472,.F.);
#5987=ORIENTED_EDGE('',*,*,#4475,.F.);
#5988=ORIENTED_EDGE('',*,*,#4478,.F.);
#5989=ORIENTED_EDGE('',*,*,#4481,.F.);
#5990=ORIENTED_EDGE('',*,*,#4484,.F.);
#5991=ORIENTED_EDGE('',*,*,#4549,.F.);
#5992=ORIENTED_EDGE('',*,*,#4489,.F.);
#5993=ORIENTED_EDGE('',*,*,#4550,.F.);
#5994=ORIENTED_EDGE('',*,*,#4540,.T.);
#5995=ORIENTED_EDGE('',*,*,#4546,.T.);
#5996=ORIENTED_EDGE('',*,*,#4538,.T.);
#5997=ORIENTED_EDGE('',*,*,#4535,.T.);
#5998=ORIENTED_EDGE('',*,*,#4532,.T.);
#5999=ORIENTED_EDGE('',*,*,#4529,.T.);
#6000=ORIENTED_EDGE('',*,*,#4526,.T.);
#6001=ORIENTED_EDGE('',*,*,#4523,.T.);
#6002=ORIENTED_EDGE('',*,*,#4520,.T.);
#6003=ORIENTED_EDGE('',*,*,#4517,.T.);
#6004=ORIENTED_EDGE('',*,*,#4514,.T.);
#6005=ORIENTED_EDGE('',*,*,#4511,.T.);
#6006=ORIENTED_EDGE('',*,*,#4508,.T.);
#6007=ORIENTED_EDGE('',*,*,#4505,.T.);
#6008=ORIENTED_EDGE('',*,*,#4502,.T.);
#6009=ORIENTED_EDGE('',*,*,#4499,.T.);
#6010=ORIENTED_EDGE('',*,*,#4496,.T.);
#6011=ORIENTED_EDGE('',*,*,#4493,.T.);
#6012=ORIENTED_EDGE('',*,*,#4486,.T.);
#6013=ORIENTED_EDGE('',*,*,#4549,.T.);
#6014=ORIENTED_EDGE('',*,*,#4483,.F.);
#6015=ORIENTED_EDGE('',*,*,#4548,.T.);
#6016=ORIENTED_EDGE('',*,*,#4327,.F.);
#6017=ORIENTED_EDGE('',*,*,#4551,.T.);
#6018=ORIENTED_EDGE('',*,*,#4383,.T.);
#6019=ORIENTED_EDGE('',*,*,#4552,.T.);
#6020=ORIENTED_EDGE('',*,*,#4330,.F.);
#6021=ORIENTED_EDGE('',*,*,#4430,.T.);
#6022=ORIENTED_EDGE('',*,*,#4553,.T.);
#6023=ORIENTED_EDGE('',*,*,#4427,.F.);
#6024=ORIENTED_EDGE('',*,*,#4554,.F.);
#6025=ORIENTED_EDGE('',*,*,#4552,.F.);
#6026=ORIENTED_EDGE('',*,*,#4382,.F.);
#6027=ORIENTED_EDGE('',*,*,#4386,.F.);
#6028=ORIENTED_EDGE('',*,*,#4389,.F.);
#6029=ORIENTED_EDGE('',*,*,#4392,.F.);
#6030=ORIENTED_EDGE('',*,*,#4395,.F.);
#6031=ORIENTED_EDGE('',*,*,#4398,.F.);
#6032=ORIENTED_EDGE('',*,*,#4401,.F.);
#6033=ORIENTED_EDGE('',*,*,#4404,.F.);
#6034=ORIENTED_EDGE('',*,*,#4407,.F.);
#6035=ORIENTED_EDGE('',*,*,#4410,.F.);
#6036=ORIENTED_EDGE('',*,*,#4413,.F.);
#6037=ORIENTED_EDGE('',*,*,#4416,.F.);
#6038=ORIENTED_EDGE('',*,*,#4419,.F.);
#6039=ORIENTED_EDGE('',*,*,#4422,.F.);
#6040=ORIENTED_EDGE('',*,*,#4425,.F.);
#6041=ORIENTED_EDGE('',*,*,#4428,.F.);
#6042=ORIENTED_EDGE('',*,*,#4553,.F.);
#6043=ORIENTED_EDGE('',*,*,#4433,.F.);
#6044=ORIENTED_EDGE('',*,*,#4555,.F.);
#6045=ORIENTED_EDGE('',*,*,#4378,.F.);
#6046=ORIENTED_EDGE('',*,*,#4556,.F.);
#6047=ORIENTED_EDGE('',*,*,#4376,.F.);
#6048=ORIENTED_EDGE('',*,*,#4373,.F.);
#6049=ORIENTED_EDGE('',*,*,#4370,.F.);
#6050=ORIENTED_EDGE('',*,*,#4367,.F.);
#6051=ORIENTED_EDGE('',*,*,#4364,.F.);
#6052=ORIENTED_EDGE('',*,*,#4361,.F.);
#6053=ORIENTED_EDGE('',*,*,#4358,.F.);
#6054=ORIENTED_EDGE('',*,*,#4355,.F.);
#6055=ORIENTED_EDGE('',*,*,#4352,.F.);
#6056=ORIENTED_EDGE('',*,*,#4349,.F.);
#6057=ORIENTED_EDGE('',*,*,#4346,.F.);
#6058=ORIENTED_EDGE('',*,*,#4343,.F.);
#6059=ORIENTED_EDGE('',*,*,#4340,.F.);
#6060=ORIENTED_EDGE('',*,*,#4337,.F.);
#6061=ORIENTED_EDGE('',*,*,#4334,.F.);
#6062=ORIENTED_EDGE('',*,*,#4331,.F.);
#6063=ORIENTED_EDGE('',*,*,#4551,.F.);
#6064=ORIENTED_EDGE('',*,*,#4326,.F.);
#6065=ORIENTED_EDGE('',*,*,#4333,.F.);
#6066=ORIENTED_EDGE('',*,*,#4336,.F.);
#6067=ORIENTED_EDGE('',*,*,#4339,.F.);
#6068=ORIENTED_EDGE('',*,*,#4342,.F.);
#6069=ORIENTED_EDGE('',*,*,#4345,.F.);
#6070=ORIENTED_EDGE('',*,*,#4348,.F.);
#6071=ORIENTED_EDGE('',*,*,#4351,.F.);
#6072=ORIENTED_EDGE('',*,*,#4354,.F.);
#6073=ORIENTED_EDGE('',*,*,#4357,.F.);
#6074=ORIENTED_EDGE('',*,*,#4360,.F.);
#6075=ORIENTED_EDGE('',*,*,#4363,.F.);
#6076=ORIENTED_EDGE('',*,*,#4366,.F.);
#6077=ORIENTED_EDGE('',*,*,#4369,.F.);
#6078=ORIENTED_EDGE('',*,*,#4372,.F.);
#6079=ORIENTED_EDGE('',*,*,#4375,.F.);
#6080=ORIENTED_EDGE('',*,*,#4557,.F.);
#6081=ORIENTED_EDGE('',*,*,#4380,.F.);
#6082=ORIENTED_EDGE('',*,*,#4558,.F.);
#6083=ORIENTED_EDGE('',*,*,#4431,.T.);
#6084=ORIENTED_EDGE('',*,*,#4554,.T.);
#6085=ORIENTED_EDGE('',*,*,#4429,.T.);
#6086=ORIENTED_EDGE('',*,*,#4426,.T.);
#6087=ORIENTED_EDGE('',*,*,#4423,.T.);
#6088=ORIENTED_EDGE('',*,*,#4420,.T.);
#6089=ORIENTED_EDGE('',*,*,#4417,.T.);
#6090=ORIENTED_EDGE('',*,*,#4414,.T.);
#6091=ORIENTED_EDGE('',*,*,#4411,.T.);
#6092=ORIENTED_EDGE('',*,*,#4408,.T.);
#6093=ORIENTED_EDGE('',*,*,#4405,.T.);
#6094=ORIENTED_EDGE('',*,*,#4402,.T.);
#6095=ORIENTED_EDGE('',*,*,#4399,.T.);
#6096=ORIENTED_EDGE('',*,*,#4396,.T.);
#6097=ORIENTED_EDGE('',*,*,#4393,.T.);
#6098=ORIENTED_EDGE('',*,*,#4390,.T.);
#6099=ORIENTED_EDGE('',*,*,#4387,.T.);
#6100=ORIENTED_EDGE('',*,*,#4384,.T.);
#6101=ORIENTED_EDGE('',*,*,#4377,.T.);
#6102=ORIENTED_EDGE('',*,*,#4557,.T.);
#6103=ORIENTED_EDGE('',*,*,#4374,.F.);
#6104=ORIENTED_EDGE('',*,*,#4556,.T.);
#6105=ORIENTED_EDGE('',*,*,#4218,.F.);
#6106=ORIENTED_EDGE('',*,*,#4559,.T.);
#6107=ORIENTED_EDGE('',*,*,#4274,.T.);
#6108=ORIENTED_EDGE('',*,*,#4560,.T.);
#6109=ORIENTED_EDGE('',*,*,#4221,.F.);
#6110=ORIENTED_EDGE('',*,*,#4321,.T.);
#6111=ORIENTED_EDGE('',*,*,#4561,.T.);
#6112=ORIENTED_EDGE('',*,*,#4318,.F.);
#6113=ORIENTED_EDGE('',*,*,#4562,.F.);
#6114=ORIENTED_EDGE('',*,*,#4560,.F.);
#6115=ORIENTED_EDGE('',*,*,#4273,.F.);
#6116=ORIENTED_EDGE('',*,*,#4277,.F.);
#6117=ORIENTED_EDGE('',*,*,#4280,.F.);
#6118=ORIENTED_EDGE('',*,*,#4283,.F.);
#6119=ORIENTED_EDGE('',*,*,#4286,.F.);
#6120=ORIENTED_EDGE('',*,*,#4289,.F.);
#6121=ORIENTED_EDGE('',*,*,#4292,.F.);
#6122=ORIENTED_EDGE('',*,*,#4295,.F.);
#6123=ORIENTED_EDGE('',*,*,#4298,.F.);
#6124=ORIENTED_EDGE('',*,*,#4301,.F.);
#6125=ORIENTED_EDGE('',*,*,#4304,.F.);
#6126=ORIENTED_EDGE('',*,*,#4307,.F.);
#6127=ORIENTED_EDGE('',*,*,#4310,.F.);
#6128=ORIENTED_EDGE('',*,*,#4313,.F.);
#6129=ORIENTED_EDGE('',*,*,#4316,.F.);
#6130=ORIENTED_EDGE('',*,*,#4319,.F.);
#6131=ORIENTED_EDGE('',*,*,#4561,.F.);
#6132=ORIENTED_EDGE('',*,*,#4324,.F.);
#6133=ORIENTED_EDGE('',*,*,#4563,.F.);
#6134=ORIENTED_EDGE('',*,*,#4269,.F.);
#6135=ORIENTED_EDGE('',*,*,#4564,.F.);
#6136=ORIENTED_EDGE('',*,*,#4267,.F.);
#6137=ORIENTED_EDGE('',*,*,#4264,.F.);
#6138=ORIENTED_EDGE('',*,*,#4261,.F.);
#6139=ORIENTED_EDGE('',*,*,#4258,.F.);
#6140=ORIENTED_EDGE('',*,*,#4255,.F.);
#6141=ORIENTED_EDGE('',*,*,#4252,.F.);
#6142=ORIENTED_EDGE('',*,*,#4249,.F.);
#6143=ORIENTED_EDGE('',*,*,#4246,.F.);
#6144=ORIENTED_EDGE('',*,*,#4243,.F.);
#6145=ORIENTED_EDGE('',*,*,#4240,.F.);
#6146=ORIENTED_EDGE('',*,*,#4237,.F.);
#6147=ORIENTED_EDGE('',*,*,#4234,.F.);
#6148=ORIENTED_EDGE('',*,*,#4231,.F.);
#6149=ORIENTED_EDGE('',*,*,#4228,.F.);
#6150=ORIENTED_EDGE('',*,*,#4225,.F.);
#6151=ORIENTED_EDGE('',*,*,#4222,.F.);
#6152=ORIENTED_EDGE('',*,*,#4559,.F.);
#6153=ORIENTED_EDGE('',*,*,#4217,.F.);
#6154=ORIENTED_EDGE('',*,*,#4224,.F.);
#6155=ORIENTED_EDGE('',*,*,#4227,.F.);
#6156=ORIENTED_EDGE('',*,*,#4230,.F.);
#6157=ORIENTED_EDGE('',*,*,#4233,.F.);
#6158=ORIENTED_EDGE('',*,*,#4236,.F.);
#6159=ORIENTED_EDGE('',*,*,#4239,.F.);
#6160=ORIENTED_EDGE('',*,*,#4242,.F.);
#6161=ORIENTED_EDGE('',*,*,#4245,.F.);
#6162=ORIENTED_EDGE('',*,*,#4248,.F.);
#6163=ORIENTED_EDGE('',*,*,#4251,.F.);
#6164=ORIENTED_EDGE('',*,*,#4254,.F.);
#6165=ORIENTED_EDGE('',*,*,#4257,.F.);
#6166=ORIENTED_EDGE('',*,*,#4260,.F.);
#6167=ORIENTED_EDGE('',*,*,#4263,.F.);
#6168=ORIENTED_EDGE('',*,*,#4266,.F.);
#6169=ORIENTED_EDGE('',*,*,#4565,.F.);
#6170=ORIENTED_EDGE('',*,*,#4271,.F.);
#6171=ORIENTED_EDGE('',*,*,#4566,.F.);
#6172=ORIENTED_EDGE('',*,*,#4322,.T.);
#6173=ORIENTED_EDGE('',*,*,#4562,.T.);
#6174=ORIENTED_EDGE('',*,*,#4320,.T.);
#6175=ORIENTED_EDGE('',*,*,#4317,.T.);
#6176=ORIENTED_EDGE('',*,*,#4314,.T.);
#6177=ORIENTED_EDGE('',*,*,#4311,.T.);
#6178=ORIENTED_EDGE('',*,*,#4308,.T.);
#6179=ORIENTED_EDGE('',*,*,#4305,.T.);
#6180=ORIENTED_EDGE('',*,*,#4302,.T.);
#6181=ORIENTED_EDGE('',*,*,#4299,.T.);
#6182=ORIENTED_EDGE('',*,*,#4296,.T.);
#6183=ORIENTED_EDGE('',*,*,#4293,.T.);
#6184=ORIENTED_EDGE('',*,*,#4290,.T.);
#6185=ORIENTED_EDGE('',*,*,#4287,.T.);
#6186=ORIENTED_EDGE('',*,*,#4284,.T.);
#6187=ORIENTED_EDGE('',*,*,#4281,.T.);
#6188=ORIENTED_EDGE('',*,*,#4278,.T.);
#6189=ORIENTED_EDGE('',*,*,#4275,.T.);
#6190=ORIENTED_EDGE('',*,*,#4268,.T.);
#6191=ORIENTED_EDGE('',*,*,#4565,.T.);
#6192=ORIENTED_EDGE('',*,*,#4265,.F.);
#6193=ORIENTED_EDGE('',*,*,#4564,.T.);
#6194=ORIENTED_EDGE('',*,*,#4109,.F.);
#6195=ORIENTED_EDGE('',*,*,#4567,.T.);
#6196=ORIENTED_EDGE('',*,*,#4165,.T.);
#6197=ORIENTED_EDGE('',*,*,#4568,.T.);
#6198=ORIENTED_EDGE('',*,*,#4112,.F.);
#6199=ORIENTED_EDGE('',*,*,#4212,.T.);
#6200=ORIENTED_EDGE('',*,*,#4569,.T.);
#6201=ORIENTED_EDGE('',*,*,#4209,.F.);
#6202=ORIENTED_EDGE('',*,*,#4570,.F.);
#6203=ORIENTED_EDGE('',*,*,#4568,.F.);
#6204=ORIENTED_EDGE('',*,*,#4164,.F.);
#6205=ORIENTED_EDGE('',*,*,#4168,.F.);
#6206=ORIENTED_EDGE('',*,*,#4171,.F.);
#6207=ORIENTED_EDGE('',*,*,#4174,.F.);
#6208=ORIENTED_EDGE('',*,*,#4177,.F.);
#6209=ORIENTED_EDGE('',*,*,#4180,.F.);
#6210=ORIENTED_EDGE('',*,*,#4183,.F.);
#6211=ORIENTED_EDGE('',*,*,#4186,.F.);
#6212=ORIENTED_EDGE('',*,*,#4189,.F.);
#6213=ORIENTED_EDGE('',*,*,#4192,.F.);
#6214=ORIENTED_EDGE('',*,*,#4195,.F.);
#6215=ORIENTED_EDGE('',*,*,#4198,.F.);
#6216=ORIENTED_EDGE('',*,*,#4201,.F.);
#6217=ORIENTED_EDGE('',*,*,#4204,.F.);
#6218=ORIENTED_EDGE('',*,*,#4207,.F.);
#6219=ORIENTED_EDGE('',*,*,#4210,.F.);
#6220=ORIENTED_EDGE('',*,*,#4569,.F.);
#6221=ORIENTED_EDGE('',*,*,#4215,.F.);
#6222=ORIENTED_EDGE('',*,*,#4571,.F.);
#6223=ORIENTED_EDGE('',*,*,#4160,.F.);
#6224=ORIENTED_EDGE('',*,*,#4572,.F.);
#6225=ORIENTED_EDGE('',*,*,#4158,.F.);
#6226=ORIENTED_EDGE('',*,*,#4155,.F.);
#6227=ORIENTED_EDGE('',*,*,#4152,.F.);
#6228=ORIENTED_EDGE('',*,*,#4149,.F.);
#6229=ORIENTED_EDGE('',*,*,#4146,.F.);
#6230=ORIENTED_EDGE('',*,*,#4143,.F.);
#6231=ORIENTED_EDGE('',*,*,#4140,.F.);
#6232=ORIENTED_EDGE('',*,*,#4137,.F.);
#6233=ORIENTED_EDGE('',*,*,#4134,.F.);
#6234=ORIENTED_EDGE('',*,*,#4131,.F.);
#6235=ORIENTED_EDGE('',*,*,#4128,.F.);
#6236=ORIENTED_EDGE('',*,*,#4125,.F.);
#6237=ORIENTED_EDGE('',*,*,#4122,.F.);
#6238=ORIENTED_EDGE('',*,*,#4119,.F.);
#6239=ORIENTED_EDGE('',*,*,#4116,.F.);
#6240=ORIENTED_EDGE('',*,*,#4113,.F.);
#6241=ORIENTED_EDGE('',*,*,#4567,.F.);
#6242=ORIENTED_EDGE('',*,*,#4108,.F.);
#6243=ORIENTED_EDGE('',*,*,#4115,.F.);
#6244=ORIENTED_EDGE('',*,*,#4118,.F.);
#6245=ORIENTED_EDGE('',*,*,#4121,.F.);
#6246=ORIENTED_EDGE('',*,*,#4124,.F.);
#6247=ORIENTED_EDGE('',*,*,#4127,.F.);
#6248=ORIENTED_EDGE('',*,*,#4130,.F.);
#6249=ORIENTED_EDGE('',*,*,#4133,.F.);
#6250=ORIENTED_EDGE('',*,*,#4136,.F.);
#6251=ORIENTED_EDGE('',*,*,#4139,.F.);
#6252=ORIENTED_EDGE('',*,*,#4142,.F.);
#6253=ORIENTED_EDGE('',*,*,#4145,.F.);
#6254=ORIENTED_EDGE('',*,*,#4148,.F.);
#6255=ORIENTED_EDGE('',*,*,#4151,.F.);
#6256=ORIENTED_EDGE('',*,*,#4154,.F.);
#6257=ORIENTED_EDGE('',*,*,#4157,.F.);
#6258=ORIENTED_EDGE('',*,*,#4573,.F.);
#6259=ORIENTED_EDGE('',*,*,#4162,.F.);
#6260=ORIENTED_EDGE('',*,*,#4574,.F.);
#6261=ORIENTED_EDGE('',*,*,#4213,.T.);
#6262=ORIENTED_EDGE('',*,*,#4570,.T.);
#6263=ORIENTED_EDGE('',*,*,#4211,.T.);
#6264=ORIENTED_EDGE('',*,*,#4208,.T.);
#6265=ORIENTED_EDGE('',*,*,#4205,.T.);
#6266=ORIENTED_EDGE('',*,*,#4202,.T.);
#6267=ORIENTED_EDGE('',*,*,#4199,.T.);
#6268=ORIENTED_EDGE('',*,*,#4196,.T.);
#6269=ORIENTED_EDGE('',*,*,#4193,.T.);
#6270=ORIENTED_EDGE('',*,*,#4190,.T.);
#6271=ORIENTED_EDGE('',*,*,#4187,.T.);
#6272=ORIENTED_EDGE('',*,*,#4184,.T.);
#6273=ORIENTED_EDGE('',*,*,#4181,.T.);
#6274=ORIENTED_EDGE('',*,*,#4178,.T.);
#6275=ORIENTED_EDGE('',*,*,#4175,.T.);
#6276=ORIENTED_EDGE('',*,*,#4172,.T.);
#6277=ORIENTED_EDGE('',*,*,#4169,.T.);
#6278=ORIENTED_EDGE('',*,*,#4166,.T.);
#6279=ORIENTED_EDGE('',*,*,#4159,.T.);
#6280=ORIENTED_EDGE('',*,*,#4573,.T.);
#6281=ORIENTED_EDGE('',*,*,#4156,.F.);
#6282=ORIENTED_EDGE('',*,*,#4572,.T.);
#6283=ORIENTED_EDGE('',*,*,#4329,.F.);
#6284=ORIENTED_EDGE('',*,*,#4220,.F.);
#6285=ORIENTED_EDGE('',*,*,#4438,.F.);
#6286=ORIENTED_EDGE('',*,*,#4111,.F.);
#6287=ORIENTED_EDGE('',*,*,#4575,.T.);
#6288=ORIENTED_EDGE('',*,*,#4576,.T.);
#6289=ORIENTED_EDGE('',*,*,#4577,.F.);
#6290=ORIENTED_EDGE('',*,*,#4578,.F.);
#6291=ORIENTED_EDGE('',*,*,#4579,.T.);
#6292=ORIENTED_EDGE('',*,*,#4578,.T.);
#6293=ORIENTED_EDGE('',*,*,#4580,.F.);
#6294=ORIENTED_EDGE('',*,*,#4581,.F.);
#6295=ORIENTED_EDGE('',*,*,#4582,.T.);
#6296=ORIENTED_EDGE('',*,*,#4581,.T.);
#6297=ORIENTED_EDGE('',*,*,#4583,.F.);
#6298=ORIENTED_EDGE('',*,*,#4584,.F.);
#6299=ORIENTED_EDGE('',*,*,#4585,.T.);
#6300=ORIENTED_EDGE('',*,*,#4584,.T.);
#6301=ORIENTED_EDGE('',*,*,#4586,.F.);
#6302=ORIENTED_EDGE('',*,*,#4576,.F.);
#6303=ORIENTED_EDGE('',*,*,#4587,.T.);
#6304=ORIENTED_EDGE('',*,*,#4588,.T.);
#6305=ORIENTED_EDGE('',*,*,#4589,.F.);
#6306=ORIENTED_EDGE('',*,*,#4590,.F.);
#6307=ORIENTED_EDGE('',*,*,#4591,.T.);
#6308=ORIENTED_EDGE('',*,*,#4590,.T.);
#6309=ORIENTED_EDGE('',*,*,#4592,.F.);
#6310=ORIENTED_EDGE('',*,*,#4593,.F.);
#6311=ORIENTED_EDGE('',*,*,#4594,.T.);
#6312=ORIENTED_EDGE('',*,*,#4593,.T.);
#6313=ORIENTED_EDGE('',*,*,#4595,.F.);
#6314=ORIENTED_EDGE('',*,*,#4596,.F.);
#6315=ORIENTED_EDGE('',*,*,#4597,.T.);
#6316=ORIENTED_EDGE('',*,*,#4596,.T.);
#6317=ORIENTED_EDGE('',*,*,#4598,.F.);
#6318=ORIENTED_EDGE('',*,*,#4588,.F.);
#6319=ORIENTED_EDGE('',*,*,#4598,.T.);
#6320=ORIENTED_EDGE('',*,*,#4595,.T.);
#6321=ORIENTED_EDGE('',*,*,#4592,.T.);
#6322=ORIENTED_EDGE('',*,*,#4589,.T.);
#6323=ORIENTED_EDGE('',*,*,#4586,.T.);
#6324=ORIENTED_EDGE('',*,*,#4583,.T.);
#6325=ORIENTED_EDGE('',*,*,#4580,.T.);
#6326=ORIENTED_EDGE('',*,*,#4577,.T.);
#6327=ORIENTED_EDGE('',*,*,#4597,.F.);
#6328=ORIENTED_EDGE('',*,*,#4587,.F.);
#6329=ORIENTED_EDGE('',*,*,#4591,.F.);
#6330=ORIENTED_EDGE('',*,*,#4594,.F.);
#6331=ORIENTED_EDGE('',*,*,#4550,.T.);
#6332=ORIENTED_EDGE('',*,*,#4488,.T.);
#6333=ORIENTED_EDGE('',*,*,#4547,.T.);
#6334=ORIENTED_EDGE('',*,*,#4541,.T.);
#6335=ORIENTED_EDGE('',*,*,#4558,.T.);
#6336=ORIENTED_EDGE('',*,*,#4379,.T.);
#6337=ORIENTED_EDGE('',*,*,#4555,.T.);
#6338=ORIENTED_EDGE('',*,*,#4432,.T.);
#6339=ORIENTED_EDGE('',*,*,#4566,.T.);
#6340=ORIENTED_EDGE('',*,*,#4270,.T.);
#6341=ORIENTED_EDGE('',*,*,#4563,.T.);
#6342=ORIENTED_EDGE('',*,*,#4323,.T.);
#6343=ORIENTED_EDGE('',*,*,#4574,.T.);
#6344=ORIENTED_EDGE('',*,*,#4161,.T.);
#6345=ORIENTED_EDGE('',*,*,#4571,.T.);
#6346=ORIENTED_EDGE('',*,*,#4214,.T.);
#6347=ORIENTED_EDGE('',*,*,#4585,.F.);
#6348=ORIENTED_EDGE('',*,*,#4575,.F.);
#6349=ORIENTED_EDGE('',*,*,#4579,.F.);
#6350=ORIENTED_EDGE('',*,*,#4582,.F.);
#7887=CYLINDRICAL_SURFACE('',#8894,2.5175);
#7888=CYLINDRICAL_SURFACE('',#8898,2.5175);
#7889=CYLINDRICAL_SURFACE('',#8899,2.5175);
#7890=CYLINDRICAL_SURFACE('',#8900,2.5175);
#7891=CYLINDRICAL_SURFACE('',#8901,2.5175);
#7892=CYLINDRICAL_SURFACE('',#8902,2.5175);
#7893=CYLINDRICAL_SURFACE('',#8903,2.5175);
#7894=CYLINDRICAL_SURFACE('',#8904,2.5175);
#7895=CYLINDRICAL_SURFACE('',#8905,2.5175);
#7896=CYLINDRICAL_SURFACE('',#8906,2.5175);
#7897=CYLINDRICAL_SURFACE('',#8907,2.5175);
#7898=CYLINDRICAL_SURFACE('',#8908,2.5175);
#7899=CYLINDRICAL_SURFACE('',#8909,2.5175);
#7900=CYLINDRICAL_SURFACE('',#8910,2.5175);
#7901=CYLINDRICAL_SURFACE('',#8911,2.5175);
#7902=CYLINDRICAL_SURFACE('',#8912,2.5175);
#7903=CYLINDRICAL_SURFACE('',#8913,2.5175);
#7904=CYLINDRICAL_SURFACE('',#8915,3.0735);
#7905=CYLINDRICAL_SURFACE('',#8917,3.0735);
#7906=CYLINDRICAL_SURFACE('',#8918,3.0735);
#7907=CYLINDRICAL_SURFACE('',#8919,3.0735);
#7908=CYLINDRICAL_SURFACE('',#8920,3.0735);
#7909=CYLINDRICAL_SURFACE('',#8921,3.0735);
#7910=CYLINDRICAL_SURFACE('',#8922,3.0735);
#7911=CYLINDRICAL_SURFACE('',#8923,3.0735);
#7912=CYLINDRICAL_SURFACE('',#8924,3.0735);
#7913=CYLINDRICAL_SURFACE('',#8925,3.0735);
#7914=CYLINDRICAL_SURFACE('',#8926,3.0735);
#7915=CYLINDRICAL_SURFACE('',#8927,3.0735);
#7916=CYLINDRICAL_SURFACE('',#8928,3.0735);
#7917=CYLINDRICAL_SURFACE('',#8929,3.0735);
#7918=CYLINDRICAL_SURFACE('',#8930,3.0735);
#7919=CYLINDRICAL_SURFACE('',#8931,3.0735);
#7920=CYLINDRICAL_SURFACE('',#8932,3.0735);
#7921=CYLINDRICAL_SURFACE('',#8934,2.5175);
#7922=CYLINDRICAL_SURFACE('',#8938,2.5175);
#7923=CYLINDRICAL_SURFACE('',#8939,2.5175);
#7924=CYLINDRICAL_SURFACE('',#8940,2.5175);
#7925=CYLINDRICAL_SURFACE('',#8941,2.5175);
#7926=CYLINDRICAL_SURFACE('',#8942,2.5175);
#7927=CYLINDRICAL_SURFACE('',#8943,2.5175);
#7928=CYLINDRICAL_SURFACE('',#8944,2.5175);
#7929=CYLINDRICAL_SURFACE('',#8945,2.5175);
#7930=CYLINDRICAL_SURFACE('',#8946,2.5175);
#7931=CYLINDRICAL_SURFACE('',#8947,2.5175);
#7932=CYLINDRICAL_SURFACE('',#8948,2.5175);
#7933=CYLINDRICAL_SURFACE('',#8949,2.5175);
#7934=CYLINDRICAL_SURFACE('',#8950,2.5175);
#7935=CYLINDRICAL_SURFACE('',#8951,2.5175);
#7936=CYLINDRICAL_SURFACE('',#8952,2.5175);
#7937=CYLINDRICAL_SURFACE('',#8953,2.5175);
#7938=CYLINDRICAL_SURFACE('',#8955,3.0735);
#7939=CYLINDRICAL_SURFACE('',#8957,3.0735);
#7940=CYLINDRICAL_SURFACE('',#8958,3.0735);
#7941=CYLINDRICAL_SURFACE('',#8959,3.0735);
#7942=CYLINDRICAL_SURFACE('',#8960,3.0735);
#7943=CYLINDRICAL_SURFACE('',#8961,3.0735);
#7944=CYLINDRICAL_SURFACE('',#8962,3.0735);
#7945=CYLINDRICAL_SURFACE('',#8963,3.0735);
#7946=CYLINDRICAL_SURFACE('',#8964,3.0735);
#7947=CYLINDRICAL_SURFACE('',#8965,3.0735);
#7948=CYLINDRICAL_SURFACE('',#8966,3.0735);
#7949=CYLINDRICAL_SURFACE('',#8967,3.0735);
#7950=CYLINDRICAL_SURFACE('',#8968,3.0735);
#7951=CYLINDRICAL_SURFACE('',#8969,3.0735);
#7952=CYLINDRICAL_SURFACE('',#8970,3.0735);
#7953=CYLINDRICAL_SURFACE('',#8971,3.0735);
#7954=CYLINDRICAL_SURFACE('',#8972,3.0735);
#7955=CYLINDRICAL_SURFACE('',#8974,2.5175);
#7956=CYLINDRICAL_SURFACE('',#8978,2.5175);
#7957=CYLINDRICAL_SURFACE('',#8979,2.5175);
#7958=CYLINDRICAL_SURFACE('',#8980,2.5175);
#7959=CYLINDRICAL_SURFACE('',#8981,2.5175);
#7960=CYLINDRICAL_SURFACE('',#8982,2.5175);
#7961=CYLINDRICAL_SURFACE('',#8983,2.5175);
#7962=CYLINDRICAL_SURFACE('',#8984,2.5175);
#7963=CYLINDRICAL_SURFACE('',#8985,2.5175);
#7964=CYLINDRICAL_SURFACE('',#8986,2.5175);
#7965=CYLINDRICAL_SURFACE('',#8987,2.5175);
#7966=CYLINDRICAL_SURFACE('',#8988,2.5175);
#7967=CYLINDRICAL_SURFACE('',#8989,2.5175);
#7968=CYLINDRICAL_SURFACE('',#8990,2.5175);
#7969=CYLINDRICAL_SURFACE('',#8991,2.5175);
#7970=CYLINDRICAL_SURFACE('',#8992,2.5175);
#7971=CYLINDRICAL_SURFACE('',#8993,2.5175);
#7972=CYLINDRICAL_SURFACE('',#8995,3.07349999999996);
#7973=CYLINDRICAL_SURFACE('',#8997,3.07349999999996);
#7974=CYLINDRICAL_SURFACE('',#8998,3.07349999999996);
#7975=CYLINDRICAL_SURFACE('',#8999,3.07349999999996);
#7976=CYLINDRICAL_SURFACE('',#9000,3.07349999999996);
#7977=CYLINDRICAL_SURFACE('',#9001,3.07349999999996);
#7978=CYLINDRICAL_SURFACE('',#9002,3.07349999999996);
#7979=CYLINDRICAL_SURFACE('',#9003,3.07349999999996);
#7980=CYLINDRICAL_SURFACE('',#9004,3.07349999999996);
#7981=CYLINDRICAL_SURFACE('',#9005,3.07349999999996);
#7982=CYLINDRICAL_SURFACE('',#9006,3.07349999999996);
#7983=CYLINDRICAL_SURFACE('',#9007,3.07349999999996);
#7984=CYLINDRICAL_SURFACE('',#9008,3.07349999999996);
#7985=CYLINDRICAL_SURFACE('',#9009,3.07349999999996);
#7986=CYLINDRICAL_SURFACE('',#9010,3.07349999999996);
#7987=CYLINDRICAL_SURFACE('',#9011,3.07349999999996);
#7988=CYLINDRICAL_SURFACE('',#9012,3.07349999999996);
#7989=CYLINDRICAL_SURFACE('',#9014,2.5175);
#7990=CYLINDRICAL_SURFACE('',#9018,2.5175);
#7991=CYLINDRICAL_SURFACE('',#9019,2.5175);
#7992=CYLINDRICAL_SURFACE('',#9020,2.5175);
#7993=CYLINDRICAL_SURFACE('',#9021,2.5175);
#7994=CYLINDRICAL_SURFACE('',#9022,2.5175);
#7995=CYLINDRICAL_SURFACE('',#9023,2.5175);
#7996=CYLINDRICAL_SURFACE('',#9024,2.5175);
#7997=CYLINDRICAL_SURFACE('',#9025,2.5175);
#7998=CYLINDRICAL_SURFACE('',#9026,2.5175);
#7999=CYLINDRICAL_SURFACE('',#9027,2.5175);
#8000=CYLINDRICAL_SURFACE('',#9028,2.5175);
#8001=CYLINDRICAL_SURFACE('',#9029,2.5175);
#8002=CYLINDRICAL_SURFACE('',#9030,2.5175);
#8003=CYLINDRICAL_SURFACE('',#9031,2.5175);
#8004=CYLINDRICAL_SURFACE('',#9032,2.5175);
#8005=CYLINDRICAL_SURFACE('',#9033,2.5175);
#8006=CYLINDRICAL_SURFACE('',#9035,3.07350000000003);
#8007=CYLINDRICAL_SURFACE('',#9037,3.07350000000003);
#8008=CYLINDRICAL_SURFACE('',#9038,3.07350000000003);
#8009=CYLINDRICAL_SURFACE('',#9039,3.07350000000003);
#8010=CYLINDRICAL_SURFACE('',#9040,3.07350000000003);
#8011=CYLINDRICAL_SURFACE('',#9041,3.07350000000003);
#8012=CYLINDRICAL_SURFACE('',#9042,3.07350000000003);
#8013=CYLINDRICAL_SURFACE('',#9043,3.07350000000003);
#8014=CYLINDRICAL_SURFACE('',#9044,3.07350000000003);
#8015=CYLINDRICAL_SURFACE('',#9045,3.07350000000003);
#8016=CYLINDRICAL_SURFACE('',#9046,3.07350000000003);
#8017=CYLINDRICAL_SURFACE('',#9047,3.07350000000003);
#8018=CYLINDRICAL_SURFACE('',#9048,3.07350000000003);
#8019=CYLINDRICAL_SURFACE('',#9049,3.07350000000003);
#8020=CYLINDRICAL_SURFACE('',#9050,3.07350000000003);
#8021=CYLINDRICAL_SURFACE('',#9051,3.07350000000003);
#8022=CYLINDRICAL_SURFACE('',#9052,3.07350000000003);
#8023=CYLINDRICAL_SURFACE('',#9055,3.07350000000003);
#8024=CYLINDRICAL_SURFACE('',#9056,2.5175);
#8025=CYLINDRICAL_SURFACE('',#9058,3.07349999999996);
#8026=CYLINDRICAL_SURFACE('',#9059,2.5175);
#8027=CYLINDRICAL_SURFACE('',#9061,3.0735);
#8028=CYLINDRICAL_SURFACE('',#9062,2.5175);
#8029=CYLINDRICAL_SURFACE('',#9064,3.0735);
#8030=CYLINDRICAL_SURFACE('',#9065,2.5175);
#8200=ADVANCED_FACE('',(#452),#7887,.F.);
#8201=ADVANCED_FACE('',(#453),#7888,.F.);
#8202=ADVANCED_FACE('',(#454),#7889,.F.);
#8203=ADVANCED_FACE('',(#455),#7890,.F.);
#8204=ADVANCED_FACE('',(#456),#7891,.F.);
#8205=ADVANCED_FACE('',(#457),#7892,.F.);
#8206=ADVANCED_FACE('',(#458),#7893,.F.);
#8207=ADVANCED_FACE('',(#459),#7894,.F.);
#8208=ADVANCED_FACE('',(#460),#7895,.F.);
#8209=ADVANCED_FACE('',(#461),#7896,.F.);
#8210=ADVANCED_FACE('',(#462),#7897,.F.);
#8211=ADVANCED_FACE('',(#463),#7898,.F.);
#8212=ADVANCED_FACE('',(#464),#7899,.F.);
#8213=ADVANCED_FACE('',(#465),#7900,.F.);
#8214=ADVANCED_FACE('',(#466),#7901,.F.);
#8215=ADVANCED_FACE('',(#467),#7902,.F.);
#8216=ADVANCED_FACE('',(#468),#7903,.F.);
#8217=ADVANCED_FACE('',(#469),#7904,.F.);
#8218=ADVANCED_FACE('',(#470),#7905,.F.);
#8219=ADVANCED_FACE('',(#471),#7906,.F.);
#8220=ADVANCED_FACE('',(#472),#7907,.F.);
#8221=ADVANCED_FACE('',(#473),#7908,.F.);
#8222=ADVANCED_FACE('',(#474),#7909,.F.);
#8223=ADVANCED_FACE('',(#475),#7910,.F.);
#8224=ADVANCED_FACE('',(#476),#7911,.F.);
#8225=ADVANCED_FACE('',(#477),#7912,.F.);
#8226=ADVANCED_FACE('',(#478),#7913,.F.);
#8227=ADVANCED_FACE('',(#479),#7914,.F.);
#8228=ADVANCED_FACE('',(#480),#7915,.F.);
#8229=ADVANCED_FACE('',(#481),#7916,.F.);
#8230=ADVANCED_FACE('',(#482),#7917,.F.);
#8231=ADVANCED_FACE('',(#483),#7918,.F.);
#8232=ADVANCED_FACE('',(#484),#7919,.F.);
#8233=ADVANCED_FACE('',(#485),#7920,.F.);
#8234=ADVANCED_FACE('',(#486),#7921,.F.);
#8235=ADVANCED_FACE('',(#487),#7922,.F.);
#8236=ADVANCED_FACE('',(#488),#7923,.F.);
#8237=ADVANCED_FACE('',(#489),#7924,.F.);
#8238=ADVANCED_FACE('',(#490),#7925,.F.);
#8239=ADVANCED_FACE('',(#491),#7926,.F.);
#8240=ADVANCED_FACE('',(#492),#7927,.F.);
#8241=ADVANCED_FACE('',(#493),#7928,.F.);
#8242=ADVANCED_FACE('',(#494),#7929,.F.);
#8243=ADVANCED_FACE('',(#495),#7930,.F.);
#8244=ADVANCED_FACE('',(#496),#7931,.F.);
#8245=ADVANCED_FACE('',(#497),#7932,.F.);
#8246=ADVANCED_FACE('',(#498),#7933,.F.);
#8247=ADVANCED_FACE('',(#499),#7934,.F.);
#8248=ADVANCED_FACE('',(#500),#7935,.F.);
#8249=ADVANCED_FACE('',(#501),#7936,.F.);
#8250=ADVANCED_FACE('',(#502),#7937,.F.);
#8251=ADVANCED_FACE('',(#503),#7938,.F.);
#8252=ADVANCED_FACE('',(#504),#7939,.F.);
#8253=ADVANCED_FACE('',(#505),#7940,.F.);
#8254=ADVANCED_FACE('',(#506),#7941,.F.);
#8255=ADVANCED_FACE('',(#507),#7942,.F.);
#8256=ADVANCED_FACE('',(#508),#7943,.F.);
#8257=ADVANCED_FACE('',(#509),#7944,.F.);
#8258=ADVANCED_FACE('',(#510),#7945,.F.);
#8259=ADVANCED_FACE('',(#511),#7946,.F.);
#8260=ADVANCED_FACE('',(#512),#7947,.F.);
#8261=ADVANCED_FACE('',(#513),#7948,.F.);
#8262=ADVANCED_FACE('',(#514),#7949,.F.);
#8263=ADVANCED_FACE('',(#515),#7950,.F.);
#8264=ADVANCED_FACE('',(#516),#7951,.F.);
#8265=ADVANCED_FACE('',(#517),#7952,.F.);
#8266=ADVANCED_FACE('',(#518),#7953,.F.);
#8267=ADVANCED_FACE('',(#519),#7954,.F.);
#8268=ADVANCED_FACE('',(#520),#7955,.F.);
#8269=ADVANCED_FACE('',(#521),#7956,.F.);
#8270=ADVANCED_FACE('',(#522),#7957,.F.);
#8271=ADVANCED_FACE('',(#523),#7958,.F.);
#8272=ADVANCED_FACE('',(#524),#7959,.F.);
#8273=ADVANCED_FACE('',(#525),#7960,.F.);
#8274=ADVANCED_FACE('',(#526),#7961,.F.);
#8275=ADVANCED_FACE('',(#527),#7962,.F.);
#8276=ADVANCED_FACE('',(#528),#7963,.F.);
#8277=ADVANCED_FACE('',(#529),#7964,.F.);
#8278=ADVANCED_FACE('',(#530),#7965,.F.);
#8279=ADVANCED_FACE('',(#531),#7966,.F.);
#8280=ADVANCED_FACE('',(#532),#7967,.F.);
#8281=ADVANCED_FACE('',(#533),#7968,.F.);
#8282=ADVANCED_FACE('',(#534),#7969,.F.);
#8283=ADVANCED_FACE('',(#535),#7970,.F.);
#8284=ADVANCED_FACE('',(#536),#7971,.F.);
#8285=ADVANCED_FACE('',(#537),#7972,.F.);
#8286=ADVANCED_FACE('',(#538),#7973,.F.);
#8287=ADVANCED_FACE('',(#539),#7974,.F.);
#8288=ADVANCED_FACE('',(#540),#7975,.F.);
#8289=ADVANCED_FACE('',(#541),#7976,.F.);
#8290=ADVANCED_FACE('',(#542),#7977,.F.);
#8291=ADVANCED_FACE('',(#543),#7978,.F.);
#8292=ADVANCED_FACE('',(#544),#7979,.F.);
#8293=ADVANCED_FACE('',(#545),#7980,.F.);
#8294=ADVANCED_FACE('',(#546),#7981,.F.);
#8295=ADVANCED_FACE('',(#547),#7982,.F.);
#8296=ADVANCED_FACE('',(#548),#7983,.F.);
#8297=ADVANCED_FACE('',(#549),#7984,.F.);
#8298=ADVANCED_FACE('',(#550),#7985,.F.);
#8299=ADVANCED_FACE('',(#551),#7986,.F.);
#8300=ADVANCED_FACE('',(#552),#7987,.F.);
#8301=ADVANCED_FACE('',(#553),#7988,.F.);
#8302=ADVANCED_FACE('',(#554),#7989,.F.);
#8303=ADVANCED_FACE('',(#555),#7990,.F.);
#8304=ADVANCED_FACE('',(#556),#7991,.F.);
#8305=ADVANCED_FACE('',(#557),#7992,.F.);
#8306=ADVANCED_FACE('',(#558),#7993,.F.);
#8307=ADVANCED_FACE('',(#559),#7994,.F.);
#8308=ADVANCED_FACE('',(#560),#7995,.F.);
#8309=ADVANCED_FACE('',(#561),#7996,.F.);
#8310=ADVANCED_FACE('',(#562),#7997,.F.);
#8311=ADVANCED_FACE('',(#563),#7998,.F.);
#8312=ADVANCED_FACE('',(#564),#7999,.F.);
#8313=ADVANCED_FACE('',(#565),#8000,.F.);
#8314=ADVANCED_FACE('',(#566),#8001,.F.);
#8315=ADVANCED_FACE('',(#567),#8002,.F.);
#8316=ADVANCED_FACE('',(#568),#8003,.F.);
#8317=ADVANCED_FACE('',(#569),#8004,.F.);
#8318=ADVANCED_FACE('',(#570),#8005,.F.);
#8319=ADVANCED_FACE('',(#571),#8006,.F.);
#8320=ADVANCED_FACE('',(#572),#8007,.F.);
#8321=ADVANCED_FACE('',(#573),#8008,.F.);
#8322=ADVANCED_FACE('',(#574),#8009,.F.);
#8323=ADVANCED_FACE('',(#575),#8010,.F.);
#8324=ADVANCED_FACE('',(#576),#8011,.F.);
#8325=ADVANCED_FACE('',(#577),#8012,.F.);
#8326=ADVANCED_FACE('',(#578),#8013,.F.);
#8327=ADVANCED_FACE('',(#579),#8014,.F.);
#8328=ADVANCED_FACE('',(#580),#8015,.F.);
#8329=ADVANCED_FACE('',(#581),#8016,.F.);
#8330=ADVANCED_FACE('',(#582),#8017,.F.);
#8331=ADVANCED_FACE('',(#583),#8018,.F.);
#8332=ADVANCED_FACE('',(#584),#8019,.F.);
#8333=ADVANCED_FACE('',(#585),#8020,.F.);
#8334=ADVANCED_FACE('',(#586),#8021,.F.);
#8335=ADVANCED_FACE('',(#587),#8022,.F.);
#8336=ADVANCED_FACE('',(#588),#311,.F.);
#8337=ADVANCED_FACE('',(#589),#8023,.F.);
#8338=ADVANCED_FACE('',(#590),#293,.F.);
#8339=ADVANCED_FACE('',(#591),#294,.F.);
#8340=ADVANCED_FACE('',(#592),#8024,.F.);
#8341=ADVANCED_FACE('',(#593),#312,.F.);
#8342=ADVANCED_FACE('',(#594),#8025,.F.);
#8343=ADVANCED_FACE('',(#595),#295,.F.);
#8344=ADVANCED_FACE('',(#596),#296,.F.);
#8345=ADVANCED_FACE('',(#597),#8026,.F.);
#8346=ADVANCED_FACE('',(#598),#313,.F.);
#8347=ADVANCED_FACE('',(#599),#8027,.F.);
#8348=ADVANCED_FACE('',(#600),#297,.F.);
#8349=ADVANCED_FACE('',(#601),#298,.F.);
#8350=ADVANCED_FACE('',(#602),#8028,.F.);
#8351=ADVANCED_FACE('',(#603),#314,.F.);
#8352=ADVANCED_FACE('',(#604),#8029,.F.);
#8353=ADVANCED_FACE('',(#605),#299,.F.);
#8354=ADVANCED_FACE('',(#606),#300,.F.);
#8355=ADVANCED_FACE('',(#607),#8030,.F.);
#8356=ADVANCED_FACE('',(#608),#315,.F.);
#8357=ADVANCED_FACE('',(#609),#316,.F.);
#8358=ADVANCED_FACE('',(#610),#317,.F.);
#8359=ADVANCED_FACE('',(#611),#318,.F.);
#8360=ADVANCED_FACE('',(#612),#319,.T.);
#8361=ADVANCED_FACE('',(#613),#320,.T.);
#8362=ADVANCED_FACE('',(#614),#321,.T.);
#8363=ADVANCED_FACE('',(#615),#322,.T.);
#8364=ADVANCED_FACE('',(#616),#323,.T.);
#8365=ADVANCED_FACE('',(#617),#324,.T.);
#8366=ADVANCED_FACE('',(#618),#325,.T.);
#8367=ADVANCED_FACE('',(#619),#326,.T.);
#8368=ADVANCED_FACE('',(#620,#234),#327,.T.);
#8369=ADVANCED_FACE('',(#621,#235,#236,#237,#238,#239),#328,.F.);
#8675=CLOSED_SHELL('',(#8200,#8201,#8202,#8203,#8204,#8205,#8206,#8207,
#8208,#8209,#8210,#8211,#8212,#8213,#8214,#8215,#8216,#8217,#8218,#8219,
#8220,#8221,#8222,#8223,#8224,#8225,#8226,#8227,#8228,#8229,#8230,#8231,
#8232,#8233,#8234,#8235,#8236,#8237,#8238,#8239,#8240,#8241,#8242,#8243,
#8244,#8245,#8246,#8247,#8248,#8249,#8250,#8251,#8252,#8253,#8254,#8255,
#8256,#8257,#8258,#8259,#8260,#8261,#8262,#8263,#8264,#8265,#8266,#8267,
#8268,#8269,#8270,#8271,#8272,#8273,#8274,#8275,#8276,#8277,#8278,#8279,
#8280,#8281,#8282,#8283,#8284,#8285,#8286,#8287,#8288,#8289,#8290,#8291,
#8292,#8293,#8294,#8295,#8296,#8297,#8298,#8299,#8300,#8301,#8302,#8303,
#8304,#8305,#8306,#8307,#8308,#8309,#8310,#8311,#8312,#8313,#8314,#8315,
#8316,#8317,#8318,#8319,#8320,#8321,#8322,#8323,#8324,#8325,#8326,#8327,
#8328,#8329,#8330,#8331,#8332,#8333,#8334,#8335,#8336,#8337,#8338,#8339,
#8340,#8341,#8342,#8343,#8344,#8345,#8346,#8347,#8348,#8349,#8350,#8351,
#8352,#8353,#8354,#8355,#8356,#8357,#8358,#8359,#8360,#8361,#8362,#8363,
#8364,#8365,#8366,#8367,#8368,#8369));
#8893=AXIS2_PLACEMENT_3D('',#11350,#9531,#9532);
#8894=AXIS2_PLACEMENT_3D('',#11351,#9533,#9534);
#8895=AXIS2_PLACEMENT_3D('',#11361,#9536,#9537);
#8896=AXIS2_PLACEMENT_3D('',#11364,#9539,#9540);
#8897=AXIS2_PLACEMENT_3D('',#11366,#9541,#9542);
#8898=AXIS2_PLACEMENT_3D('',#11377,#9543,#9544);
#8899=AXIS2_PLACEMENT_3D('',#11425,#9546,#9547);
#8900=AXIS2_PLACEMENT_3D('',#11476,#9549,#9550);
#8901=AXIS2_PLACEMENT_3D('',#11524,#9552,#9553);
#8902=AXIS2_PLACEMENT_3D('',#11572,#9555,#9556);
#8903=AXIS2_PLACEMENT_3D('',#11623,#9558,#9559);
#8904=AXIS2_PLACEMENT_3D('',#11674,#9561,#9562);
#8905=AXIS2_PLACEMENT_3D('',#11722,#9564,#9565);
#8906=AXIS2_PLACEMENT_3D('',#11773,#9567,#9568);
#8907=AXIS2_PLACEMENT_3D('',#11824,#9570,#9571);
#8908=AXIS2_PLACEMENT_3D('',#11872,#9573,#9574);
#8909=AXIS2_PLACEMENT_3D('',#11920,#9576,#9577);
#8910=AXIS2_PLACEMENT_3D('',#11971,#9579,#9580);
#8911=AXIS2_PLACEMENT_3D('',#12022,#9582,#9583);
#8912=AXIS2_PLACEMENT_3D('',#12070,#9585,#9586);
#8913=AXIS2_PLACEMENT_3D('',#12121,#9588,#9589);
#8914=AXIS2_PLACEMENT_3D('',#12140,#9591,#9592);
#8915=AXIS2_PLACEMENT_3D('',#12160,#9593,#9594);
#8916=AXIS2_PLACEMENT_3D('',#12174,#9596,#9597);
#8917=AXIS2_PLACEMENT_3D('',#12184,#9598,#9599);
#8918=AXIS2_PLACEMENT_3D('',#12208,#9601,#9602);
#8919=AXIS2_PLACEMENT_3D('',#12233,#9604,#9605);
#8920=AXIS2_PLACEMENT_3D('',#12257,#9607,#9608);
#8921=AXIS2_PLACEMENT_3D('',#12282,#9610,#9611);
#8922=AXIS2_PLACEMENT_3D('',#12306,#9613,#9614);
#8923=AXIS2_PLACEMENT_3D('',#12331,#9616,#9617);
#8924=AXIS2_PLACEMENT_3D('',#12356,#9619,#9620);
#8925=AXIS2_PLACEMENT_3D('',#12380,#9622,#9623);
#8926=AXIS2_PLACEMENT_3D('',#12405,#9625,#9626);
#8927=AXIS2_PLACEMENT_3D('',#12429,#9628,#9629);
#8928=AXIS2_PLACEMENT_3D('',#12454,#9631,#9632);
#8929=AXIS2_PLACEMENT_3D('',#12478,#9634,#9635);
#8930=AXIS2_PLACEMENT_3D('',#12503,#9637,#9638);
#8931=AXIS2_PLACEMENT_3D('',#12528,#9640,#9641);
#8932=AXIS2_PLACEMENT_3D('',#12552,#9643,#9644);
#8933=AXIS2_PLACEMENT_3D('',#12563,#9646,#9647);
#8934=AXIS2_PLACEMENT_3D('',#12569,#9648,#9649);
#8935=AXIS2_PLACEMENT_3D('',#12579,#9651,#9652);
#8936=AXIS2_PLACEMENT_3D('',#12582,#9654,#9655);
#8937=AXIS2_PLACEMENT_3D('',#12584,#9656,#9657);
#8938=AXIS2_PLACEMENT_3D('',#12595,#9658,#9659);
#8939=AXIS2_PLACEMENT_3D('',#12643,#9661,#9662);
#8940=AXIS2_PLACEMENT_3D('',#12694,#9664,#9665);
#8941=AXIS2_PLACEMENT_3D('',#12742,#9667,#9668);
#8942=AXIS2_PLACEMENT_3D('',#12790,#9670,#9671);
#8943=AXIS2_PLACEMENT_3D('',#12841,#9673,#9674);
#8944=AXIS2_PLACEMENT_3D('',#12892,#9676,#9677);
#8945=AXIS2_PLACEMENT_3D('',#12940,#9679,#9680);
#8946=AXIS2_PLACEMENT_3D('',#12991,#9682,#9683);
#8947=AXIS2_PLACEMENT_3D('',#13042,#9685,#9686);
#8948=AXIS2_PLACEMENT_3D('',#13090,#9688,#9689);
#8949=AXIS2_PLACEMENT_3D('',#13138,#9691,#9692);
#8950=AXIS2_PLACEMENT_3D('',#13189,#9694,#9695);
#8951=AXIS2_PLACEMENT_3D('',#13240,#9697,#9698);
#8952=AXIS2_PLACEMENT_3D('',#13288,#9700,#9701);
#8953=AXIS2_PLACEMENT_3D('',#13339,#9703,#9704);
#8954=AXIS2_PLACEMENT_3D('',#13358,#9706,#9707);
#8955=AXIS2_PLACEMENT_3D('',#13378,#9708,#9709);
#8956=AXIS2_PLACEMENT_3D('',#13392,#9711,#9712);
#8957=AXIS2_PLACEMENT_3D('',#13402,#9713,#9714);
#8958=AXIS2_PLACEMENT_3D('',#13426,#9716,#9717);
#8959=AXIS2_PLACEMENT_3D('',#13451,#9719,#9720);
#8960=AXIS2_PLACEMENT_3D('',#13475,#9722,#9723);
#8961=AXIS2_PLACEMENT_3D('',#13500,#9725,#9726);
#8962=AXIS2_PLACEMENT_3D('',#13524,#9728,#9729);
#8963=AXIS2_PLACEMENT_3D('',#13549,#9731,#9732);
#8964=AXIS2_PLACEMENT_3D('',#13574,#9734,#9735);
#8965=AXIS2_PLACEMENT_3D('',#13598,#9737,#9738);
#8966=AXIS2_PLACEMENT_3D('',#13623,#9740,#9741);
#8967=AXIS2_PLACEMENT_3D('',#13647,#9743,#9744);
#8968=AXIS2_PLACEMENT_3D('',#13672,#9746,#9747);
#8969=AXIS2_PLACEMENT_3D('',#13696,#9749,#9750);
#8970=AXIS2_PLACEMENT_3D('',#13721,#9752,#9753);
#8971=AXIS2_PLACEMENT_3D('',#13746,#9755,#9756);
#8972=AXIS2_PLACEMENT_3D('',#13770,#9758,#9759);
#8973=AXIS2_PLACEMENT_3D('',#13781,#9761,#9762);
#8974=AXIS2_PLACEMENT_3D('',#13787,#9763,#9764);
#8975=AXIS2_PLACEMENT_3D('',#13797,#9766,#9767);
#8976=AXIS2_PLACEMENT_3D('',#13800,#9769,#9770);
#8977=AXIS2_PLACEMENT_3D('',#13802,#9771,#9772);
#8978=AXIS2_PLACEMENT_3D('',#13813,#9773,#9774);
#8979=AXIS2_PLACEMENT_3D('',#13861,#9776,#9777);
#8980=AXIS2_PLACEMENT_3D('',#13912,#9779,#9780);
#8981=AXIS2_PLACEMENT_3D('',#13960,#9782,#9783);
#8982=AXIS2_PLACEMENT_3D('',#14008,#9785,#9786);
#8983=AXIS2_PLACEMENT_3D('',#14059,#9788,#9789);
#8984=AXIS2_PLACEMENT_3D('',#14110,#9791,#9792);
#8985=AXIS2_PLACEMENT_3D('',#14158,#9794,#9795);
#8986=AXIS2_PLACEMENT_3D('',#14209,#9797,#9798);
#8987=AXIS2_PLACEMENT_3D('',#14260,#9800,#9801);
#8988=AXIS2_PLACEMENT_3D('',#14308,#9803,#9804);
#8989=AXIS2_PLACEMENT_3D('',#14356,#9806,#9807);
#8990=AXIS2_PLACEMENT_3D('',#14407,#9809,#9810);
#8991=AXIS2_PLACEMENT_3D('',#14458,#9812,#9813);
#8992=AXIS2_PLACEMENT_3D('',#14506,#9815,#9816);
#8993=AXIS2_PLACEMENT_3D('',#14557,#9818,#9819);
#8994=AXIS2_PLACEMENT_3D('',#14576,#9821,#9822);
#8995=AXIS2_PLACEMENT_3D('',#14596,#9823,#9824);
#8996=AXIS2_PLACEMENT_3D('',#14610,#9826,#9827);
#8997=AXIS2_PLACEMENT_3D('',#14620,#9828,#9829);
#8998=AXIS2_PLACEMENT_3D('',#14644,#9831,#9832);
#8999=AXIS2_PLACEMENT_3D('',#14669,#9834,#9835);
#9000=AXIS2_PLACEMENT_3D('',#14693,#9837,#9838);
#9001=AXIS2_PLACEMENT_3D('',#14718,#9840,#9841);
#9002=AXIS2_PLACEMENT_3D('',#14742,#9843,#9844);
#9003=AXIS2_PLACEMENT_3D('',#14767,#9846,#9847);
#9004=AXIS2_PLACEMENT_3D('',#14792,#9849,#9850);
#9005=AXIS2_PLACEMENT_3D('',#14816,#9852,#9853);
#9006=AXIS2_PLACEMENT_3D('',#14841,#9855,#9856);
#9007=AXIS2_PLACEMENT_3D('',#14865,#9858,#9859);
#9008=AXIS2_PLACEMENT_3D('',#14890,#9861,#9862);
#9009=AXIS2_PLACEMENT_3D('',#14914,#9864,#9865);
#9010=AXIS2_PLACEMENT_3D('',#14939,#9867,#9868);
#9011=AXIS2_PLACEMENT_3D('',#14964,#9870,#9871);
#9012=AXIS2_PLACEMENT_3D('',#14988,#9873,#9874);
#9013=AXIS2_PLACEMENT_3D('',#14999,#9876,#9877);
#9014=AXIS2_PLACEMENT_3D('',#15005,#9878,#9879);
#9015=AXIS2_PLACEMENT_3D('',#15015,#9881,#9882);
#9016=AXIS2_PLACEMENT_3D('',#15018,#9884,#9885);
#9017=AXIS2_PLACEMENT_3D('',#15020,#9886,#9887);
#9018=AXIS2_PLACEMENT_3D('',#15031,#9888,#9889);
#9019=AXIS2_PLACEMENT_3D('',#15079,#9891,#9892);
#9020=AXIS2_PLACEMENT_3D('',#15130,#9894,#9895);
#9021=AXIS2_PLACEMENT_3D('',#15178,#9897,#9898);
#9022=AXIS2_PLACEMENT_3D('',#15226,#9900,#9901);
#9023=AXIS2_PLACEMENT_3D('',#15277,#9903,#9904);
#9024=AXIS2_PLACEMENT_3D('',#15328,#9906,#9907);
#9025=AXIS2_PLACEMENT_3D('',#15376,#9909,#9910);
#9026=AXIS2_PLACEMENT_3D('',#15427,#9912,#9913);
#9027=AXIS2_PLACEMENT_3D('',#15478,#9915,#9916);
#9028=AXIS2_PLACEMENT_3D('',#15526,#9918,#9919);
#9029=AXIS2_PLACEMENT_3D('',#15574,#9921,#9922);
#9030=AXIS2_PLACEMENT_3D('',#15625,#9924,#9925);
#9031=AXIS2_PLACEMENT_3D('',#15676,#9927,#9928);
#9032=AXIS2_PLACEMENT_3D('',#15724,#9930,#9931);
#9033=AXIS2_PLACEMENT_3D('',#15775,#9933,#9934);
#9034=AXIS2_PLACEMENT_3D('',#15794,#9936,#9937);
#9035=AXIS2_PLACEMENT_3D('',#15814,#9938,#9939);
#9036=AXIS2_PLACEMENT_3D('',#15828,#9941,#9942);
#9037=AXIS2_PLACEMENT_3D('',#15838,#9943,#9944);
#9038=AXIS2_PLACEMENT_3D('',#15862,#9946,#9947);
#9039=AXIS2_PLACEMENT_3D('',#15887,#9949,#9950);
#9040=AXIS2_PLACEMENT_3D('',#15911,#9952,#9953);
#9041=AXIS2_PLACEMENT_3D('',#15936,#9955,#9956);
#9042=AXIS2_PLACEMENT_3D('',#15960,#9958,#9959);
#9043=AXIS2_PLACEMENT_3D('',#15985,#9961,#9962);
#9044=AXIS2_PLACEMENT_3D('',#16010,#9964,#9965);
#9045=AXIS2_PLACEMENT_3D('',#16034,#9967,#9968);
#9046=AXIS2_PLACEMENT_3D('',#16059,#9970,#9971);
#9047=AXIS2_PLACEMENT_3D('',#16083,#9973,#9974);
#9048=AXIS2_PLACEMENT_3D('',#16108,#9976,#9977);
#9049=AXIS2_PLACEMENT_3D('',#16132,#9979,#9980);
#9050=AXIS2_PLACEMENT_3D('',#16157,#9982,#9983);
#9051=AXIS2_PLACEMENT_3D('',#16182,#9985,#9986);
#9052=AXIS2_PLACEMENT_3D('',#16206,#9988,#9989);
#9053=AXIS2_PLACEMENT_3D('',#16217,#9991,#9992);
#9054=AXIS2_PLACEMENT_3D('',#16223,#9993,#9994);
#9055=AXIS2_PLACEMENT_3D('',#16406,#9995,#9996);
#9056=AXIS2_PLACEMENT_3D('',#17562,#9997,#9998);
#9057=AXIS2_PLACEMENT_3D('',#17563,#9999,#10000);
#9058=AXIS2_PLACEMENT_3D('',#17746,#10001,#10002);
#9059=AXIS2_PLACEMENT_3D('',#18902,#10003,#10004);
#9060=AXIS2_PLACEMENT_3D('',#18903,#10005,#10006);
#9061=AXIS2_PLACEMENT_3D('',#19086,#10007,#10008);
#9062=AXIS2_PLACEMENT_3D('',#20242,#10009,#10010);
#9063=AXIS2_PLACEMENT_3D('',#20243,#10011,#10012);
#9064=AXIS2_PLACEMENT_3D('',#20426,#10013,#10014);
#9065=AXIS2_PLACEMENT_3D('',#21582,#10015,#10016);
#9066=AXIS2_PLACEMENT_3D('',#21583,#10017,#10018);
#9067=AXIS2_PLACEMENT_3D('',#21584,#10019,#10020);
#9068=AXIS2_PLACEMENT_3D('',#21585,#10021,#10022);
#9069=AXIS2_PLACEMENT_3D('',#21586,#10023,#10024);
#9070=AXIS2_PLACEMENT_3D('',#21587,#10025,#10026);
#9071=AXIS2_PLACEMENT_3D('',#21596,#10031,#10032);
#9072=AXIS2_PLACEMENT_3D('',#21602,#10036,#10037);
#9073=AXIS2_PLACEMENT_3D('',#21608,#10041,#10042);
#9074=AXIS2_PLACEMENT_3D('',#21611,#10045,#10046);
#9075=AXIS2_PLACEMENT_3D('',#21620,#10051,#10052);
#9076=AXIS2_PLACEMENT_3D('',#21626,#10056,#10057);
#9077=AXIS2_PLACEMENT_3D('',#21632,#10061,#10062);
#9078=AXIS2_PLACEMENT_3D('',#21635,#10065,#10066);
#9079=AXIS2_PLACEMENT_3D('',#21636,#10067,#10068);
#9531=DIRECTION('axis',(0.,0.,1.));
#9532=DIRECTION('refdir',(1.,0.,0.));
#9533=DIRECTION('center_axis',(0.,0.,1.));
#9534=DIRECTION('ref_axis',(-1.,0.,0.));
#9535=DIRECTION('',(0.,0.,1.));
#9536=DIRECTION('center_axis',(0.,0.,-1.));
#9537=DIRECTION('ref_axis',(-1.,0.,0.));
#9538=DIRECTION('',(0.,0.,1.));
#9539=DIRECTION('center_axis',(0.,0.,-1.));
#9540=DIRECTION('ref_axis',(-1.,0.,0.));
#9541=DIRECTION('center_axis',(0.,0.,-1.));
#9542=DIRECTION('ref_axis',(-1.,0.,0.));
#9543=DIRECTION('center_axis',(0.,0.,1.));
#9544=DIRECTION('ref_axis',(-1.,0.,0.));
#9545=DIRECTION('',(0.,0.,1.));
#9546=DIRECTION('center_axis',(0.,0.,1.));
#9547=DIRECTION('ref_axis',(-1.,0.,0.));
#9548=DIRECTION('',(0.,0.,1.));
#9549=DIRECTION('center_axis',(0.,0.,1.));
#9550=DIRECTION('ref_axis',(-1.,0.,0.));
#9551=DIRECTION('',(0.,0.,1.));
#9552=DIRECTION('center_axis',(0.,0.,1.));
#9553=DIRECTION('ref_axis',(-1.,0.,0.));
#9554=DIRECTION('',(0.,0.,1.));
#9555=DIRECTION('center_axis',(0.,0.,1.));
#9556=DIRECTION('ref_axis',(-1.,0.,0.));
#9557=DIRECTION('',(0.,0.,1.));
#9558=DIRECTION('center_axis',(0.,0.,1.));
#9559=DIRECTION('ref_axis',(-1.,0.,0.));
#9560=DIRECTION('',(0.,0.,1.));
#9561=DIRECTION('center_axis',(0.,0.,1.));
#9562=DIRECTION('ref_axis',(-1.,0.,0.));
#9563=DIRECTION('',(0.,0.,1.));
#9564=DIRECTION('center_axis',(0.,0.,1.));
#9565=DIRECTION('ref_axis',(-1.,0.,0.));
#9566=DIRECTION('',(0.,0.,1.));
#9567=DIRECTION('center_axis',(0.,0.,1.));
#9568=DIRECTION('ref_axis',(-1.,0.,0.));
#9569=DIRECTION('',(0.,0.,1.));
#9570=DIRECTION('center_axis',(0.,0.,1.));
#9571=DIRECTION('ref_axis',(-1.,0.,0.));
#9572=DIRECTION('',(0.,0.,1.));
#9573=DIRECTION('center_axis',(0.,0.,1.));
#9574=DIRECTION('ref_axis',(-1.,0.,0.));
#9575=DIRECTION('',(0.,0.,1.));
#9576=DIRECTION('center_axis',(0.,0.,1.));
#9577=DIRECTION('ref_axis',(-1.,0.,0.));
#9578=DIRECTION('',(0.,0.,1.));
#9579=DIRECTION('center_axis',(0.,0.,1.));
#9580=DIRECTION('ref_axis',(-1.,0.,0.));
#9581=DIRECTION('',(0.,0.,1.));
#9582=DIRECTION('center_axis',(0.,0.,1.));
#9583=DIRECTION('ref_axis',(-1.,0.,0.));
#9584=DIRECTION('',(0.,0.,1.));
#9585=DIRECTION('center_axis',(0.,0.,1.));
#9586=DIRECTION('ref_axis',(-1.,0.,0.));
#9587=DIRECTION('',(0.,0.,1.));
#9588=DIRECTION('center_axis',(0.,0.,1.));
#9589=DIRECTION('ref_axis',(-0.937990746613933,-0.34666029375548,0.));
#9590=DIRECTION('',(0.,0.,1.));
#9591=DIRECTION('center_axis',(0.,0.,-1.));
#9592=DIRECTION('ref_axis',(-1.,0.,0.));
#9593=DIRECTION('center_axis',(0.,0.,1.));
#9594=DIRECTION('ref_axis',(-1.,-9.82530218636873E-14,0.));
#9595=DIRECTION('',(-1.22464679914735E-16,-1.20475224710186E-29,1.));
#9596=DIRECTION('center_axis',(0.,0.,-1.));
#9597=DIRECTION('ref_axis',(-1.,-9.82530218636873E-14,0.));
#9598=DIRECTION('center_axis',(0.,0.,1.));
#9599=DIRECTION('ref_axis',(-1.,-9.82530218636873E-14,0.));
#9600=DIRECTION('',(-1.22464679914735E-16,-1.20475224710186E-29,1.));
#9601=DIRECTION('center_axis',(0.,0.,1.));
#9602=DIRECTION('ref_axis',(-1.,-9.82530218636873E-14,0.));
#9603=DIRECTION('',(-1.22464679914735E-16,-1.20475224710186E-29,1.));
#9604=DIRECTION('center_axis',(0.,0.,1.));
#9605=DIRECTION('ref_axis',(-1.,-9.82530218636873E-14,0.));
#9606=DIRECTION('',(-1.22464679914735E-16,-1.20475224710186E-29,1.));
#9607=DIRECTION('center_axis',(0.,0.,1.));
#9608=DIRECTION('ref_axis',(-1.,-9.82530218636873E-14,0.));
#9609=DIRECTION('',(-1.22464679914735E-16,-1.20475224710186E-29,1.));
#9610=DIRECTION('center_axis',(0.,0.,1.));
#9611=DIRECTION('ref_axis',(-1.,-9.82530218636873E-14,0.));
#9612=DIRECTION('',(-1.22464679914735E-16,-1.20475224710186E-29,1.));
#9613=DIRECTION('center_axis',(0.,0.,1.));
#9614=DIRECTION('ref_axis',(-1.,-9.82530218636873E-14,0.));
#9615=DIRECTION('',(-1.22464679914735E-16,-1.20475224710186E-29,1.));
#9616=DIRECTION('center_axis',(0.,0.,1.));
#9617=DIRECTION('ref_axis',(-1.,-9.82530218636873E-14,0.));
#9618=DIRECTION('',(-1.22464679914735E-16,-1.20475224710186E-29,1.));
#9619=DIRECTION('center_axis',(0.,0.,1.));
#9620=DIRECTION('ref_axis',(-1.,-9.82530218636873E-14,0.));
#9621=DIRECTION('',(-1.22464679914735E-16,-1.20475224710186E-29,1.));
#9622=DIRECTION('center_axis',(0.,0.,1.));
#9623=DIRECTION('ref_axis',(-1.,-9.82530218636873E-14,0.));
#9624=DIRECTION('',(-1.22464679914735E-16,-1.20475224710186E-29,1.));
#9625=DIRECTION('center_axis',(0.,0.,1.));
#9626=DIRECTION('ref_axis',(-1.,-9.82530218636873E-14,0.));
#9627=DIRECTION('',(-1.22464679914735E-16,-1.20475224710186E-29,1.));
#9628=DIRECTION('center_axis',(0.,0.,1.));
#9629=DIRECTION('ref_axis',(-1.,-9.82530218636873E-14,0.));
#9630=DIRECTION('',(-1.22464679914735E-16,-1.20475224710186E-29,1.));
#9631=DIRECTION('center_axis',(0.,0.,1.));
#9632=DIRECTION('ref_axis',(-1.,-9.82530218636873E-14,0.));
#9633=DIRECTION('',(-1.22464679914735E-16,-1.20475224710186E-29,1.));
#9634=DIRECTION('center_axis',(0.,0.,1.));
#9635=DIRECTION('ref_axis',(-1.,-9.82530218636873E-14,0.));
#9636=DIRECTION('',(-1.22464679914735E-16,-1.20475224710186E-29,1.));
#9637=DIRECTION('center_axis',(0.,0.,1.));
#9638=DIRECTION('ref_axis',(-1.,-9.82530218636873E-14,0.));
#9639=DIRECTION('',(-1.22464679914735E-16,-1.20475224710186E-29,1.));
#9640=DIRECTION('center_axis',(0.,0.,1.));
#9641=DIRECTION('ref_axis',(-1.,-9.82530218636873E-14,0.));
#9642=DIRECTION('',(-1.22464679914735E-16,-1.20475224710186E-29,1.));
#9643=DIRECTION('center_axis',(0.,0.,1.));
#9644=DIRECTION('ref_axis',(0.60923771710773,-0.792987644325787,0.));
#9645=DIRECTION('',(-1.22464679914735E-16,-1.20475224710186E-29,1.));
#9646=DIRECTION('center_axis',(0.,0.,1.));
#9647=DIRECTION('ref_axis',(-1.,-9.82530218636873E-14,0.));
#9648=DIRECTION('center_axis',(0.,0.,1.));
#9649=DIRECTION('ref_axis',(-1.,0.,0.));
#9650=DIRECTION('',(0.,0.,1.));
#9651=DIRECTION('center_axis',(0.,0.,-1.));
#9652=DIRECTION('ref_axis',(-1.,0.,0.));
#9653=DIRECTION('',(0.,0.,1.));
#9654=DIRECTION('center_axis',(0.,0.,-1.));
#9655=DIRECTION('ref_axis',(-1.,0.,0.));
#9656=DIRECTION('center_axis',(0.,0.,-1.));
#9657=DIRECTION('ref_axis',(-1.,0.,0.));
#9658=DIRECTION('center_axis',(0.,0.,1.));
#9659=DIRECTION('ref_axis',(-1.,0.,0.));
#9660=DIRECTION('',(0.,0.,1.));
#9661=DIRECTION('center_axis',(0.,0.,1.));
#9662=DIRECTION('ref_axis',(-1.,0.,0.));
#9663=DIRECTION('',(0.,0.,1.));
#9664=DIRECTION('center_axis',(0.,0.,1.));
#9665=DIRECTION('ref_axis',(-1.,0.,0.));
#9666=DIRECTION('',(0.,0.,1.));
#9667=DIRECTION('center_axis',(0.,0.,1.));
#9668=DIRECTION('ref_axis',(-1.,0.,0.));
#9669=DIRECTION('',(0.,0.,1.));
#9670=DIRECTION('center_axis',(0.,0.,1.));
#9671=DIRECTION('ref_axis',(-1.,0.,0.));
#9672=DIRECTION('',(0.,0.,1.));
#9673=DIRECTION('center_axis',(0.,0.,1.));
#9674=DIRECTION('ref_axis',(-1.,0.,0.));
#9675=DIRECTION('',(0.,0.,1.));
#9676=DIRECTION('center_axis',(0.,0.,1.));
#9677=DIRECTION('ref_axis',(-1.,0.,0.));
#9678=DIRECTION('',(0.,0.,1.));
#9679=DIRECTION('center_axis',(0.,0.,1.));
#9680=DIRECTION('ref_axis',(-1.,0.,0.));
#9681=DIRECTION('',(0.,0.,1.));
#9682=DIRECTION('center_axis',(0.,0.,1.));
#9683=DIRECTION('ref_axis',(-1.,0.,0.));
#9684=DIRECTION('',(0.,0.,1.));
#9685=DIRECTION('center_axis',(0.,0.,1.));
#9686=DIRECTION('ref_axis',(-1.,0.,0.));
#9687=DIRECTION('',(0.,0.,1.));
#9688=DIRECTION('center_axis',(0.,0.,1.));
#9689=DIRECTION('ref_axis',(-1.,0.,0.));
#9690=DIRECTION('',(0.,0.,1.));
#9691=DIRECTION('center_axis',(0.,0.,1.));
#9692=DIRECTION('ref_axis',(-1.,0.,0.));
#9693=DIRECTION('',(0.,0.,1.));
#9694=DIRECTION('center_axis',(0.,0.,1.));
#9695=DIRECTION('ref_axis',(-1.,0.,0.));
#9696=DIRECTION('',(0.,0.,1.));
#9697=DIRECTION('center_axis',(0.,0.,1.));
#9698=DIRECTION('ref_axis',(-1.,0.,0.));
#9699=DIRECTION('',(0.,0.,1.));
#9700=DIRECTION('center_axis',(0.,0.,1.));
#9701=DIRECTION('ref_axis',(-1.,0.,0.));
#9702=DIRECTION('',(0.,0.,1.));
#9703=DIRECTION('center_axis',(0.,0.,1.));
#9704=DIRECTION('ref_axis',(-0.937990745316897,-0.346660297264991,0.));
#9705=DIRECTION('',(0.,0.,1.));
#9706=DIRECTION('center_axis',(0.,0.,-1.));
#9707=DIRECTION('ref_axis',(-1.,0.,0.));
#9708=DIRECTION('center_axis',(0.,0.,1.));
#9709=DIRECTION('ref_axis',(-1.,-1.09812200906474E-13,0.));
#9710=DIRECTION('',(-1.22464679914735E-16,-1.34631136325706E-29,1.));
#9711=DIRECTION('center_axis',(0.,0.,-1.));
#9712=DIRECTION('ref_axis',(-1.,-1.09812200906474E-13,0.));
#9713=DIRECTION('center_axis',(0.,0.,1.));
#9714=DIRECTION('ref_axis',(-1.,-1.09812200906474E-13,0.));
#9715=DIRECTION('',(-1.22464679914735E-16,-1.34631136325706E-29,1.));
#9716=DIRECTION('center_axis',(0.,0.,1.));
#9717=DIRECTION('ref_axis',(-1.,-1.09812200906474E-13,0.));
#9718=DIRECTION('',(-1.22464679914735E-16,-1.34631136325706E-29,1.));
#9719=DIRECTION('center_axis',(0.,0.,1.));
#9720=DIRECTION('ref_axis',(-1.,-1.09812200906474E-13,0.));
#9721=DIRECTION('',(-1.22464679914735E-16,-1.34631136325706E-29,1.));
#9722=DIRECTION('center_axis',(0.,0.,1.));
#9723=DIRECTION('ref_axis',(-1.,-1.09812200906474E-13,0.));
#9724=DIRECTION('',(-1.22464679914735E-16,-1.34631136325706E-29,1.));
#9725=DIRECTION('center_axis',(0.,0.,1.));
#9726=DIRECTION('ref_axis',(-1.,-1.09812200906474E-13,0.));
#9727=DIRECTION('',(-1.22464679914735E-16,-1.34631136325706E-29,1.));
#9728=DIRECTION('center_axis',(0.,0.,1.));
#9729=DIRECTION('ref_axis',(-1.,-1.09812200906474E-13,0.));
#9730=DIRECTION('',(-1.22464679914735E-16,-1.34631136325706E-29,1.));
#9731=DIRECTION('center_axis',(0.,0.,1.));
#9732=DIRECTION('ref_axis',(-1.,-1.09812200906474E-13,0.));
#9733=DIRECTION('',(-1.22464679914735E-16,-1.34631136325706E-29,1.));
#9734=DIRECTION('center_axis',(0.,0.,1.));
#9735=DIRECTION('ref_axis',(-1.,-1.09812200906474E-13,0.));
#9736=DIRECTION('',(-1.22464679914735E-16,-1.34631136325706E-29,1.));
#9737=DIRECTION('center_axis',(0.,0.,1.));
#9738=DIRECTION('ref_axis',(-1.,-1.09812200906474E-13,0.));
#9739=DIRECTION('',(-1.22464679914735E-16,-1.34631136325706E-29,1.));
#9740=DIRECTION('center_axis',(0.,0.,1.));
#9741=DIRECTION('ref_axis',(-1.,-1.09812200906474E-13,0.));
#9742=DIRECTION('',(-1.22464679914735E-16,-1.34631136325706E-29,1.));
#9743=DIRECTION('center_axis',(0.,0.,1.));
#9744=DIRECTION('ref_axis',(-1.,-1.09812200906474E-13,0.));
#9745=DIRECTION('',(-1.22464679914735E-16,-1.34631136325706E-29,1.));
#9746=DIRECTION('center_axis',(0.,0.,1.));
#9747=DIRECTION('ref_axis',(-1.,-1.09812200906474E-13,0.));
#9748=DIRECTION('',(-1.22464679914735E-16,-1.34631136325706E-29,1.));
#9749=DIRECTION('center_axis',(0.,0.,1.));
#9750=DIRECTION('ref_axis',(-1.,-1.09812200906474E-13,0.));
#9751=DIRECTION('',(-1.22464679914735E-16,-1.34631136325706E-29,1.));
#9752=DIRECTION('center_axis',(0.,0.,1.));
#9753=DIRECTION('ref_axis',(-1.,-1.09812200906474E-13,0.));
#9754=DIRECTION('',(-1.22464679914735E-16,-1.34631136325706E-29,1.));
#9755=DIRECTION('center_axis',(0.,0.,1.));
#9756=DIRECTION('ref_axis',(-1.,-1.09812200906474E-13,0.));
#9757=DIRECTION('',(-1.22464679914735E-16,-1.34631136325706E-29,1.));
#9758=DIRECTION('center_axis',(0.,0.,1.));
#9759=DIRECTION('ref_axis',(0.609237720020655,-0.792987642087841,0.));
#9760=DIRECTION('',(-1.22464679914735E-16,-1.34631136325706E-29,1.));
#9761=DIRECTION('center_axis',(0.,0.,1.));
#9762=DIRECTION('ref_axis',(-1.,-1.09812200906474E-13,0.));
#9763=DIRECTION('center_axis',(0.,0.,1.));
#9764=DIRECTION('ref_axis',(-1.,0.,0.));
#9765=DIRECTION('',(0.,0.,1.));
#9766=DIRECTION('center_axis',(0.,0.,-1.));
#9767=DIRECTION('ref_axis',(-1.,0.,0.));
#9768=DIRECTION('',(0.,0.,1.));
#9769=DIRECTION('center_axis',(0.,0.,-1.));
#9770=DIRECTION('ref_axis',(-1.,0.,0.));
#9771=DIRECTION('center_axis',(0.,0.,-1.));
#9772=DIRECTION('ref_axis',(-1.,0.,0.));
#9773=DIRECTION('center_axis',(0.,0.,1.));
#9774=DIRECTION('ref_axis',(-1.,0.,0.));
#9775=DIRECTION('',(0.,0.,1.));
#9776=DIRECTION('center_axis',(0.,0.,1.));
#9777=DIRECTION('ref_axis',(-1.,0.,0.));
#9778=DIRECTION('',(0.,0.,1.));
#9779=DIRECTION('center_axis',(0.,0.,1.));
#9780=DIRECTION('ref_axis',(-1.,0.,0.));
#9781=DIRECTION('',(0.,0.,1.));
#9782=DIRECTION('center_axis',(0.,0.,1.));
#9783=DIRECTION('ref_axis',(-1.,0.,0.));
#9784=DIRECTION('',(0.,0.,1.));
#9785=DIRECTION('center_axis',(0.,0.,1.));
#9786=DIRECTION('ref_axis',(-1.,0.,0.));
#9787=DIRECTION('',(0.,0.,1.));
#9788=DIRECTION('center_axis',(0.,0.,1.));
#9789=DIRECTION('ref_axis',(-1.,0.,0.));
#9790=DIRECTION('',(0.,0.,1.));
#9791=DIRECTION('center_axis',(0.,0.,1.));
#9792=DIRECTION('ref_axis',(-1.,0.,0.));
#9793=DIRECTION('',(0.,0.,1.));
#9794=DIRECTION('center_axis',(0.,0.,1.));
#9795=DIRECTION('ref_axis',(-1.,0.,0.));
#9796=DIRECTION('',(0.,0.,1.));
#9797=DIRECTION('center_axis',(0.,0.,1.));
#9798=DIRECTION('ref_axis',(-1.,0.,0.));
#9799=DIRECTION('',(0.,0.,1.));
#9800=DIRECTION('center_axis',(0.,0.,1.));
#9801=DIRECTION('ref_axis',(-1.,0.,0.));
#9802=DIRECTION('',(0.,0.,1.));
#9803=DIRECTION('center_axis',(0.,0.,1.));
#9804=DIRECTION('ref_axis',(-1.,0.,0.));
#9805=DIRECTION('',(0.,0.,1.));
#9806=DIRECTION('center_axis',(0.,0.,1.));
#9807=DIRECTION('ref_axis',(-1.,0.,0.));
#9808=DIRECTION('',(0.,0.,1.));
#9809=DIRECTION('center_axis',(0.,0.,1.));
#9810=DIRECTION('ref_axis',(-1.,0.,0.));
#9811=DIRECTION('',(0.,0.,1.));
#9812=DIRECTION('center_axis',(0.,0.,1.));
#9813=DIRECTION('ref_axis',(-1.,0.,0.));
#9814=DIRECTION('',(0.,0.,1.));
#9815=DIRECTION('center_axis',(0.,0.,1.));
#9816=DIRECTION('ref_axis',(-1.,0.,0.));
#9817=DIRECTION('',(0.,0.,1.));
#9818=DIRECTION('center_axis',(0.,0.,1.));
#9819=DIRECTION('ref_axis',(-0.937990855083185,-0.346660000260074,0.));
#9820=DIRECTION('',(0.,0.,1.));
#9821=DIRECTION('center_axis',(0.,0.,-1.));
#9822=DIRECTION('ref_axis',(-1.,0.,0.));
#9823=DIRECTION('center_axis',(0.,0.,1.));
#9824=DIRECTION('ref_axis',(-1.,-1.01142816624385E-13,0.));
#9825=DIRECTION('',(-1.22464679914735E-16,-1.24014202614067E-29,1.));
#9826=DIRECTION('center_axis',(0.,0.,-1.));
#9827=DIRECTION('ref_axis',(-1.,-1.01142816624385E-13,0.));
#9828=DIRECTION('center_axis',(0.,0.,1.));
#9829=DIRECTION('ref_axis',(-1.,-1.01142816624385E-13,0.));
#9830=DIRECTION('',(-1.22464679914735E-16,-1.24014202614067E-29,1.));
#9831=DIRECTION('center_axis',(0.,0.,1.));
#9832=DIRECTION('ref_axis',(-1.,-1.01142816624385E-13,0.));
#9833=DIRECTION('',(-1.22464679914735E-16,-1.24014202614067E-29,1.));
#9834=DIRECTION('center_axis',(0.,0.,1.));
#9835=DIRECTION('ref_axis',(-1.,-1.01142816624385E-13,0.));
#9836=DIRECTION('',(-1.22464679914735E-16,-1.24014202614067E-29,1.));
#9837=DIRECTION('center_axis',(0.,0.,1.));
#9838=DIRECTION('ref_axis',(-1.,-1.01142816624385E-13,0.));
#9839=DIRECTION('',(-1.22464679914735E-16,-1.24014202614067E-29,1.));
#9840=DIRECTION('center_axis',(0.,0.,1.));
#9841=DIRECTION('ref_axis',(-1.,-1.01142816624385E-13,0.));
#9842=DIRECTION('',(-1.22464679914735E-16,-1.24014202614067E-29,1.));
#9843=DIRECTION('center_axis',(0.,0.,1.));
#9844=DIRECTION('ref_axis',(-1.,-1.01142816624385E-13,0.));
#9845=DIRECTION('',(-1.22464679914735E-16,-1.24014202614067E-29,1.));
#9846=DIRECTION('center_axis',(0.,0.,1.));
#9847=DIRECTION('ref_axis',(-1.,-1.01142816624385E-13,0.));
#9848=DIRECTION('',(-1.22464679914735E-16,-1.24014202614067E-29,1.));
#9849=DIRECTION('center_axis',(0.,0.,1.));
#9850=DIRECTION('ref_axis',(-1.,-1.01142816624385E-13,0.));
#9851=DIRECTION('',(-1.22464679914735E-16,-1.24014202614067E-29,1.));
#9852=DIRECTION('center_axis',(0.,0.,1.));
#9853=DIRECTION('ref_axis',(-1.,-1.01142816624385E-13,0.));
#9854=DIRECTION('',(-1.22464679914735E-16,-1.24014202614067E-29,1.));
#9855=DIRECTION('center_axis',(0.,0.,1.));
#9856=DIRECTION('ref_axis',(-1.,-1.01142816624385E-13,0.));
#9857=DIRECTION('',(-1.22464679914735E-16,-1.24014202614067E-29,1.));
#9858=DIRECTION('center_axis',(0.,0.,1.));
#9859=DIRECTION('ref_axis',(-1.,-1.01142816624385E-13,0.));
#9860=DIRECTION('',(-1.22464679914735E-16,-1.24014202614067E-29,1.));
#9861=DIRECTION('center_axis',(0.,0.,1.));
#9862=DIRECTION('ref_axis',(-1.,-1.01142816624385E-13,0.));
#9863=DIRECTION('',(-1.22464679914735E-16,-1.24014202614067E-29,1.));
#9864=DIRECTION('center_axis',(0.,0.,1.));
#9865=DIRECTION('ref_axis',(-1.,-1.01142816624385E-13,0.));
#9866=DIRECTION('',(-1.22464679914735E-16,-1.24014202614067E-29,1.));
#9867=DIRECTION('center_axis',(0.,0.,1.));
#9868=DIRECTION('ref_axis',(-1.,-1.01142816624385E-13,0.));
#9869=DIRECTION('',(-1.22464679914735E-16,-1.24014202614067E-29,1.));
#9870=DIRECTION('center_axis',(0.,0.,1.));
#9871=DIRECTION('ref_axis',(-1.,-1.01142816624385E-13,0.));
#9872=DIRECTION('',(-1.22464679914735E-16,-1.24014202614067E-29,1.));
#9873=DIRECTION('center_axis',(0.,0.,1.));
#9874=DIRECTION('ref_axis',(0.609237468266457,-0.792987835505865,0.));
#9875=DIRECTION('',(-1.22464679914735E-16,-1.24014202614067E-29,1.));
#9876=DIRECTION('center_axis',(0.,0.,1.));
#9877=DIRECTION('ref_axis',(-1.,-1.01142816624385E-13,0.));
#9878=DIRECTION('center_axis',(0.,0.,1.));
#9879=DIRECTION('ref_axis',(-1.,0.,0.));
#9880=DIRECTION('',(0.,0.,1.));
#9881=DIRECTION('center_axis',(0.,0.,-1.));
#9882=DIRECTION('ref_axis',(-1.,0.,0.));
#9883=DIRECTION('',(0.,0.,1.));
#9884=DIRECTION('center_axis',(0.,0.,-1.));
#9885=DIRECTION('ref_axis',(-1.,0.,0.));
#9886=DIRECTION('center_axis',(0.,0.,-1.));
#9887=DIRECTION('ref_axis',(-1.,0.,0.));
#9888=DIRECTION('center_axis',(0.,0.,1.));
#9889=DIRECTION('ref_axis',(-1.,0.,0.));
#9890=DIRECTION('',(0.,0.,1.));
#9891=DIRECTION('center_axis',(0.,0.,1.));
#9892=DIRECTION('ref_axis',(-1.,0.,0.));
#9893=DIRECTION('',(0.,0.,1.));
#9894=DIRECTION('center_axis',(0.,0.,1.));
#9895=DIRECTION('ref_axis',(-1.,0.,0.));
#9896=DIRECTION('',(0.,0.,1.));
#9897=DIRECTION('center_axis',(0.,0.,1.));
#9898=DIRECTION('ref_axis',(-1.,0.,0.));
#9899=DIRECTION('',(0.,0.,1.));
#9900=DIRECTION('center_axis',(0.,0.,1.));
#9901=DIRECTION('ref_axis',(-1.,0.,0.));
#9902=DIRECTION('',(0.,0.,1.));
#9903=DIRECTION('center_axis',(0.,0.,1.));
#9904=DIRECTION('ref_axis',(-1.,0.,0.));
#9905=DIRECTION('',(0.,0.,1.));
#9906=DIRECTION('center_axis',(0.,0.,1.));
#9907=DIRECTION('ref_axis',(-1.,0.,0.));
#9908=DIRECTION('',(0.,0.,1.));
#9909=DIRECTION('center_axis',(0.,0.,1.));
#9910=DIRECTION('ref_axis',(-1.,0.,0.));
#9911=DIRECTION('',(0.,0.,1.));
#9912=DIRECTION('center_axis',(0.,0.,1.));
#9913=DIRECTION('ref_axis',(-1.,0.,0.));
#9914=DIRECTION('',(0.,0.,1.));
#9915=DIRECTION('center_axis',(0.,0.,1.));
#9916=DIRECTION('ref_axis',(-1.,0.,0.));
#9917=DIRECTION('',(0.,0.,1.));
#9918=DIRECTION('center_axis',(0.,0.,1.));
#9919=DIRECTION('ref_axis',(-1.,0.,0.));
#9920=DIRECTION('',(0.,0.,1.));
#9921=DIRECTION('center_axis',(0.,0.,1.));
#9922=DIRECTION('ref_axis',(-1.,0.,0.));
#9923=DIRECTION('',(0.,0.,1.));
#9924=DIRECTION('center_axis',(0.,0.,1.));
#9925=DIRECTION('ref_axis',(-1.,0.,0.));
#9926=DIRECTION('',(0.,0.,1.));
#9927=DIRECTION('center_axis',(0.,0.,1.));
#9928=DIRECTION('ref_axis',(-1.,0.,0.));
#9929=DIRECTION('',(0.,0.,1.));
#9930=DIRECTION('center_axis',(0.,0.,1.));
#9931=DIRECTION('ref_axis',(-1.,0.,0.));
#9932=DIRECTION('',(0.,0.,1.));
#9933=DIRECTION('center_axis',(0.,0.,1.));
#9934=DIRECTION('ref_axis',(-0.937990854518778,-0.346660001787244,0.));
#9935=DIRECTION('',(0.,0.,1.));
#9936=DIRECTION('center_axis',(0.,0.,-1.));
#9937=DIRECTION('ref_axis',(-1.,0.,0.));
#9938=DIRECTION('center_axis',(0.,0.,1.));
#9939=DIRECTION('ref_axis',(-1.,-9.53632271029895E-14,0.));
#9940=DIRECTION('',(-1.22464679914735E-16,-1.16936246806304E-29,1.));
#9941=DIRECTION('center_axis',(0.,0.,-1.));
#9942=DIRECTION('ref_axis',(-1.,-9.53632271029895E-14,0.));
#9943=DIRECTION('center_axis',(0.,0.,1.));
#9944=DIRECTION('ref_axis',(-1.,-9.53632271029895E-14,0.));
#9945=DIRECTION('',(-1.22464679914735E-16,-1.16936246806304E-29,1.));
#9946=DIRECTION('center_axis',(0.,0.,1.));
#9947=DIRECTION('ref_axis',(-1.,-9.53632271029895E-14,0.));
#9948=DIRECTION('',(-1.22464679914735E-16,-1.16936246806304E-29,1.));
#9949=DIRECTION('center_axis',(0.,0.,1.));
#9950=DIRECTION('ref_axis',(-1.,-9.53632271029895E-14,0.));
#9951=DIRECTION('',(-1.22464679914735E-16,-1.16936246806304E-29,1.));
#9952=DIRECTION('center_axis',(0.,0.,1.));
#9953=DIRECTION('ref_axis',(-1.,-9.53632271029895E-14,0.));
#9954=DIRECTION('',(-1.22464679914735E-16,-1.16936246806304E-29,1.));
#9955=DIRECTION('center_axis',(0.,0.,1.));
#9956=DIRECTION('ref_axis',(-1.,-9.53632271029895E-14,0.));
#9957=DIRECTION('',(-1.22464679914735E-16,-1.16936246806304E-29,1.));
#9958=DIRECTION('center_axis',(0.,0.,1.));
#9959=DIRECTION('ref_axis',(-1.,-9.53632271029895E-14,0.));
#9960=DIRECTION('',(-1.22464679914735E-16,-1.16936246806304E-29,1.));
#9961=DIRECTION('center_axis',(0.,0.,1.));
#9962=DIRECTION('ref_axis',(-1.,-9.53632271029895E-14,0.));
#9963=DIRECTION('',(-1.22464679914735E-16,-1.16936246806304E-29,1.));
#9964=DIRECTION('center_axis',(0.,0.,1.));
#9965=DIRECTION('ref_axis',(-1.,-9.53632271029895E-14,0.));
#9966=DIRECTION('',(-1.22464679914735E-16,-1.16936246806304E-29,1.));
#9967=DIRECTION('center_axis',(0.,0.,1.));
#9968=DIRECTION('ref_axis',(-1.,-9.53632271029895E-14,0.));
#9969=DIRECTION('',(-1.22464679914735E-16,-1.16936246806304E-29,1.));
#9970=DIRECTION('center_axis',(0.,0.,1.));
#9971=DIRECTION('ref_axis',(-1.,-9.53632271029895E-14,0.));
#9972=DIRECTION('',(-1.22464679914735E-16,-1.16936246806304E-29,1.));
#9973=DIRECTION('center_axis',(0.,0.,1.));
#9974=DIRECTION('ref_axis',(-1.,-9.53632271029895E-14,0.));
#9975=DIRECTION('',(-1.22464679914735E-16,-1.16936246806304E-29,1.));
#9976=DIRECTION('center_axis',(0.,0.,1.));
#9977=DIRECTION('ref_axis',(-1.,-9.53632271029895E-14,0.));
#9978=DIRECTION('',(-1.22464679914735E-16,-1.16936246806304E-29,1.));
#9979=DIRECTION('center_axis',(0.,0.,1.));
#9980=DIRECTION('ref_axis',(-1.,-9.53632271029895E-14,0.));
#9981=DIRECTION('',(-1.22464679914735E-16,-1.16936246806304E-29,1.));
#9982=DIRECTION('center_axis',(0.,0.,1.));
#9983=DIRECTION('ref_axis',(-1.,-9.53632271029895E-14,0.));
#9984=DIRECTION('',(-1.22464679914735E-16,-1.16936246806304E-29,1.));
#9985=DIRECTION('center_axis',(0.,0.,1.));
#9986=DIRECTION('ref_axis',(-1.,-9.53632271029895E-14,0.));
#9987=DIRECTION('',(-1.22464679914735E-16,-1.16936246806304E-29,1.));
#9988=DIRECTION('center_axis',(0.,0.,1.));
#9989=DIRECTION('ref_axis',(0.609237469603756,-0.792987834478444,0.));
#9990=DIRECTION('',(-1.22464679914735E-16,-1.16936246806304E-29,1.));
#9991=DIRECTION('center_axis',(0.,0.,1.));
#9992=DIRECTION('ref_axis',(-1.,-9.53632271029895E-14,0.));
#9993=DIRECTION('center_axis',(0.,0.,1.));
#9994=DIRECTION('ref_axis',(1.,0.,0.));
#9995=DIRECTION('center_axis',(0.,0.,1.));
#9996=DIRECTION('ref_axis',(-1.,-9.53632271029895E-14,0.));
#9997=DIRECTION('center_axis',(0.,0.,1.));
#9998=DIRECTION('ref_axis',(-1.,0.,0.));
#9999=DIRECTION('center_axis',(0.,0.,1.));
#10000=DIRECTION('ref_axis',(1.,0.,0.));
#10001=DIRECTION('center_axis',(0.,0.,1.));
#10002=DIRECTION('ref_axis',(-1.,-1.01142816624385E-13,0.));
#10003=DIRECTION('center_axis',(0.,0.,1.));
#10004=DIRECTION('ref_axis',(-1.,0.,0.));
#10005=DIRECTION('center_axis',(0.,0.,1.));
#10006=DIRECTION('ref_axis',(1.,0.,0.));
#10007=DIRECTION('center_axis',(0.,0.,1.));
#10008=DIRECTION('ref_axis',(-1.,-1.09812200906474E-13,0.));
#10009=DIRECTION('center_axis',(0.,0.,1.));
#10010=DIRECTION('ref_axis',(-1.,0.,0.));
#10011=DIRECTION('center_axis',(0.,0.,1.));
#10012=DIRECTION('ref_axis',(1.,0.,0.));
#10013=DIRECTION('center_axis',(0.,0.,1.));
#10014=DIRECTION('ref_axis',(-1.,-9.82530218636873E-14,0.));
#10015=DIRECTION('center_axis',(0.,0.,1.));
#10016=DIRECTION('ref_axis',(-1.,0.,0.));
#10017=DIRECTION('center_axis',(0.,0.,1.));
#10018=DIRECTION('ref_axis',(-1.,0.,0.));
#10019=DIRECTION('center_axis',(0.,0.,1.));
#10020=DIRECTION('ref_axis',(-1.,0.,0.));
#10021=DIRECTION('center_axis',(0.,0.,1.));
#10022=DIRECTION('ref_axis',(-1.,0.,0.));
#10023=DIRECTION('center_axis',(0.,0.,1.));
#10024=DIRECTION('ref_axis',(-1.,0.,0.));
#10025=DIRECTION('center_axis',(0.,1.,0.));
#10026=DIRECTION('ref_axis',(-1.,0.,0.));
#10027=DIRECTION('',(-1.,0.,0.));
#10028=DIRECTION('',(0.,0.,1.));
#10029=DIRECTION('',(-1.,0.,0.));
#10030=DIRECTION('',(0.,0.,1.));
#10031=DIRECTION('center_axis',(-1.,0.,0.));
#10032=DIRECTION('ref_axis',(0.,-1.,0.));
#10033=DIRECTION('',(0.,-1.,0.));
#10034=DIRECTION('',(0.,-1.,0.));
#10035=DIRECTION('',(0.,0.,1.));
#10036=DIRECTION('center_axis',(0.,-1.,0.));
#10037=DIRECTION('ref_axis',(1.,0.,0.));
#10038=DIRECTION('',(1.,0.,0.));
#10039=DIRECTION('',(1.,0.,0.));
#10040=DIRECTION('',(0.,0.,1.));
#10041=DIRECTION('center_axis',(1.,0.,0.));
#10042=DIRECTION('ref_axis',(0.,1.,0.));
#10043=DIRECTION('',(0.,1.,0.));
#10044=DIRECTION('',(0.,1.,0.));
#10045=DIRECTION('center_axis',(0.,1.,0.));
#10046=DIRECTION('ref_axis',(-1.,0.,0.));
#10047=DIRECTION('',(1.,0.,0.));
#10048=DIRECTION('',(0.,0.,1.));
#10049=DIRECTION('',(1.,0.,0.));
#10050=DIRECTION('',(0.,0.,-1.));
#10051=DIRECTION('center_axis',(1.,0.,0.));
#10052=DIRECTION('ref_axis',(0.,1.,0.));
#10053=DIRECTION('',(0.,-1.,0.));
#10054=DIRECTION('',(0.,-1.,0.));
#10055=DIRECTION('',(0.,0.,-1.));
#10056=DIRECTION('center_axis',(0.,-1.,0.));
#10057=DIRECTION('ref_axis',(1.,0.,0.));
#10058=DIRECTION('',(-1.,0.,0.));
#10059=DIRECTION('',(-1.,0.,0.));
#10060=DIRECTION('',(0.,0.,1.));
#10061=DIRECTION('center_axis',(-1.,0.,0.));
#10062=DIRECTION('ref_axis',(0.,-1.,0.));
#10063=DIRECTION('',(0.,1.,0.));
#10064=DIRECTION('',(0.,1.,0.));
#10065=DIRECTION('center_axis',(0.,0.,1.));
#10066=DIRECTION('ref_axis',(1.,0.,0.));
#10067=DIRECTION('center_axis',(0.,0.,1.));
#10068=DIRECTION('ref_axis',(1.,0.,0.));
#11350=CARTESIAN_POINT('',(0.,0.,0.));
#11351=CARTESIAN_POINT('Origin',(-205.,95.,9.));
#11352=CARTESIAN_POINT('',(-202.486487043593,95.0006372934558,16.612583302492));
#11353=CARTESIAN_POINT('',(-202.484597865978,94.9962675362615,16.887416697508));
#11354=CARTESIAN_POINT('',(-202.4825,95.,9.));
#11355=CARTESIAN_POINT('',(-203.086534003335,96.6359872033749,17.));
#11356=CARTESIAN_POINT('Ctrl Pts',(-202.484597865978,94.9962675362615,16.887416697508));
#11357=CARTESIAN_POINT('Ctrl Pts',(-202.48977981228,95.5889553626798,16.9249444650054));
#11358=CARTESIAN_POINT('Ctrl Pts',(-202.700778171916,96.1848035603043,16.9624722325027));
#11359=CARTESIAN_POINT('Ctrl Pts',(-203.086534003335,96.6359872033749,17.));
#11360=CARTESIAN_POINT('',(-202.4825,95.,17.));
#11361=CARTESIAN_POINT('Origin',(-205.,95.,17.));
#11362=CARTESIAN_POINT('',(-202.4825,95.,18.));
#11363=CARTESIAN_POINT('',(-202.4825,95.,9.));
#11364=CARTESIAN_POINT('Origin',(-205.,95.,18.));
#11365=CARTESIAN_POINT('',(-206.917150800208,96.6387883530143,17.));
#11366=CARTESIAN_POINT('Origin',(-205.,95.,17.));
#11367=CARTESIAN_POINT('Ctrl Pts',(-206.917153830491,96.638790656604,17.));
#11368=CARTESIAN_POINT('Ctrl Pts',(-206.385184906259,97.2593583513323,16.9480939310855));
#11369=CARTESIAN_POINT('Ctrl Pts',(-205.522590916198,97.5988876213873,16.896187862171));
#11370=CARTESIAN_POINT('Ctrl Pts',(-204.710520946275,97.5049655781755,16.8442817932565));
#11371=CARTESIAN_POINT('Ctrl Pts',(-203.881814551752,97.4091194064428,16.7913123536551));
#11372=CARTESIAN_POINT('Ctrl Pts',(-203.105723496861,96.8618802537328,16.7383429140536));
#11373=CARTESIAN_POINT('Ctrl Pts',(-202.737493201107,96.1136066926246,16.6853734744522));
#11374=CARTESIAN_POINT('Ctrl Pts',(-202.568820177878,95.7708495506689,16.6611100837988));
#11375=CARTESIAN_POINT('Ctrl Pts',(-202.485725551784,95.3859108502911,16.6368466931454));
#11376=CARTESIAN_POINT('Ctrl Pts',(-202.486487043593,95.0006372934558,16.612583302492));
#11377=CARTESIAN_POINT('Origin',(-205.,95.,9.));
#11378=CARTESIAN_POINT('',(-202.482805429294,94.9976897526833,15.612583302492));
#11379=CARTESIAN_POINT('',(-202.478254054321,95.0000324001602,15.887416697508));
#11380=CARTESIAN_POINT('',(-202.4825,95.,9.));
#11381=CARTESIAN_POINT('Ctrl Pts',(-202.478254054321,95.0000324001602,15.887416697508));
#11382=CARTESIAN_POINT('Ctrl Pts',(-202.4781431837,95.835267846479,15.9404611607301));
#11383=CARTESIAN_POINT('Ctrl Pts',(-202.934422716347,96.6703686768054,15.9935056239521));
#11384=CARTESIAN_POINT('Ctrl Pts',(-203.637201874695,97.1217724188669,16.0465500871742));
#11385=CARTESIAN_POINT('Ctrl Pts',(-204.338987054902,97.5725377164795,16.0995195267756));
#11386=CARTESIAN_POINT('Ctrl Pts',(-205.286574244665,97.6406905263686,16.152488966377));
#11387=CARTESIAN_POINT('Ctrl Pts',(-206.045561328886,97.294827824976,16.2054584059785));
#11388=CARTESIAN_POINT('Ctrl Pts',(-206.804548413106,96.9489651235833,16.2584278455799));
#11389=CARTESIAN_POINT('Ctrl Pts',(-207.374935391785,96.189086910909,16.3113972851814));
#11390=CARTESIAN_POINT('Ctrl Pts',(-207.495329285435,95.3638523036021,16.3643667247828));
#11391=CARTESIAN_POINT('Ctrl Pts',(-207.615723179085,94.5386176962952,16.4173361643842));
#11392=CARTESIAN_POINT('Ctrl Pts',(-207.286123987708,93.6480266943556,16.4703056039857));
#11393=CARTESIAN_POINT('Ctrl Pts',(-206.657476699318,93.0996259784246,16.5232750435871));
#11394=CARTESIAN_POINT('Ctrl Pts',(-206.028829410928,92.5512252624936,16.5762444831885));
#11395=CARTESIAN_POINT('Ctrl Pts',(-205.101134025526,92.3450148325712,16.62921392279));
#11396=CARTESIAN_POINT('Ctrl Pts',(-204.299947458499,92.576953621889,16.6821833623914));
#11397=CARTESIAN_POINT('Ctrl Pts',(-203.498760891472,92.8088924112068,16.7351528019928));
#11398=CARTESIAN_POINT('Ctrl Pts',(-202.824083142821,93.4789804197649,16.7881222415943));
#11399=CARTESIAN_POINT('Ctrl Pts',(-202.584905412425,94.2765457081108,16.8410916811957));
#11400=CARTESIAN_POINT('Ctrl Pts',(-202.515180225313,94.5090522582447,16.8565333532998));
#11401=CARTESIAN_POINT('Ctrl Pts',(-202.482465633741,94.7523923556688,16.8719750254039));
#11402=CARTESIAN_POINT('Ctrl Pts',(-202.484597865978,94.9962675362615,16.887416697508));
#11403=CARTESIAN_POINT('Ctrl Pts',(-202.486487043593,95.0006372934558,16.612583302492));
#11404=CARTESIAN_POINT('Ctrl Pts',(-202.48738796554,94.5448196487217,16.583877253544));
#11405=CARTESIAN_POINT('Ctrl Pts',(-202.605664700594,94.0885332958007,16.5551712045959));
#11406=CARTESIAN_POINT('Ctrl Pts',(-202.838465118499,93.7010772441806,16.5264651556479));
#11407=CARTESIAN_POINT('Ctrl Pts',(-203.268036868263,92.9861293263514,16.4734957160465));
#11408=CARTESIAN_POINT('Ctrl Pts',(-204.087549904409,92.5055414601994,16.420526276445));
#11409=CARTESIAN_POINT('Ctrl Pts',(-204.921224621725,92.4794977627324,16.3675568368436));
#11410=CARTESIAN_POINT('Ctrl Pts',(-205.754899339041,92.4534540652654,16.3145873972421));
#11411=CARTESIAN_POINT('Ctrl Pts',(-206.602735737526,92.8819545364836,16.2616179576407));
#11412=CARTESIAN_POINT('Ctrl Pts',(-207.076148107766,93.5686324160268,16.2086485180393));
#11413=CARTESIAN_POINT('Ctrl Pts',(-207.549560478006,94.2553102955701,16.1556790784378));
#11414=CARTESIAN_POINT('Ctrl Pts',(-207.64854882,95.2001655834383,16.1027096388364));
#11415=CARTESIAN_POINT('Ctrl Pts',(-207.327709494231,95.970055069638,16.049740199235));
#11416=CARTESIAN_POINT('Ctrl Pts',(-207.006870168461,96.7399445558378,15.9967707596335));
#11417=CARTESIAN_POINT('Ctrl Pts',(-206.266203174927,97.3348682403689,15.9438013200321));
#11418=CARTESIAN_POINT('Ctrl Pts',(-205.445239637068,97.4821294064964,15.8908318804307));
#11419=CARTESIAN_POINT('Ctrl Pts',(-204.624276099208,97.6293905726238,15.8378624408292));
#11420=CARTESIAN_POINT('Ctrl Pts',(-203.723016017023,97.3289892203476,15.7848930012278));
#11421=CARTESIAN_POINT('Ctrl Pts',(-203.154585439598,96.7186213746173,15.7319235616264));
#11422=CARTESIAN_POINT('Ctrl Pts',(-202.727693676347,96.260234693386,15.6921434752482));
#11423=CARTESIAN_POINT('Ctrl Pts',(-202.488518438045,95.6270262725852,15.6523633888701));
#11424=CARTESIAN_POINT('Ctrl Pts',(-202.482805429294,94.9976897526833,15.612583302492));
#11425=CARTESIAN_POINT('Origin',(-205.,95.,9.));
#11426=CARTESIAN_POINT('',(-202.47847166618,95.0006753796333,14.612583302492));
#11427=CARTESIAN_POINT('',(-202.483904416421,95.0021895168216,14.887416697508));
#11428=CARTESIAN_POINT('',(-202.4825,95.,9.));
#11429=CARTESIAN_POINT('Ctrl Pts',(-202.483904416421,95.0021895168216,14.887416697508));
#11430=CARTESIAN_POINT('Ctrl Pts',(-202.481855095851,95.2491301525216,14.9030084168534));
#11431=CARTESIAN_POINT('Ctrl Pts',(-202.515258340335,95.4955283668393,14.9186001361987));
#11432=CARTESIAN_POINT('Ctrl Pts',(-202.586378614567,95.7305110407181,14.934191855544));
#11433=CARTESIAN_POINT('Ctrl Pts',(-202.82799411488,96.5288130288264,14.9871612951455));
#11434=CARTESIAN_POINT('Ctrl Pts',(-203.504921198234,97.1953624104036,15.0401307347469));
#11435=CARTESIAN_POINT('Ctrl Pts',(-204.306860479768,97.4246176783161,15.0931001743483));
#11436=CARTESIAN_POINT('Ctrl Pts',(-205.108799761302,97.6538729462285,15.1460696139498));
#11437=CARTESIAN_POINT('Ctrl Pts',(-206.035751241016,97.4458341004763,15.1990390535512));
#11438=CARTESIAN_POINT('Ctrl Pts',(-206.662805112391,96.8958629087621,15.2520084931526));
#11439=CARTESIAN_POINT('Ctrl Pts',(-207.289858983766,96.3458917170479,15.3049779327541));
#11440=CARTESIAN_POINT('Ctrl Pts',(-207.617015246803,95.4539881793718,15.3579473723555));
#11441=CARTESIAN_POINT('Ctrl Pts',(-207.494308184462,94.6290001862474,15.4109168119569));
#11442=CARTESIAN_POINT('Ctrl Pts',(-207.37160112212,93.8040121931229,15.4638862515584));
#11443=CARTESIAN_POINT('Ctrl Pts',(-206.799030734401,93.0459397445501,15.5168556911598));
#11444=CARTESIAN_POINT('Ctrl Pts',(-206.039058256267,92.7022701388405,15.5698251307613));
#11445=CARTESIAN_POINT('Ctrl Pts',(-205.279085778134,92.3586005331309,15.6227945703627));
#11446=CARTESIAN_POINT('Ctrl Pts',(-204.331711209586,92.4293337702846,15.6757640099641));
#11447=CARTESIAN_POINT('Ctrl Pts',(-203.631209544004,92.8820644793853,15.7287334495656));
#11448=CARTESIAN_POINT('Ctrl Pts',(-202.931700038648,93.3341539603135,15.7816278655464));
#11449=CARTESIAN_POINT('Ctrl Pts',(-202.478364611322,94.1671595901444,15.8345222815272));
#11450=CARTESIAN_POINT('Ctrl Pts',(-202.478254054321,95.0000324001602,15.887416697508));
#11451=CARTESIAN_POINT('Ctrl Pts',(-202.482805429294,94.9976897526833,15.612583302492));
#11452=CARTESIAN_POINT('Ctrl Pts',(-202.480911243101,94.7890290278569,15.5993939492687));
#11453=CARTESIAN_POINT('Ctrl Pts',(-202.504681520023,94.5807939404367,15.5862045960454));
#11454=CARTESIAN_POINT('Ctrl Pts',(-202.55578359808,94.3794975106792,15.5730152428221));
#11455=CARTESIAN_POINT('Ctrl Pts',(-202.761013406651,93.5710758316558,15.5200458032206));
#11456=CARTESIAN_POINT('Ctrl Pts',(-203.407074096456,92.8745668127933,15.4670763636192));
#11457=CARTESIAN_POINT('Ctrl Pts',(-204.197813528595,92.6092448276169,15.4141069240178));
#11458=CARTESIAN_POINT('Ctrl Pts',(-204.988552960733,92.3439228424405,15.3611374844163));
#11459=CARTESIAN_POINT('Ctrl Pts',(-205.923971135204,92.5097878909503,15.3081680448149));
#11460=CARTESIAN_POINT('Ctrl Pts',(-206.575278327948,93.0308090720576,15.2551986052134));
#11461=CARTESIAN_POINT('Ctrl Pts',(-207.226585520692,93.551830253165,15.202229165612));
#11462=CARTESIAN_POINT('Ctrl Pts',(-207.593781731709,94.4280075668699,15.1492597260106));
#11463=CARTESIAN_POINT('Ctrl Pts',(-207.508545912156,95.2577058854654,15.0962902864091));
#11464=CARTESIAN_POINT('Ctrl Pts',(-207.423310092601,96.0874042040608,15.0433208468077));
#11465=CARTESIAN_POINT('Ctrl Pts',(-206.885642242476,96.8706235275468,14.9903514072063));
#11466=CARTESIAN_POINT('Ctrl Pts',(-206.142006472617,97.2483406611404,14.9373819676048));
#11467=CARTESIAN_POINT('Ctrl Pts',(-205.398370702758,97.626057794734,14.8844125280034));
#11468=CARTESIAN_POINT('Ctrl Pts',(-204.448767013166,97.5982727384352,14.831443088402));
#11469=CARTESIAN_POINT('Ctrl Pts',(-203.728488344688,97.177721926406,14.7784736488005));
#11470=CARTESIAN_POINT('Ctrl Pts',(-203.008209676211,96.7571711143768,14.7255042091991));
#11471=CARTESIAN_POINT('Ctrl Pts',(-202.517256028848,95.9438545466172,14.6725347695977));
#11472=CARTESIAN_POINT('Ctrl Pts',(-202.480677851392,95.1105920315276,14.6195653299962));
#11473=CARTESIAN_POINT('Ctrl Pts',(-202.479070699274,95.0739805951826,14.6172379874948));
#11474=CARTESIAN_POINT('Ctrl Pts',(-202.47834071908,95.0373306531828,14.6149106449934));
#11475=CARTESIAN_POINT('Ctrl Pts',(-202.47847166618,95.0006753796333,14.612583302492));
#11476=CARTESIAN_POINT('Origin',(-205.,95.,9.));
#11477=CARTESIAN_POINT('',(-202.484820331358,95.0019240783679,13.612583302492));
#11478=CARTESIAN_POINT('',(-202.48602791266,94.998843140303,13.887416697508));
#11479=CARTESIAN_POINT('',(-202.4825,95.,9.));
#11480=CARTESIAN_POINT('Ctrl Pts',(-202.48602791266,94.998843140303,13.887416697508));
#11481=CARTESIAN_POINT('Ctrl Pts',(-202.488072688334,95.4925836353709,13.9185251125781));
#11482=CARTESIAN_POINT('Ctrl Pts',(-202.628459938899,95.9873972957536,13.9496335276481));
#11483=CARTESIAN_POINT('Ctrl Pts',(-202.899511357491,96.3954074594928,13.9807419427182));
#11484=CARTESIAN_POINT('Ctrl Pts',(-203.361040551879,97.0901413337929,14.0337113823196));
#11485=CARTESIAN_POINT('Ctrl Pts',(-204.201405965845,97.5332047692011,14.0866808219211));
#11486=CARTESIAN_POINT('Ctrl Pts',(-205.035388792576,97.521499975804,14.1396502615225));
#11487=CARTESIAN_POINT('Ctrl Pts',(-205.869371619307,97.509795182407,14.1926197011239));
#11488=CARTESIAN_POINT('Ctrl Pts',(-206.696971858804,97.0433221602047,14.2455891407254));
#11489=CARTESIAN_POINT('Ctrl Pts',(-207.138822180752,96.335909509144,14.2985585803268));
#11490=CARTESIAN_POINT('Ctrl Pts',(-207.580672502701,95.6284968580833,14.3515280199282));
#11491=CARTESIAN_POINT('Ctrl Pts',(-207.636772907101,94.6801445781641,14.4044974595297));
#11492=CARTESIAN_POINT('Ctrl Pts',(-207.281407293431,93.9255721097145,14.4574668991311));
#11493=CARTESIAN_POINT('Ctrl Pts',(-206.92604167976,93.1709996412648,14.5104363387325));
#11494=CARTESIAN_POINT('Ctrl Pts',(-206.159210048017,92.6102069842847,14.563405778334));
#11495=CARTESIAN_POINT('Ctrl Pts',(-205.332423709386,92.5002582451323,14.6163752179354));
#11496=CARTESIAN_POINT('Ctrl Pts',(-204.505637370754,92.3903095059799,14.6693446575369));
#11497=CARTESIAN_POINT('Ctrl Pts',(-203.618896325232,92.7312046846553,14.7223140971383));
#11498=CARTESIAN_POINT('Ctrl Pts',(-203.078677761108,93.3666795713128,14.7752835367397));
#11499=CARTESIAN_POINT('Ctrl Pts',(-202.697474212062,93.8151004479916,14.8126612569958));
#11500=CARTESIAN_POINT('Ctrl Pts',(-202.488817212071,94.410203617343,14.8500389772519));
#11501=CARTESIAN_POINT('Ctrl Pts',(-202.483904416421,95.0021895168216,14.887416697508));
#11502=CARTESIAN_POINT('Ctrl Pts',(-202.47847166618,95.0006753796333,14.612583302492));
#11503=CARTESIAN_POINT('Ctrl Pts',(-202.481321025821,94.2030704198136,14.561941205392));
#11504=CARTESIAN_POINT('Ctrl Pts',(-202.891803295554,93.402941071284,14.5112991082919));
#11505=CARTESIAN_POINT('Ctrl Pts',(-203.542553765119,92.9420726165712,14.4606570111919));
#11506=CARTESIAN_POINT('Ctrl Pts',(-204.223210563852,92.4600241791239,14.4076875715905));
#11507=CARTESIAN_POINT('Ctrl Pts',(-205.166726868867,92.3491357666491,14.354718131989));
#11508=CARTESIAN_POINT('Ctrl Pts',(-205.940600088161,92.6602380168317,14.3017486923876));
#11509=CARTESIAN_POINT('Ctrl Pts',(-206.714473307454,92.9713402670144,14.2487792527862));
#11510=CARTESIAN_POINT('Ctrl Pts',(-207.318703441026,93.7044331798545,14.1958098131847));
#11511=CARTESIAN_POINT('Ctrl Pts',(-207.476314767743,94.523471056521,14.1428403735833));
#11512=CARTESIAN_POINT('Ctrl Pts',(-207.63392609446,95.3425089331874,14.0898709339819));
#11513=CARTESIAN_POINT('Ctrl Pts',(-207.344918614323,96.2474917736803,14.0369014943804));
#11514=CARTESIAN_POINT('Ctrl Pts',(-206.741771743353,96.8235805034484,13.983932054779));
#11515=CARTESIAN_POINT('Ctrl Pts',(-206.138624872383,97.3996692332166,13.9309626151776));
#11516=CARTESIAN_POINT('Ctrl Pts',(-205.221338610581,97.64686385226,13.8779931755761));
#11517=CARTESIAN_POINT('Ctrl Pts',(-204.410391853126,97.4518517276016,13.8250237359747));
#11518=CARTESIAN_POINT('Ctrl Pts',(-203.599445095671,97.2568396029432,13.7720542963732));
#11519=CARTESIAN_POINT('Ctrl Pts',(-202.894837842562,96.619620734583,13.7190848567718));
#11520=CARTESIAN_POINT('Ctrl Pts',(-202.619558121519,95.8322926912433,13.6661154171704));
#11521=CARTESIAN_POINT('Ctrl Pts',(-202.526823482411,95.5670621770531,13.6482713789442));
#11522=CARTESIAN_POINT('Ctrl Pts',(-202.482810749722,95.2847966380167,13.6304273407181));
#11523=CARTESIAN_POINT('Ctrl Pts',(-202.484820331358,95.0019240783679,13.612583302492));
#11524=CARTESIAN_POINT('Origin',(-205.,95.,9.));
#11525=CARTESIAN_POINT('',(-202.485427355471,94.9983727942933,12.612583302492));
#11526=CARTESIAN_POINT('',(-202.479664315357,94.9983441169425,12.887416697508));
#11527=CARTESIAN_POINT('',(-202.4825,95.,9.));
#11528=CARTESIAN_POINT('Ctrl Pts',(-202.479664315357,94.9983441169425,12.887416697508));
#11529=CARTESIAN_POINT('Ctrl Pts',(-202.485253167408,95.7336004827625,12.9340418083028));
#11530=CARTESIAN_POINT('Ctrl Pts',(-202.825737604096,96.473362659355,12.9806669190976));
#11531=CARTESIAN_POINT('Ctrl Pts',(-203.391055625289,96.9417807577727,13.0272920298924));
#11532=CARTESIAN_POINT('Ctrl Pts',(-204.033297075631,97.4739370089732,13.0802614694938));
#11533=CARTESIAN_POINT('Ctrl Pts',(-204.965721673696,97.6558809958686,13.1332309090952));
#11534=CARTESIAN_POINT('Ctrl Pts',(-205.760911194526,97.4042106118059,13.1862003486967));
#11535=CARTESIAN_POINT('Ctrl Pts',(-206.556100715355,97.1525402277431,13.2391697882981));
#11536=CARTESIAN_POINT('Ctrl Pts',(-207.214055158948,96.4672554727222,13.2921392278995));
#11537=CARTESIAN_POINT('Ctrl Pts',(-207.433171885202,95.6624870484612,13.345108667501));
#11538=CARTESIAN_POINT('Ctrl Pts',(-207.652288611455,94.8577186242001,13.3980781071024));
#11539=CARTESIAN_POINT('Ctrl Pts',(-207.432567620369,93.9334665306991,13.4510475467038));
#11540=CARTESIAN_POINT('Ctrl Pts',(-206.874727786515,93.3134027632356,13.5040169863053));
#11541=CARTESIAN_POINT('Ctrl Pts',(-206.316887952661,92.6933389957721,13.5569864259067));
#11542=CARTESIAN_POINT('Ctrl Pts',(-205.420929276038,92.3774635543461,13.6099558655081));
#11543=CARTESIAN_POINT('Ctrl Pts',(-204.597554206738,92.5105719746145,13.6629253051096));
#11544=CARTESIAN_POINT('Ctrl Pts',(-203.774179137438,92.6436803948829,13.715894744711));
#11545=CARTESIAN_POINT('Ctrl Pts',(-203.023387675461,93.2257726768456,13.7688641843124));
#11546=CARTESIAN_POINT('Ctrl Pts',(-202.689338431877,93.990020974423,13.8218336239139));
#11547=CARTESIAN_POINT('Ctrl Pts',(-202.551472923697,94.3054339919501,13.8436946484453));
#11548=CARTESIAN_POINT('Ctrl Pts',(-202.484590973778,94.6518735807638,13.8655556729767));
#11549=CARTESIAN_POINT('Ctrl Pts',(-202.48602791266,94.998843140303,13.887416697508));
#11550=CARTESIAN_POINT('Ctrl Pts',(-202.484820331358,95.0019240783679,13.612583302492));
#11551=CARTESIAN_POINT('Ctrl Pts',(-202.488776126603,94.4450987639516,13.5774579011167));
#11552=CARTESIAN_POINT('Ctrl Pts',(-202.671062063926,93.8859213280996,13.5423324997414));
#11553=CARTESIAN_POINT('Ctrl Pts',(-203.011086898641,93.4496970181517,13.5072070983661));
#11554=CARTESIAN_POINT('Ctrl Pts',(-203.523847585785,92.7918666067188,13.4542376587646));
#11555=CARTESIAN_POINT('Ctrl Pts',(-204.395321149052,92.4136430021722,13.4012682191632));
#11556=CARTESIAN_POINT('Ctrl Pts',(-205.2260289773,92.4884017912889,13.3482987795618));
#11557=CARTESIAN_POINT('Ctrl Pts',(-206.056736805549,92.5631605804057,13.2953293399603));
#11558=CARTESIAN_POINT('Ctrl Pts',(-206.84667889878,93.0909017631857,13.2423599003589));
#11559=CARTESIAN_POINT('Ctrl Pts',(-207.233750215907,93.8297117306135,13.1893904607575));
#11560=CARTESIAN_POINT('Ctrl Pts',(-207.620821533034,94.5685216980413,13.136421021156));
#11561=CARTESIAN_POINT('Ctrl Pts',(-207.605022074058,95.5184004501168,13.0834515815546));
#11562=CARTESIAN_POINT('Ctrl Pts',(-207.193594222707,96.2439288752151,13.0304821419532));
#11563=CARTESIAN_POINT('Ctrl Pts',(-206.782166371356,96.9694573003133,12.9775127023517));
#11564=CARTESIAN_POINT('Ctrl Pts',(-205.975110127631,97.4706353984343,12.9245432627503));
#11565=CARTESIAN_POINT('Ctrl Pts',(-205.142375563491,97.5177259301682,12.8715738231488));
#11566=CARTESIAN_POINT('Ctrl Pts',(-204.309640999352,97.564816461902,12.8186043835474));
#11567=CARTESIAN_POINT('Ctrl Pts',(-203.451228114797,97.1578194272488,12.765634943946));
#11568=CARTESIAN_POINT('Ctrl Pts',(-202.960628578963,96.483299992439,12.7126655043445));
#11569=CARTESIAN_POINT('Ctrl Pts',(-202.65164361113,96.058480255272,12.6793047703937));
#11570=CARTESIAN_POINT('Ctrl Pts',(-202.488556167955,95.5275445869965,12.6459440364428));
#11571=CARTESIAN_POINT('Ctrl Pts',(-202.485427355471,94.9983727942933,12.612583302492));
#11572=CARTESIAN_POINT('Origin',(-205.,95.,9.));
#11573=CARTESIAN_POINT('',(-202.478890863588,94.9988537196689,11.612583302492));
#11574=CARTESIAN_POINT('',(-202.480886672631,95.0021035940924,11.887416697508));
#11575=CARTESIAN_POINT('',(-202.4825,95.,9.));
#11576=CARTESIAN_POINT('Ctrl Pts',(-202.480886672631,95.0021035940924,11.887416697508));
#11577=CARTESIAN_POINT('Ctrl Pts',(-202.479589474908,95.146930289923,11.8965890644261));
#11578=CARTESIAN_POINT('Ctrl Pts',(-202.491001904373,95.2915526532226,11.9057614313441));
#11579=CARTESIAN_POINT('Ctrl Pts',(-202.515848826212,95.4338288347626,11.9149337982622));
#11580=CARTESIAN_POINT('Ctrl Pts',(-202.659337146883,96.2554585920688,11.9679032378636));
#11581=CARTESIAN_POINT('Ctrl Pts',(-203.250857617326,96.998844614645,12.0208726774651));
#11582=CARTESIAN_POINT('Ctrl Pts',(-204.019260559541,97.3232229040773,12.0738421170665));
#11583=CARTESIAN_POINT('Ctrl Pts',(-204.787663501755,97.6476011935096,12.1268115566679));
#11584=CARTESIAN_POINT('Ctrl Pts',(-205.732948915742,97.552971749798,12.1797809962694));
#11585=CARTESIAN_POINT('Ctrl Pts',(-206.42180325036,97.0827121811151,12.2327504358708));
#11586=CARTESIAN_POINT('Ctrl Pts',(-207.110657584977,96.6124526124322,12.2857198754723));
#11587=CARTESIAN_POINT('Ctrl Pts',(-207.543080840225,95.766562918778,12.3386893150737));
#11588=CARTESIAN_POINT('Ctrl Pts',(-207.52085261245,94.932794208552,12.3916587546751));
#11589=CARTESIAN_POINT('Ctrl Pts',(-207.498624384675,94.0990254983261,12.4446281942766));
#11590=CARTESIAN_POINT('Ctrl Pts',(-207.021744673877,93.2773777715286,12.497597633878));
#11591=CARTESIAN_POINT('Ctrl Pts',(-206.308812474494,92.844489754439,12.5505670734794));
#11592=CARTESIAN_POINT('Ctrl Pts',(-205.595880275112,92.4116017373494,12.6035365130809));
#11593=CARTESIAN_POINT('Ctrl Pts',(-204.646895587144,92.3674734299677,12.6565059526823));
#11594=CARTESIAN_POINT('Ctrl Pts',(-203.89686768825,92.7323330017727,12.7094753922837));
#11595=CARTESIAN_POINT('Ctrl Pts',(-203.146839789356,93.0971925735776,12.7624448318852));
#11596=CARTESIAN_POINT('Ctrl Pts',(-202.595768679535,93.8710400245692,12.8154142714866));
#11597=CARTESIAN_POINT('Ctrl Pts',(-202.496262275933,94.6991480078178,12.868383711088));
#11598=CARTESIAN_POINT('Ctrl Pts',(-202.484344057662,94.7983332998029,12.8747280398947));
#11599=CARTESIAN_POINT('Ctrl Pts',(-202.478903834267,94.8982969950711,12.8810723687014));
#11600=CARTESIAN_POINT('Ctrl Pts',(-202.479664315357,94.9983441169425,12.887416697508));
#11601=CARTESIAN_POINT('Ctrl Pts',(-202.485427355471,94.9983727942933,12.612583302492));
#11602=CARTESIAN_POINT('Ctrl Pts',(-202.483588308311,94.6873372536185,12.5929745968414));
#11603=CARTESIAN_POINT('Ctrl Pts',(-202.537012246085,94.3769111019385,12.5733658911908));
#11604=CARTESIAN_POINT('Ctrl Pts',(-202.648554519612,94.0890012001821,12.5537571855402));
#11605=CARTESIAN_POINT('Ctrl Pts',(-202.949866183209,93.3112636777014,12.5007877459388));
#11606=CARTESIAN_POINT('Ctrl Pts',(-203.675275697519,92.6978304677061,12.4478183063374));
#11607=CARTESIAN_POINT('Ctrl Pts',(-204.492259395059,92.5298959255516,12.3948488667359));
#11608=CARTESIAN_POINT('Ctrl Pts',(-205.309243092599,92.3619613833971,12.3418794271345));
#11609=CARTESIAN_POINT('Ctrl Pts',(-206.217800973369,92.6395255090834,12.2889099875331));
#11610=CARTESIAN_POINT('Ctrl Pts',(-206.801455182205,93.2353544585335,12.2359405479316));
#11611=CARTESIAN_POINT('Ctrl Pts',(-207.385109391041,93.8311834079836,12.1829711083302));
#11612=CARTESIAN_POINT('Ctrl Pts',(-207.643859927944,94.7452771811977,12.1300016687287));
#11613=CARTESIAN_POINT('Ctrl Pts',(-207.459096992797,95.5586203008532,12.0770322291273));
#11614=CARTESIAN_POINT('Ctrl Pts',(-207.274334057651,96.3719634205086,12.0240627895259));
#11615=CARTESIAN_POINT('Ctrl Pts',(-206.646057650456,97.0845558866056,11.9710933499244));
#11616=CARTESIAN_POINT('Ctrl Pts',(-205.862266165212,97.3697492949344,11.918123910323));
#11617=CARTESIAN_POINT('Ctrl Pts',(-205.078474679968,97.6549427032632,11.8651544707216));
#11618=CARTESIAN_POINT('Ctrl Pts',(-204.139168116676,97.5127370538238,11.8121850311201));
#11619=CARTESIAN_POINT('Ctrl Pts',(-203.474919354731,97.0083186216177,11.7592155915187));
#11620=CARTESIAN_POINT('Ctrl Pts',(-202.86198532346,96.5428676628624,11.7103381618431));
#11621=CARTESIAN_POINT('Ctrl Pts',(-202.483252930993,95.7690057922765,11.6614607321676));
#11622=CARTESIAN_POINT('Ctrl Pts',(-202.478890863588,94.9988537196689,11.612583302492));
#11623=CARTESIAN_POINT('Origin',(-205.,95.,9.));
#11624=CARTESIAN_POINT('',(-202.481958520358,95.002283592634,10.612583302492));
#11625=CARTESIAN_POINT('',(-202.486464188569,95.0004666863557,10.887416697508));
#11626=CARTESIAN_POINT('',(-202.4825,95.,9.));
#11627=CARTESIAN_POINT('Ctrl Pts',(-202.486464188569,95.0004666863557,10.887416697508));
#11628=CARTESIAN_POINT('Ctrl Pts',(-202.485815967357,95.3924916278335,10.9121057601508));
#11629=CARTESIAN_POINT('Ctrl Pts',(-202.571975294708,95.7842468732566,10.9367948227936));
#11630=CARTESIAN_POINT('Ctrl Pts',(-202.746434438658,96.1316610680036,10.9614838854364));
#11631=CARTESIAN_POINT('Ctrl Pts',(-203.12072985935,96.8770249350567,11.0144533250378));
#11632=CARTESIAN_POINT('Ctrl Pts',(-203.901469877197,97.4182866740021,11.0674227646392));
#11633=CARTESIAN_POINT('Ctrl Pts',(-204.730767631102,97.5073349284926,11.1203922042407));
#11634=CARTESIAN_POINT('Ctrl Pts',(-205.560065385007,97.5963831829831,11.1733616438421));
#11635=CARTESIAN_POINT('Ctrl Pts',(-206.437920874971,97.2332179530186,11.2263310834435));
#11636=CARTESIAN_POINT('Ctrl Pts',(-206.961930050197,96.5843121505036,11.279300523045));
#11637=CARTESIAN_POINT('Ctrl Pts',(-207.485939225424,95.9354063479886,11.3322699626464));
#11638=CARTESIAN_POINT('Ctrl Pts',(-207.656102085915,95.000759972923,11.3852394022478));
#11639=CARTESIAN_POINT('Ctrl Pts',(-207.394416927358,94.2088097004623,11.4382088418493));
#11640=CARTESIAN_POINT('Ctrl Pts',(-207.132731768801,93.4168594280015,11.4911782814507));
#11641=CARTESIAN_POINT('Ctrl Pts',(-206.439198591197,92.7676052581456,11.5441477210522));
#11642=CARTESIAN_POINT('Ctrl Pts',(-205.63172912742,92.5586616740667,11.5971171606536));
#11643=CARTESIAN_POINT('Ctrl Pts',(-204.824259663643,92.3497180899878,11.650086600255));
#11644=CARTESIAN_POINT('Ctrl Pts',(-203.902853913694,92.581085091686,11.7030560398565));
#11645=CARTESIAN_POINT('Ctrl Pts',(-203.289879124169,93.1467053385531,11.7560254794579));
#11646=CARTESIAN_POINT('Ctrl Pts',(-202.783049117812,93.6143808746666,11.7998225521413));
#11647=CARTESIAN_POINT('Ctrl Pts',(-202.487080653257,94.3105715849115,11.8436196248247));
#11648=CARTESIAN_POINT('Ctrl Pts',(-202.480886672631,95.0021035940924,11.887416697508));
#11649=CARTESIAN_POINT('Ctrl Pts',(-202.478890863588,94.9988537196689,11.612583302492));
#11650=CARTESIAN_POINT('Ctrl Pts',(-202.478525672062,94.9343767218714,11.6084912925661));
#11651=CARTESIAN_POINT('Ctrl Pts',(-202.480784445636,94.8699257260826,11.6043992826403));
#11652=CARTESIAN_POINT('Ctrl Pts',(-202.485749434321,94.8056838825638,11.6003072727144));
#11653=CARTESIAN_POINT('Ctrl Pts',(-202.550019236455,93.9740987906889,11.547337833113));
#11654=CARTESIAN_POINT('Ctrl Pts',(-203.067749801321,93.1775598219119,11.4943683935115));
#11655=CARTESIAN_POINT('Ctrl Pts',(-203.801616331267,92.7811959881444,11.4413989539101));
#11656=CARTESIAN_POINT('Ctrl Pts',(-204.535482861214,92.384832154377,11.3884295143086));
#11657=CARTESIAN_POINT('Ctrl Pts',(-205.485485356242,92.3886434556191,11.3354600747072));
#11658=CARTESIAN_POINT('Ctrl Pts',(-206.216147981621,92.7908828126805,11.2824906351058));
#11659=CARTESIAN_POINT('Ctrl Pts',(-206.946810607,93.1931221697419,11.2295211955043));
#11660=CARTESIAN_POINT('Ctrl Pts',(-207.45813336273,93.9937895826225,11.1765517559029));
#11661=CARTESIAN_POINT('Ctrl Pts',(-207.515728755059,94.825863583705,11.1235823163015));
#11662=CARTESIAN_POINT('Ctrl Pts',(-207.573324147388,95.6579375847875,11.0706128767));
#11663=CARTESIAN_POINT('Ctrl Pts',(-207.177192176316,96.5214181740719,11.0176434370986));
#11664=CARTESIAN_POINT('Ctrl Pts',(-206.508917523639,97.0204906749021,10.9646739974972));
#11665=CARTESIAN_POINT('Ctrl Pts',(-205.840642870963,97.5195631757323,10.9117045578957));
#11666=CARTESIAN_POINT('Ctrl Pts',(-204.900225536682,97.6542275881084,10.8587351182943));
#11667=CARTESIAN_POINT('Ctrl Pts',(-204.118747571406,97.3627544979554,10.8057656786929));
#11668=CARTESIAN_POINT('Ctrl Pts',(-203.33726960613,97.0712814078023,10.7527962390914));
#11669=CARTESIAN_POINT('Ctrl Pts',(-202.714731009859,96.3536708151202,10.69982679949));
#11670=CARTESIAN_POINT('Ctrl Pts',(-202.536499996132,95.5388714053017,10.6468573598885));
#11671=CARTESIAN_POINT('Ctrl Pts',(-202.498058333415,95.3631318219437,10.6354326740897));
#11672=CARTESIAN_POINT('Ctrl Pts',(-202.480285767457,95.1828710349325,10.6240079882908));
#11673=CARTESIAN_POINT('Ctrl Pts',(-202.481958520358,95.002283592634,10.612583302492));
#11674=CARTESIAN_POINT('Origin',(-205.,95.,9.));
#11675=CARTESIAN_POINT('',(-202.486537867015,94.9998805722871,9.61258330249198));
#11676=CARTESIAN_POINT('',(-202.482602635909,94.9976869505601,9.88741669750804));
#11677=CARTESIAN_POINT('',(-202.4825,95.,9.));
#11678=CARTESIAN_POINT('Ctrl Pts',(-202.482602635909,94.9976869505601,9.88741669750804));
#11679=CARTESIAN_POINT('Ctrl Pts',(-202.488423732856,95.6336264814084,9.92762245587553));
#11680=CARTESIAN_POINT('Ctrl Pts',(-202.733269733893,96.273556587542,9.96782821424303));
#11681=CARTESIAN_POINT('Ctrl Pts',(-203.168433611194,96.7333721687788,10.0080339726105));
#11682=CARTESIAN_POINT('Ctrl Pts',(-203.741744192846,97.3391603604975,10.061003412212));
#11683=CARTESIAN_POINT('Ctrl Pts',(-204.645389190247,97.6323240761667,10.1139728518134));
#11684=CARTESIAN_POINT('Ctrl Pts',(-205.465142786516,97.4784787068388,10.1669422914148));
#11685=CARTESIAN_POINT('Ctrl Pts',(-206.284896382785,97.3246333375108,10.2199117310163));
#11686=CARTESIAN_POINT('Ctrl Pts',(-207.020758577922,96.7237788831858,10.2728811706177));
#11687=CARTESIAN_POINT('Ctrl Pts',(-207.335414253965,95.9513436679131,10.3258506102191));
#11688=CARTESIAN_POINT('Ctrl Pts',(-207.650069930008,95.1789084526404,10.3788200498206));
#11689=CARTESIAN_POINT('Ctrl Pts',(-207.543519086958,94.2348924764201,10.431789489422));
#11690=CARTESIAN_POINT('Ctrl Pts',(-207.064604035821,93.552027387216,10.4847589290234));
#11691=CARTESIAN_POINT('Ctrl Pts',(-206.585688984684,92.869162298012,10.5377283686249));
#11692=CARTESIAN_POINT('Ctrl Pts',(-205.734409725459,92.4474480958241,10.5906978082263));
#11693=CARTESIAN_POINT('Ctrl Pts',(-204.900987913289,92.480196214229,10.6436672478278));
#11694=CARTESIAN_POINT('Ctrl Pts',(-204.067566101119,92.5129443326339,10.6966366874292));
#11695=CARTESIAN_POINT('Ctrl Pts',(-203.252001736004,93.0001547716316,10.7496061270306));
#11696=CARTESIAN_POINT('Ctrl Pts',(-202.828144965216,93.7184929887108,10.8025755666321));
#11697=CARTESIAN_POINT('Ctrl Pts',(-202.601847890061,94.1020136699879,10.8308559435907));
#11698=CARTESIAN_POINT('Ctrl Pts',(-202.487206701174,94.5514171099257,10.8591363205494));
#11699=CARTESIAN_POINT('Ctrl Pts',(-202.486464188569,95.0004666863557,10.887416697508));
#11700=CARTESIAN_POINT('Ctrl Pts',(-202.481958520358,95.002283592634,10.612583302492));
#11701=CARTESIAN_POINT('Ctrl Pts',(-202.488041322869,94.3455950007355,10.5710385486894));
#11702=CARTESIAN_POINT('Ctrl Pts',(-202.751257777578,93.684586908207,10.5294937948868));
#11703=CARTESIAN_POINT('Ctrl Pts',(-203.212761690374,93.2209570311217,10.4879490410842));
#11704=CARTESIAN_POINT('Ctrl Pts',(-203.801177829528,92.6298302937148,10.4349796014828));
#11705=CARTESIAN_POINT('Ctrl Pts',(-204.711933539022,92.3595650458559,10.3820101618814));
#11706=CARTESIAN_POINT('Ctrl Pts',(-205.527543491288,92.5340493668139,10.3290407222799));
#11707=CARTESIAN_POINT('Ctrl Pts',(-206.343153443554,92.7085336877719,10.2760712826785));
#11708=CARTESIAN_POINT('Ctrl Pts',(-207.063617638591,93.3277675775469,10.2231018430771));
#11709=CARTESIAN_POINT('Ctrl Pts',(-207.358679315634,94.1078976815906,10.1701324034756));
#11710=CARTESIAN_POINT('Ctrl Pts',(-207.653740992677,94.8880277856344,10.1171629638742));
#11711=CARTESIAN_POINT('Ctrl Pts',(-207.523400151727,95.8290541039469,10.0641935242728));
#11712=CARTESIAN_POINT('Ctrl Pts',(-207.027404305878,96.499615431042,10.0112240846713));
#11713=CARTESIAN_POINT('Ctrl Pts',(-206.531408460029,97.1701767581371,9.95825464506989));
#11714=CARTESIAN_POINT('Ctrl Pts',(-205.669757609282,97.5702730940147,9.90528520546845));
#11715=CARTESIAN_POINT('Ctrl Pts',(-204.837427688372,97.5165025142056,9.85231576586701));
#11716=CARTESIAN_POINT('Ctrl Pts',(-204.005097767462,97.4627319343966,9.79934632626558));
#11717=CARTESIAN_POINT('Ctrl Pts',(-203.202088776389,96.9550944389009,9.74637688666414));
#11718=CARTESIAN_POINT('Ctrl Pts',(-202.796495549129,96.226288218774,9.69340744706271));
#11719=CARTESIAN_POINT('Ctrl Pts',(-202.590202222992,95.8556019026464,9.66646606553913));
#11720=CARTESIAN_POINT('Ctrl Pts',(-202.48671858869,95.427700220413,9.63952468401556));
#11721=CARTESIAN_POINT('Ctrl Pts',(-202.486537867015,94.9998805722871,9.61258330249198));
#11722=CARTESIAN_POINT('Origin',(-205.,95.,9.));
#11723=CARTESIAN_POINT('',(-202.481519189143,94.9977697596226,8.61258330249198));
#11724=CARTESIAN_POINT('',(-202.478555055026,95.000793452331,8.88741669750803));
#11725=CARTESIAN_POINT('',(-202.4825,95.,9.));
#11726=CARTESIAN_POINT('Ctrl Pts',(-202.478555055026,95.000793452331,8.88741669750803));
#11727=CARTESIAN_POINT('Ctrl Pts',(-202.478376198151,95.0441568163808,8.89016971199881));
#11728=CARTESIAN_POINT('Ctrl Pts',(-202.479397808956,95.0875115778544,8.89292272648959));
#11729=CARTESIAN_POINT('Ctrl Pts',(-202.481646333745,95.1308026137449,8.89567574098038));
#11730=CARTESIAN_POINT('Ctrl Pts',(-202.524909127459,95.9637448007781,8.94864518058181));
#11731=CARTESIAN_POINT('Ctrl Pts',(-203.022372703672,96.7730959210315,9.00161462018325));
#11732=CARTESIAN_POINT('Ctrl Pts',(-203.746002539071,97.187853943956,9.05458405978468));
#11733=CARTESIAN_POINT('Ctrl Pts',(-204.46963237447,97.6026119668805,9.10755349938612));
#11734=CARTESIAN_POINT('Ctrl Pts',(-205.419428469055,97.6227768924762,9.16052293898755));
#11735=CARTESIAN_POINT('Ctrl Pts',(-206.160009600906,97.2391052315395,9.21349237858899));
#11736=CARTESIAN_POINT('Ctrl Pts',(-206.900590732757,96.8554335706029,9.26646181819042));
#11737=CARTESIAN_POINT('Ctrl Pts',(-207.431956901874,96.0679253231338,9.31943125779186));
#11738=CARTESIAN_POINT('Ctrl Pts',(-207.510532825818,95.2375698688638,9.3724006973933));
#11739=CARTESIAN_POINT('Ctrl Pts',(-207.589108749762,94.4072144145938,9.42537013699473));
#11740=CARTESIAN_POINT('Ctrl Pts',(-207.214894428534,93.5340117535228,9.47833957659617));
#11741=CARTESIAN_POINT('Ctrl Pts',(-206.559427615726,93.018233105683,9.53130901619761));
#11742=CARTESIAN_POINT('Ctrl Pts',(-205.903960802919,92.5024544578432,9.58427845579904));
#11743=CARTESIAN_POINT('Ctrl Pts',(-204.967241498532,92.3440998232346,9.63724789540047));
#11744=CARTESIAN_POINT('Ctrl Pts',(-204.178656596937,92.6157580814132,9.69021733500191));
#11745=CARTESIAN_POINT('Ctrl Pts',(-203.390071695343,92.8874163395918,9.74318677460335));
#11746=CARTESIAN_POINT('Ctrl Pts',(-202.74962119654,93.5890874905577,9.79615621420478));
#11747=CARTESIAN_POINT('Ctrl Pts',(-202.55088403009,94.3991293999248,9.84912565380622));
#11748=CARTESIAN_POINT('Ctrl Pts',(-202.502995703142,94.5943196227229,9.86188933504016));
#11749=CARTESIAN_POINT('Ctrl Pts',(-202.480754676092,94.7958022010768,9.8746530162741));
#11750=CARTESIAN_POINT('Ctrl Pts',(-202.482602635909,94.9976869505601,9.88741669750804));
#11751=CARTESIAN_POINT('Ctrl Pts',(-202.486537867015,94.9998805722871,9.61258330249198));
#11752=CARTESIAN_POINT('Ctrl Pts',(-202.486363271877,94.5865641787485,9.58655524441412));
#11753=CARTESIAN_POINT('Ctrl Pts',(-202.582606290008,94.1733243516167,9.56052718633626));
#11754=CARTESIAN_POINT('Ctrl Pts',(-202.775711662331,93.8118265903401,9.5344991282584));
#11755=CARTESIAN_POINT('Ctrl Pts',(-203.168698466242,93.0761461267913,9.48152968865697));
#11756=CARTESIAN_POINT('Ctrl Pts',(-203.96284953751,92.5547601444516,9.42856024905553));
#11757=CARTESIAN_POINT('Ctrl Pts',(-204.794130463097,92.486669063914,9.3755908094541));
#11758=CARTESIAN_POINT('Ctrl Pts',(-205.625411388685,92.4185779833763,9.32262136985266));
#11759=CARTESIAN_POINT('Ctrl Pts',(-206.493822168593,92.8037818046407,9.26965193025122));
#11760=CARTESIAN_POINT('Ctrl Pts',(-207.001288154334,93.4657052487113,9.21668249064978));
#11761=CARTESIAN_POINT('Ctrl Pts',(-207.508754140076,94.1276286927818,9.16371305104835));
#11762=CARTESIAN_POINT('Ctrl Pts',(-207.655275331652,95.0662717596585,9.11074361144692));
#11763=CARTESIAN_POINT('Ctrl Pts',(-207.373687233662,95.8513657129949,9.05777417184548));
#11764=CARTESIAN_POINT('Ctrl Pts',(-207.092099135672,96.6364596663312,9.00480473224405));
#11765=CARTESIAN_POINT('Ctrl Pts',(-206.382401748116,97.2680045061271,8.95183529264261));
#11766=CARTESIAN_POINT('Ctrl Pts',(-205.569916387379,97.4565036071433,8.89886585304117));
#11767=CARTESIAN_POINT('Ctrl Pts',(-204.757431026643,97.6450027081595,8.84589641343974));
#11768=CARTESIAN_POINT('Ctrl Pts',(-203.842157692726,97.3904560703959,8.79292697383831));
#11769=CARTESIAN_POINT('Ctrl Pts',(-203.243652566985,96.8095464500958,8.73995753423687));
#11770=CARTESIAN_POINT('Ctrl Pts',(-202.763916004669,96.3439137056573,8.69749945698858));
#11771=CARTESIAN_POINT('Ctrl Pts',(-202.487701496429,95.6685943106478,8.65504137974028));
#11772=CARTESIAN_POINT('Ctrl Pts',(-202.481519189143,94.9977697596226,8.61258330249198));
#11773=CARTESIAN_POINT('Origin',(-205.,95.,9.));
#11774=CARTESIAN_POINT('',(-202.47917661211,95.0013671579498,7.61258330249198));
#11775=CARTESIAN_POINT('',(-202.484976668263,95.0018590801224,7.88741669750804));
#11776=CARTESIAN_POINT('',(-202.4825,95.,9.));
#11777=CARTESIAN_POINT('Ctrl Pts',(-202.484976668263,95.0018590801224,7.88741669750804));
#11778=CARTESIAN_POINT('Ctrl Pts',(-202.48299671483,95.291524891365,7.90568640772354));
#11779=CARTESIAN_POINT('Ctrl Pts',(-202.529190133705,95.5805786424467,7.92395611793904));
#11780=CARTESIAN_POINT('Ctrl Pts',(-202.626312794037,95.8513657030603,7.94222582815454));
#11781=CARTESIAN_POINT('Ctrl Pts',(-202.907900888741,96.6364596472354,7.99519526775598));
#11782=CARTESIAN_POINT('Ctrl Pts',(-203.617598268015,97.2680044796619,8.04816470735741));
#11783=CARTESIAN_POINT('Ctrl Pts',(-204.430083619271,97.4565035784785,8.10113414695885));
#11784=CARTESIAN_POINT('Ctrl Pts',(-205.242568970527,97.6450026772951,8.15410358656028));
#11785=CARTESIAN_POINT('Ctrl Pts',(-206.157842293763,97.3904560425019,8.20707302616171));
#11786=CARTESIAN_POINT('Ctrl Pts',(-206.75634741252,96.8095464289804,8.26004246576315));
#11787=CARTESIAN_POINT('Ctrl Pts',(-207.354852531277,96.2286368154588,8.31301190536458));
#11788=CARTESIAN_POINT('Ctrl Pts',(-207.636589445553,95.321364223209,8.36598134496602));
#11789=CARTESIAN_POINT('Ctrl Pts',(-207.472411528303,94.5036173383193,8.41895078456746));
#11790=CARTESIAN_POINT('Ctrl Pts',(-207.308233611052,93.6858704534295,8.47192022416889));
#11791=CARTESIAN_POINT('Ctrl Pts',(-206.698140862275,92.9576492758997,8.52488966377033));
#11792=CARTESIAN_POINT('Ctrl Pts',(-205.92179638857,92.6527663239208,8.57785910337176));
#11793=CARTESIAN_POINT('Ctrl Pts',(-205.145451914865,92.3478833719418,8.6308285429732));
#11794=CARTESIAN_POINT('Ctrl Pts',(-204.202855716232,92.4663386455136,8.68379798257463));
#11795=CARTESIAN_POINT('Ctrl Pts',(-203.526088622524,92.9538329092061,8.73676742217607));
#11796=CARTESIAN_POINT('Ctrl Pts',(-202.884495576906,93.415990322401,8.78698384728672));
#11797=CARTESIAN_POINT('Ctrl Pts',(-202.481817498035,94.2098229977097,8.83720027239738));
#11798=CARTESIAN_POINT('Ctrl Pts',(-202.478555055026,95.000793452331,8.88741669750803));
#11799=CARTESIAN_POINT('Ctrl Pts',(-202.481519189143,94.9977697596226,8.61258330249198));
#11800=CARTESIAN_POINT('Ctrl Pts',(-202.479988632974,94.8316934700635,8.60207194013884));
#11801=CARTESIAN_POINT('Ctrl Pts',(-202.495008645671,94.6658926744072,8.5915605777857));
#11802=CARTESIAN_POINT('Ctrl Pts',(-202.527588442847,94.5036173325269,8.58104921543256));
#11803=CARTESIAN_POINT('Ctrl Pts',(-202.691766362013,93.6858704380949,8.52807977583112));
#11804=CARTESIAN_POINT('Ctrl Pts',(-203.30185911791,92.9576492520676,8.47511033622969));
#11805=CARTESIAN_POINT('Ctrl Pts',(-204.078203600674,92.652766296531,8.42214089662825));
#11806=CARTESIAN_POINT('Ctrl Pts',(-204.854548083438,92.3478833409944,8.36917145702682));
#11807=CARTESIAN_POINT('Ctrl Pts',(-205.79714429307,92.4663386159487,8.31620201742538));
#11808=CARTESIAN_POINT('Ctrl Pts',(-206.473911394675,92.9538328853297,8.26323257782395));
#11809=CARTESIAN_POINT('Ctrl Pts',(-207.150678496281,93.4413271547107,8.21026313822251));
#11810=CARTESIAN_POINT('Ctrl Pts',(-207.56161648986,94.2978604185185,8.15729369862107));
#11811=CARTESIAN_POINT('Ctrl Pts',(-207.518353695641,95.1308026152713,8.10432425901964));
#11812=CARTESIAN_POINT('Ctrl Pts',(-207.475090901422,95.963744812024,8.0513548194182));
#11813=CARTESIAN_POINT('Ctrl Pts',(-206.977627319405,96.7730959417216,7.99838537981677));
#11814=CARTESIAN_POINT('Ctrl Pts',(-206.253997475562,97.1878539694859,7.94541594021533));
#11815=CARTESIAN_POINT('Ctrl Pts',(-205.530367631719,97.6026119972502,7.8924465006139));
#11816=CARTESIAN_POINT('Ctrl Pts',(-204.580571526051,97.6227769230812,7.83947706101246));
#11817=CARTESIAN_POINT('Ctrl Pts',(-203.839990385558,97.2391052576674,7.78650762141103));
#11818=CARTESIAN_POINT('Ctrl Pts',(-203.099409245065,96.8554335922537,7.73353818180959));
#11819=CARTESIAN_POINT('Ctrl Pts',(-202.568043069748,96.0679253355952,7.68056874220816));
#11820=CARTESIAN_POINT('Ctrl Pts',(-202.489467144887,95.2375698716359,7.62759930260672));
#11821=CARTESIAN_POINT('Ctrl Pts',(-202.482042133373,95.1591056487688,7.62259396923514));
#11822=CARTESIAN_POINT('Ctrl Pts',(-202.478660201786,95.0802588322316,7.61758863586356));
#11823=CARTESIAN_POINT('Ctrl Pts',(-202.47917661211,95.0013671579498,7.61258330249198));
#11824=CARTESIAN_POINT('Origin',(-205.,95.,9.));
#11825=CARTESIAN_POINT('',(-202.485696042915,95.0014474120785,6.61258330249198));
#11826=CARTESIAN_POINT('',(-202.485291143957,94.9982947746438,6.88741669750803));
#11827=CARTESIAN_POINT('',(-202.4825,95.,9.));
#11828=CARTESIAN_POINT('Ctrl Pts',(-202.485291143957,94.9982947746438,6.88741669750803));
#11829=CARTESIAN_POINT('Ctrl Pts',(-202.488623019757,95.53414575907,6.92120310344825));
#11830=CARTESIAN_POINT('Ctrl Pts',(-202.656226186158,96.0718997890027,6.95498950938847));
#11831=CARTESIAN_POINT('Ctrl Pts',(-202.97259571778,96.499615413543,6.9887759153287));
#11832=CARTESIAN_POINT('Ctrl Pts',(-203.468591557841,97.1701767328134,7.04174535493013));
#11833=CARTESIAN_POINT('Ctrl Pts',(-204.330242398534,97.5702730640224,7.09471479453157));
#11834=CARTESIAN_POINT('Ctrl Pts',(-205.162572309731,97.5165024848408,7.147684234133));
#11835=CARTESIAN_POINT('Ctrl Pts',(-205.994902220929,97.4627319056592,7.20065367373444));
#11836=CARTESIAN_POINT('Ctrl Pts',(-206.797911202631,96.9550944160871,7.25362311333587));
#11837=CARTESIAN_POINT('Ctrl Pts',(-207.203504425158,96.2262882044646,7.30659255293731));
#11838=CARTESIAN_POINT('Ctrl Pts',(-207.609097647686,95.4974819928421,7.35956199253874));
#11839=CARTESIAN_POINT('Ctrl Pts',(-207.617275111038,94.5475070591692,7.41253143214018));
#11840=CARTESIAN_POINT('Ctrl Pts',(-207.224288311714,93.8118266042049,7.46550087174162));
#11841=CARTESIAN_POINT('Ctrl Pts',(-206.831301512389,93.0761461492407,7.51847031134305));
#11842=CARTESIAN_POINT('Ctrl Pts',(-206.037150450388,92.554760172985,7.57143975094449));
#11843=CARTESIAN_POINT('Ctrl Pts',(-205.205869534501,92.4866690932419,7.62440919054592));
#11844=CARTESIAN_POINT('Ctrl Pts',(-204.374588618613,92.4185780134987,7.67737863014736));
#11845=CARTESIAN_POINT('Ctrl Pts',(-203.506177848839,92.8037818302682,7.73034806974879));
#11846=CARTESIAN_POINT('Ctrl Pts',(-202.998711869018,93.4657052666148,7.78331750935023));
#11847=CARTESIAN_POINT('Ctrl Pts',(-202.666276179594,93.8993244305753,7.81801723873616));
#11848=CARTESIAN_POINT('Ctrl Pts',(-202.488737201272,94.4516957144252,7.8527169681221));
#11849=CARTESIAN_POINT('Ctrl Pts',(-202.484976668263,95.0018590801224,7.88741669750804));
#11850=CARTESIAN_POINT('Ctrl Pts',(-202.47917661211,95.0013671579498,7.61258330249198));
#11851=CARTESIAN_POINT('Ctrl Pts',(-202.484125165545,94.2453798210446,7.56461919626212));
#11852=CARTESIAN_POINT('Ctrl Pts',(-202.847043711761,93.4852733671239,7.51665509003227));
#11853=CARTESIAN_POINT('Ctrl Pts',(-203.440572366077,93.0182330825579,7.46869098380242));
#11854=CARTESIAN_POINT('Ctrl Pts',(-204.096039186533,92.5024544286996,7.41572154420098));
#11855=CARTESIAN_POINT('Ctrl Pts',(-205.03275850185,92.3440997922431,7.36275210459954));
#11856=CARTESIAN_POINT('Ctrl Pts',(-205.821343412647,92.6157580535917,7.3097826649981));
#11857=CARTESIAN_POINT('Ctrl Pts',(-206.609928323444,92.8874163149403,7.25681322539667));
#11858=CARTESIAN_POINT('Ctrl Pts',(-207.250378829719,93.589087474094,7.20384378579524));
#11859=CARTESIAN_POINT('Ctrl Pts',(-207.449115998488,94.3991293929133,7.15087434619381));
#11860=CARTESIAN_POINT('Ctrl Pts',(-207.647853167257,95.2091713117327,7.09790490659237));
#11861=CARTESIAN_POINT('Ctrl Pts',(-207.40487699852,96.1275839902179,7.04493546699093));
#11862=CARTESIAN_POINT('Ctrl Pts',(-206.831566410178,96.7333721890055,6.99196602738949));
#11863=CARTESIAN_POINT('Ctrl Pts',(-206.258255821837,97.3391603877931,6.93899658778806));
#11864=CARTESIAN_POINT('Ctrl Pts',(-205.354610813891,97.6323241068831,6.88602714818662));
#11865=CARTESIAN_POINT('Ctrl Pts',(-204.534857208056,97.4784787357599,6.83305770858519));
#11866=CARTESIAN_POINT('Ctrl Pts',(-203.715103602222,97.3246333646367,6.78008826898375));
#11867=CARTESIAN_POINT('Ctrl Pts',(-202.979241398498,96.7237789033003,6.72711882938231));
#11868=CARTESIAN_POINT('Ctrl Pts',(-202.664585718783,95.9513436790141,6.67414938978088));
#11869=CARTESIAN_POINT('Ctrl Pts',(-202.542678198843,95.6520779464127,6.65362736068458));
#11870=CARTESIAN_POINT('Ctrl Pts',(-202.483995110087,95.3270573987234,6.63310533158828));
#11871=CARTESIAN_POINT('Ctrl Pts',(-202.485696042915,95.0014474120785,6.61258330249198));
#11872=CARTESIAN_POINT('Origin',(-205.,95.,9.));
#11873=CARTESIAN_POINT('',(-202.484465795159,94.9979518675787,5.61258330249198));
#11874=CARTESIAN_POINT('',(-202.478772719,94.9989624714564,5.88741669750803));
#11875=CARTESIAN_POINT('',(-202.4825,95.,9.));
#11876=CARTESIAN_POINT('Ctrl Pts',(-202.478772719,94.9989624714564,5.88741669750803));
#11877=CARTESIAN_POINT('Ctrl Pts',(-202.482817100591,95.7757252592268,5.93671979917298));
#11878=CARTESIAN_POINT('Ctrl Pts',(-202.869063212578,96.5559620071741,5.98602290083791));
#11879=CARTESIAN_POINT('Ctrl Pts',(-203.491082493968,97.020490651325,6.03532600250285));
#11880=CARTESIAN_POINT('Ctrl Pts',(-204.159357138847,97.5195631463317,6.08829544210429));
#11881=CARTESIAN_POINT('Ctrl Pts',(-205.099774462154,97.6542275571366,6.14126488170573));
#11882=CARTESIAN_POINT('Ctrl Pts',(-205.881252418311,97.3627544703847,6.19423432130716));
#11883=CARTESIAN_POINT('Ctrl Pts',(-206.662730374467,97.0712813836329,6.2472037609086));
#11884=CARTESIAN_POINT('Ctrl Pts',(-207.285268963474,96.3536707993244,6.30017320051003));
#11885=CARTESIAN_POINT('Ctrl Pts',(-207.463499975122,95.5388713990138,6.35314264011147));
#11886=CARTESIAN_POINT('Ctrl Pts',(-207.64173098677,94.7240719987032,6.4061120797129));
#11887=CARTESIAN_POINT('Ctrl Pts',(-207.37565442106,93.8120837823904,6.45908151931434));
#11888=CARTESIAN_POINT('Ctrl Pts',(-206.787238288771,93.2209570518813,6.51205095891577));
#11889=CARTESIAN_POINT('Ctrl Pts',(-206.198822156483,92.6298303213723,6.56502039851721));
#11890=CARTESIAN_POINT('Ctrl Pts',(-205.288066457616,92.3595650766669,6.61798983811865));
#11891=CARTESIAN_POINT('Ctrl Pts',(-204.472456514868,92.5340493955888,6.67095927772008));
#11892=CARTESIAN_POINT('Ctrl Pts',(-203.65684657212,92.7085337145107,6.72392871732152));
#11893=CARTESIAN_POINT('Ctrl Pts',(-202.936382385489,93.3277675970599,6.77689815692295));
#11894=CARTESIAN_POINT('Ctrl Pts',(-202.641320711889,94.1078976920004,6.82986759652439));
#11895=CARTESIAN_POINT('Ctrl Pts',(-202.534463285052,94.3904240314138,6.8490506301856));
#11896=CARTESIAN_POINT('Ctrl Pts',(-202.483399392413,94.6940526634873,6.86823366384682));
#11897=CARTESIAN_POINT('Ctrl Pts',(-202.485291143957,94.9982947746438,6.88741669750803));
#11898=CARTESIAN_POINT('Ctrl Pts',(-202.485696042915,95.0014474120785,6.61258330249198));
#11899=CARTESIAN_POINT('Ctrl Pts',(-202.48838539032,94.4866249814282,6.58013589198684));
#11900=CARTESIAN_POINT('Ctrl Pts',(-202.642027659063,93.9703290230142,6.54768848148171));
#11901=CARTESIAN_POINT('Ctrl Pts',(-202.935395940087,93.5520273703197,6.51524107097657));
#11902=CARTESIAN_POINT('Ctrl Pts',(-203.414310996813,92.8691622731474,6.46227163137514));
#11903=CARTESIAN_POINT('Ctrl Pts',(-204.265590265972,92.4474480660385,6.4093021917737));
#11904=CARTESIAN_POINT('Ctrl Pts',(-205.099012087867,92.4801961848256,6.35633275217227));
#11905=CARTESIAN_POINT('Ctrl Pts',(-205.932433909762,92.5129443036126,6.30336331257083));
#11906=CARTESIAN_POINT('Ctrl Pts',(-206.747998284393,93.0001547482956,6.2503938729694));
#11907=CARTESIAN_POINT('Ctrl Pts',(-207.171855060127,93.718492973757,6.19742443336796));
#11908=CARTESIAN_POINT('Ctrl Pts',(-207.595711835862,94.4368311992184,6.14445499376652));
#11909=CARTESIAN_POINT('Ctrl Pts',(-207.627861012699,95.3862972054583,6.09148555416509));
#11910=CARTESIAN_POINT('Ctrl Pts',(-207.253565587638,96.1316610812089,6.03851611456365));
#11911=CARTESIAN_POINT('Ctrl Pts',(-206.879270162578,96.8770249569596,5.98554667496222));
#11912=CARTESIAN_POINT('Ctrl Pts',(-206.098530135621,97.4182867022209,5.93257723536078));
#11913=CARTESIAN_POINT('Ctrl Pts',(-205.269232372039,97.5073349577505,5.87960779575935));
#11914=CARTESIAN_POINT('Ctrl Pts',(-204.439934608457,97.59638321328,5.82663835615791));
#11915=CARTESIAN_POINT('Ctrl Pts',(-203.56207910825,97.2332179790778,5.77366891655647));
#11916=CARTESIAN_POINT('Ctrl Pts',(-203.038069926909,96.5843121689908,5.72069947695504));
#11917=CARTESIAN_POINT('Ctrl Pts',(-202.681550718245,96.1428172598422,5.68466075213402));
#11918=CARTESIAN_POINT('Ctrl Pts',(-202.488827307777,95.5690527658245,5.648622027313));
#11919=CARTESIAN_POINT('Ctrl Pts',(-202.484465795159,94.9979518675787,5.61258330249198));
#11920=CARTESIAN_POINT('Origin',(-205.,95.,9.));
#11921=CARTESIAN_POINT('',(-202.478335424994,94.9995851060564,4.61258330249197));
#11922=CARTESIAN_POINT('',(-202.482163844592,95.0022992344272,4.88741669750803));
#11923=CARTESIAN_POINT('',(-202.4825,95.,9.));
#11924=CARTESIAN_POINT('Ctrl Pts',(-202.482163844592,95.0022992344272,4.88741669750803));
#11925=CARTESIAN_POINT('Ctrl Pts',(-202.480430729047,95.189654321574,4.89926705529626));
#11926=CARTESIAN_POINT('Ctrl Pts',(-202.49956775128,95.3766586399814,4.91111741308448));
#11927=CARTESIAN_POINT('Ctrl Pts',(-202.540903035897,95.5586202943346,4.92296777087271));
#11928=CARTESIAN_POINT('Ctrl Pts',(-202.725665968888,96.3719634044993,4.97593721047414));
#11929=CARTESIAN_POINT('Ctrl Pts',(-203.353942368752,97.0845558622811,5.02890665007558));
#11930=CARTESIAN_POINT('Ctrl Pts',(-204.13773384485,97.369749267282,5.08187608967702));
#11931=CARTESIAN_POINT('Ctrl Pts',(-204.921525320947,97.6549426722829,5.13484552927845));
#11932=CARTESIAN_POINT('Ctrl Pts',(-205.860831873279,97.5127370245029,5.18781496887989));
#11933=CARTESIAN_POINT('Ctrl Pts',(-206.525080627473,97.0083185981828,5.24078440848132));
#11934=CARTESIAN_POINT('Ctrl Pts',(-207.189329381667,96.5039001718628,5.29375384808276));
#11935=CARTESIAN_POINT('Ctrl Pts',(-207.578520337724,95.6372689670026,5.34672328768419));
#11936=CARTESIAN_POINT('Ctrl Pts',(-207.51425053634,94.8056838848314,5.39969272728563));
#11937=CARTESIAN_POINT('Ctrl Pts',(-207.449980734956,93.9740988026602,5.45266216688706));
#11938=CARTESIAN_POINT('Ctrl Pts',(-206.932250176132,93.1775598431778,5.5056316064885));
#11939=CARTESIAN_POINT('Ctrl Pts',(-206.198383654749,92.7811960140355,5.55860104608994));
#11940=CARTESIAN_POINT('Ctrl Pts',(-205.464517133366,92.3848321848932,5.61157048569137));
#11941=CARTESIAN_POINT('Ctrl Pts',(-204.514514649423,92.3886434860908,5.66453992529281));
#11942=CARTESIAN_POINT('Ctrl Pts',(-203.78385203257,92.7908828384584,5.71750936489424));
#11943=CARTESIAN_POINT('Ctrl Pts',(-203.053189415717,93.1931221908261,5.77047880449568));
#11944=CARTESIAN_POINT('Ctrl Pts',(-202.541866665953,93.9937895943638,5.82344824409711));
#11945=CARTESIAN_POINT('Ctrl Pts',(-202.484271274297,94.8258635857369,5.87641768369855));
#11946=CARTESIAN_POINT('Ctrl Pts',(-202.480284746008,94.8834565008875,5.88008402163505));
#11947=CARTESIAN_POINT('Ctrl Pts',(-202.478471965718,94.9411998808629,5.88375035957154));
#11948=CARTESIAN_POINT('Ctrl Pts',(-202.478772719,94.9989624714564,5.88741669750803));
#11949=CARTESIAN_POINT('Ctrl Pts',(-202.484465795159,94.9979518675787,5.61258330249198));
#11950=CARTESIAN_POINT('Ctrl Pts',(-202.482416790193,94.7296530732386,5.59565258771156));
#11951=CARTESIAN_POINT('Ctrl Pts',(-202.521940158033,94.4619421472396,5.57872187293115));
#11952=CARTESIAN_POINT('Ctrl Pts',(-202.605583044702,94.2088096912299,5.56179115815073));
#11953=CARTESIAN_POINT('Ctrl Pts',(-202.867268206312,93.416859409528,5.5088217185493));
#11954=CARTESIAN_POINT('Ctrl Pts',(-203.56080139201,92.7676052320959,5.45585227894786));
#11955=CARTESIAN_POINT('Ctrl Pts',(-204.368270865209,92.5586616455789,5.40288283934642));
#11956=CARTESIAN_POINT('Ctrl Pts',(-205.175740338408,92.3497180590619,5.34991339974499));
#11957=CARTESIAN_POINT('Ctrl Pts',(-206.097146099108,92.5810850634599,5.29694396014356));
#11958=CARTESIAN_POINT('Ctrl Pts',(-206.710120895786,93.1467053169272,5.24397452054212));
#11959=CARTESIAN_POINT('Ctrl Pts',(-207.323095692464,93.7123255703945,5.19100508094069));
#11960=CARTESIAN_POINT('Ctrl Pts',(-207.62763952512,94.6121990729312,5.13803564133925));
#11961=CARTESIAN_POINT('Ctrl Pts',(-207.484151202775,95.4338288398249,5.08506620173782));
#11962=CARTESIAN_POINT('Ctrl Pts',(-207.34066288043,96.2554586067186,5.03209676213638));
#11963=CARTESIAN_POINT('Ctrl Pts',(-206.749142403085,96.9988446379694,4.97912732253494));
#11964=CARTESIAN_POINT('Ctrl Pts',(-205.980739451904,97.3232229311869,4.92615788293351));
#11965=CARTESIAN_POINT('Ctrl Pts',(-205.212336500722,97.6476012244043,4.87318844333207));
#11966=CARTESIAN_POINT('Ctrl Pts',(-204.267051075705,97.5529717795884,4.82021900373064));
#11967=CARTESIAN_POINT('Ctrl Pts',(-203.578196733049,97.082712205418,4.7672495641292));
#11968=CARTESIAN_POINT('Ctrl Pts',(-202.907731355322,96.6250062093864,4.71569414358346));
#11969=CARTESIAN_POINT('Ctrl Pts',(-202.48018894443,95.8114572920712,4.66413872303772));
#11970=CARTESIAN_POINT('Ctrl Pts',(-202.478335424994,94.9995851060564,4.61258330249197));
#11971=CARTESIAN_POINT('Origin',(-205.,95.,9.));
#11972=CARTESIAN_POINT('',(-202.483233810455,95.0022852208457,3.61258330249198));
#11973=CARTESIAN_POINT('',(-202.486523939152,94.9997695205866,3.88741669750803));
#11974=CARTESIAN_POINT('',(-202.4825,95.,9.));
#11975=CARTESIAN_POINT('Ctrl Pts',(-202.486523939152,94.9997695205866,3.88741669750803));
#11976=CARTESIAN_POINT('Ctrl Pts',(-202.486878327319,95.4343426674579,3.91478375102098));
#11977=CARTESIAN_POINT('Ctrl Pts',(-202.593838556984,95.8690792275426,3.94215080453392));
#11978=CARTESIAN_POINT('Ctrl Pts',(-202.80640580289,96.2439288606997,3.96951785804687));
#11979=CARTESIAN_POINT('Ctrl Pts',(-203.21783364944,96.9694572773319,4.0224872976483));
#11980=CARTESIAN_POINT('Ctrl Pts',(-204.024889883747,97.4706353696046,4.07545673724974));
#11981=CARTESIAN_POINT('Ctrl Pts',(-204.85762443817,97.517725900789,4.12842617685117));
#11982=CARTESIAN_POINT('Ctrl Pts',(-205.690358992592,97.5648164319734,4.18139561645261));
#11983=CARTESIAN_POINT('Ctrl Pts',(-206.54877186713,97.1578194020694,4.23436505605404));
#11984=CARTESIAN_POINT('Ctrl Pts',(-207.03937139724,96.4832999751306,4.28733449565548));
#11985=CARTESIAN_POINT('Ctrl Pts',(-207.529970927349,95.8087805481917,4.34030393525692));
#11986=CARTESIAN_POINT('Ctrl Pts',(-207.652757113031,94.866738724218,4.39327337485835));
#11987=CARTESIAN_POINT('Ctrl Pts',(-207.35144545295,94.0890012108126,4.44624281445979));
#11988=CARTESIAN_POINT('Ctrl Pts',(-207.050133792868,93.3112636974072,4.49921225406122));
#11989=CARTESIAN_POINT('Ctrl Pts',(-206.324724287023,92.69783049457,4.55218169366266));
#11990=CARTESIAN_POINT('Ctrl Pts',(-205.507740599016,92.529895954375,4.6051511332641));
#11991=CARTESIAN_POINT('Ctrl Pts',(-204.69075691101,92.3619614141801,4.65812057286553));
#11992=CARTESIAN_POINT('Ctrl Pts',(-203.782199040842,92.6395255366275,4.71109001246697));
#11993=CARTESIAN_POINT('Ctrl Pts',(-203.198544838816,93.2353544791249,4.7640594520684));
#11994=CARTESIAN_POINT('Ctrl Pts',(-202.745466137884,93.6978841796009,4.80517853388161));
#11995=CARTESIAN_POINT('Ctrl Pts',(-202.488177512802,94.3522033222036,4.84629761569482));
#11996=CARTESIAN_POINT('Ctrl Pts',(-202.482163844592,95.0022992344272,4.88741669750803));
#11997=CARTESIAN_POINT('Ctrl Pts',(-202.478335424994,94.9995851060564,4.61258330249197));
#11998=CARTESIAN_POINT('Ctrl Pts',(-202.478284588209,94.9773177531833,4.61116928343628));
#11999=CARTESIAN_POINT('Ctrl Pts',(-202.478553975643,94.9550516616304,4.60975526438059));
#12000=CARTESIAN_POINT('Ctrl Pts',(-202.479147358134,94.9327942077677,4.60834124532489));
#12001=CARTESIAN_POINT('Ctrl Pts',(-202.501375586168,94.0990254878127,4.55537180572346));
#12002=CARTESIAN_POINT('Ctrl Pts',(-202.978255302531,93.2773777514274,4.50240236612202));
#12003=CARTESIAN_POINT('Ctrl Pts',(-203.691187510233,92.8444897292865,4.44943292652059));
#12004=CARTESIAN_POINT('Ctrl Pts',(-204.404119717935,92.4116017071456,4.39646348691915));
#12005=CARTESIAN_POINT('Ctrl Pts',(-205.353104416976,92.367473399249,4.34349404731772));
#12006=CARTESIAN_POINT('Ctrl Pts',(-206.103132324622,92.7323329753115,4.29052460771628));
#12007=CARTESIAN_POINT('Ctrl Pts',(-206.853160232269,93.097192551374,4.23755516811485));
#12008=CARTESIAN_POINT('Ctrl Pts',(-207.40423134852,93.8710400113955,4.18458572851341));
#12009=CARTESIAN_POINT('Ctrl Pts',(-207.503737753283,94.6991480043073,4.13161628891197));
#12010=CARTESIAN_POINT('Ctrl Pts',(-207.603244158046,95.527255997219,4.07864684931054));
#12011=CARTESIAN_POINT('Ctrl Pts',(-207.251185851321,96.409624523021,4.0256774097091));
#12012=CARTESIAN_POINT('Ctrl Pts',(-206.608944393485,96.9417807804312,3.97270797010767));
#12013=CARTESIAN_POINT('Ctrl Pts',(-205.96670293565,97.4739370378414,3.91973853050623));
#12014=CARTESIAN_POINT('Ctrl Pts',(-205.034278326703,97.6558810268598,3.86676909090479));
#12015=CARTESIAN_POINT('Ctrl Pts',(-204.239088796595,97.4042106398603,3.81379965130336));
#12016=CARTESIAN_POINT('Ctrl Pts',(-203.443899266487,97.1525402528608,3.76083021170192));
#12017=CARTESIAN_POINT('Ctrl Pts',(-202.785944815216,96.4672554898434,3.70786077210049));
#12018=CARTESIAN_POINT('Ctrl Pts',(-202.566828086406,95.6624870561916,3.65489133249905));
#12019=CARTESIAN_POINT('Ctrl Pts',(-202.50849006353,95.4482240944041,3.64078865583003));
#12020=CARTESIAN_POINT('Ctrl Pts',(-202.481258909196,95.2254915716718,3.626685979161));
#12021=CARTESIAN_POINT('Ctrl Pts',(-202.483233810455,95.0022852208457,3.61258330249198));
#12022=CARTESIAN_POINT('Origin',(-205.,95.,9.));
#12023=CARTESIAN_POINT('',(-202.486304042859,94.9991964067408,2.61258330249198));
#12024=CARTESIAN_POINT('',(-202.481316067847,94.9978038198253,2.88741669750803));
#12025=CARTESIAN_POINT('',(-202.4825,95.,9.));
#12026=CARTESIAN_POINT('Ctrl Pts',(-202.481316067847,94.9978038198253,2.88741669750803));
#12027=CARTESIAN_POINT('Ctrl Pts',(-202.487520285317,95.6752130989754,2.9303004467457));
#12028=CARTESIAN_POINT('Ctrl Pts',(-202.769924095146,96.3571824133273,2.97318419598336));
#12029=CARTESIAN_POINT('Ctrl Pts',(-203.258228276972,96.823580482169,3.01606794522103));
#12030=CARTESIAN_POINT('Ctrl Pts',(-203.861375140903,97.3996692052147,3.06903738482246));
#12031=CARTESIAN_POINT('Ctrl Pts',(-204.778661392001,97.646863821374,3.1220068244239));
#12032=CARTESIAN_POINT('Ctrl Pts',(-205.589608139994,97.4518516989913,3.17497626402533));
#12033=CARTESIAN_POINT('Ctrl Pts',(-206.400554887986,97.2568395766086,3.22794570362677));
#12034=CARTESIAN_POINT('Ctrl Pts',(-207.105162132873,96.6196207156839,3.2809151432282));
#12035=CARTESIAN_POINT('Ctrl Pts',(-207.380441850704,95.8322926815315,3.33388458282964));
#12036=CARTESIAN_POINT('Ctrl Pts',(-207.655721568535,95.044964647379,3.38685402243108));
#12037=CARTESIAN_POINT('Ctrl Pts',(-207.501673759311,94.1075274399988,3.43982346203251));
#12038=CARTESIAN_POINT('Ctrl Pts',(-206.98891307815,93.4496970362421,3.49279290163395));
#12039=CARTESIAN_POINT('Ctrl Pts',(-206.47615239699,92.7918666324854,3.54576234123538));
#12040=CARTESIAN_POINT('Ctrl Pts',(-205.604678843892,92.4136430323522,3.59873178083682));
#12041=CARTESIAN_POINT('Ctrl Pts',(-204.773971025337,92.4884018205965,3.65170122043826));
#12042=CARTESIAN_POINT('Ctrl Pts',(-203.943263206782,92.5631606088408,3.70467066003969));
#12043=CARTESIAN_POINT('Ctrl Pts',(-203.153321122769,93.0909017854627,3.75764009964113));
#12044=CARTESIAN_POINT('Ctrl Pts',(-202.766249810158,93.8297117442694,3.81060953924256));
#12045=CARTESIAN_POINT('Ctrl Pts',(-202.579161759694,94.1868100627285,3.83621192533105));
#12046=CARTESIAN_POINT('Ctrl Pts',(-202.486192402449,94.5932182824481,3.86181431141954));
#12047=CARTESIAN_POINT('Ctrl Pts',(-202.486523939152,94.9997695205866,3.88741669750803));
#12048=CARTESIAN_POINT('Ctrl Pts',(-202.483233810455,95.0022852208457,3.61258330249198));
#12049=CARTESIAN_POINT('Ctrl Pts',(-202.488676608362,94.3871319044816,3.57371653955957));
#12050=CARTESIAN_POINT('Ctrl Pts',(-202.715952610492,93.7683796493997,3.53484977662716));
#12051=CARTESIAN_POINT('Ctrl Pts',(-203.125272191609,93.3134027435547,3.49598301369475));
#12052=CARTESIAN_POINT('Ctrl Pts',(-203.683112031973,92.6933389688557,3.44301357409331));
#12053=CARTESIAN_POINT('Ctrl Pts',(-204.57907071905,92.3774635237437,3.39004413449188));
#12054=CARTESIAN_POINT('Ctrl Pts',(-205.402445797958,92.5105719455655,3.33707469489044));
#12055=CARTESIAN_POINT('Ctrl Pts',(-206.225820876866,92.6436803673873,3.28410525528901));
#12056=CARTESIAN_POINT('Ctrl Pts',(-206.976612347604,93.2257726561428,3.23113581568757));
#12057=CARTESIAN_POINT('Ctrl Pts',(-207.310661595086,93.990020962638,3.17816637608613));
#12058=CARTESIAN_POINT('Ctrl Pts',(-207.644710842568,94.7542692691331,3.1251969364847));
#12059=CARTESIAN_POINT('Ctrl Pts',(-207.562017866793,95.7006735933678,3.07222749688326));
#12060=CARTESIAN_POINT('Ctrl Pts',(-207.10048866702,96.3954074757752,3.01925805728183));
#12061=CARTESIAN_POINT('Ctrl Pts',(-206.638959467246,97.0901413581826,2.96628861768039));
#12062=CARTESIAN_POINT('Ctrl Pts',(-205.798594043474,97.5332047987627,2.91331917807896));
#12063=CARTESIAN_POINT('Ctrl Pts',(-204.964611207011,97.5215000052282,2.86034973847752));
#12064=CARTESIAN_POINT('Ctrl Pts',(-204.130628370548,97.5097952116936,2.80738029887609));
#12065=CARTESIAN_POINT('Ctrl Pts',(-203.303028121394,97.0433221840444,2.75441085927465));
#12066=CARTESIAN_POINT('Ctrl Pts',(-202.86117779429,96.3359095247307,2.70144141967321));
#12067=CARTESIAN_POINT('Ctrl Pts',(-202.614104586054,95.940339566847,2.67182204727947));
#12068=CARTESIAN_POINT('Ctrl Pts',(-202.487647897893,95.4694324584975,2.64220267488572));
#12069=CARTESIAN_POINT('Ctrl Pts',(-202.486304042859,94.9991964067408,2.61258330249198));
#12070=CARTESIAN_POINT('Origin',(-205.,95.,9.));
#12071=CARTESIAN_POINT('',(-202.480282650156,94.9980775783256,1.61258330249198));
#12072=CARTESIAN_POINT('',(-202.479323465531,95.0014637551426,1.88741669750803));
#12073=CARTESIAN_POINT('',(-202.4825,95.,9.));
#12074=CARTESIAN_POINT('Ctrl Pts',(-202.479323465531,95.0014637551426,1.88741669750803));
#12075=CARTESIAN_POINT('Ctrl Pts',(-202.478731735526,95.0870778064218,1.89284770286898));
#12076=CARTESIAN_POINT('Ctrl Pts',(-202.482714810237,95.1726361517413,1.89827870822993));
#12077=CARTESIAN_POINT('Ctrl Pts',(-202.491454117109,95.25770588247,1.90370971359088));
#12078=CARTESIAN_POINT('Ctrl Pts',(-202.576689935662,96.087404191395,1.95667915319232));
#12079=CARTESIAN_POINT('Ctrl Pts',(-203.114357779528,96.8706235057184,2.00964859279375));
#12080=CARTESIAN_POINT('Ctrl Pts',(-203.857993540713,97.2483406348987,2.06261803239519));
#12081=CARTESIAN_POINT('Ctrl Pts',(-204.601629301898,97.626057764079,2.11558747199662));
#12082=CARTESIAN_POINT('Ctrl Pts',(-205.551232980402,97.5982727081163,2.16855691159806));
#12083=CARTESIAN_POINT('Ctrl Pts',(-206.271511640473,97.1777219009975,2.22152635119949));
#12084=CARTESIAN_POINT('Ctrl Pts',(-206.991790300543,96.7571710938786,2.27449579080093));
#12085=CARTESIAN_POINT('Ctrl Pts',(-207.482743942181,95.9438545356035,2.32746523040237));
#12086=CARTESIAN_POINT('Ctrl Pts',(-207.519322119212,95.1105920302357,2.3804346700038));
#12087=CARTESIAN_POINT('Ctrl Pts',(-207.555900296242,94.2773295248679,2.43340410960524));
#12088=CARTESIAN_POINT('Ctrl Pts',(-207.138103008664,93.4241210724073,2.48637354920667));
#12089=CARTESIAN_POINT('Ctrl Pts',(-206.457446217874,92.9420726405858,2.53934298880811));
#12090=CARTESIAN_POINT('Ctrl Pts',(-205.776789427083,92.4600242087642,2.59231242840954));
#12091=CARTESIAN_POINT('Ctrl Pts',(-204.833273133079,92.3491357975817,2.64528186801098));
#12092=CARTESIAN_POINT('Ctrl Pts',(-204.059399922816,92.6602380441338,2.69825130761242));
#12093=CARTESIAN_POINT('Ctrl Pts',(-203.285526712553,92.9713402906858,2.75122074721385));
#12094=CARTESIAN_POINT('Ctrl Pts',(-202.681296586031,93.7044331949723,2.80419018681529));
#12095=CARTESIAN_POINT('Ctrl Pts',(-202.523685261153,94.5234710620817,2.85715962641672));
#12096=CARTESIAN_POINT('Ctrl Pts',(-202.493675145273,94.6794206508639,2.86724531678049));
#12097=CARTESIAN_POINT('Ctrl Pts',(-202.479856917995,94.8384861211514,2.87733100714426));
#12098=CARTESIAN_POINT('Ctrl Pts',(-202.481316067847,94.9978038198253,2.88741669750803));
#12099=CARTESIAN_POINT('Ctrl Pts',(-202.486304042859,94.9991964067408,2.61258330249198));
#12100=CARTESIAN_POINT('Ctrl Pts',(-202.485244631304,94.628491610365,2.58923323528429));
#12101=CARTESIAN_POINT('Ctrl Pts',(-202.561939879356,94.2582038597523,2.5658831680766));
#12102=CARTESIAN_POINT('Ctrl Pts',(-202.718592679948,93.9255720971807,2.54253310086891));
#12103=CARTESIAN_POINT('Ctrl Pts',(-203.073958297766,93.1709996199226,2.48956366126747));
#12104=CARTESIAN_POINT('Ctrl Pts',(-203.840789938455,92.6102069563844,2.43659422166604));
#12105=CARTESIAN_POINT('Ctrl Pts',(-204.667576286735,92.5002582159558,2.3836247820646));
#12106=CARTESIAN_POINT('Ctrl Pts',(-205.494362635015,92.3903094755271,2.33065534246316));
#12107=CARTESIAN_POINT('Ctrl Pts',(-206.381103690885,92.731204658208,2.27768590286173));
#12108=CARTESIAN_POINT('Ctrl Pts',(-206.921322261313,93.3666795522678,2.22471646326029));
#12109=CARTESIAN_POINT('Ctrl Pts',(-207.46154083174,94.0021544463277,2.17174702365886));
#12110=CARTESIAN_POINT('Ctrl Pts',(-207.655236916725,94.9322090517666,2.11877758405742));
#12111=CARTESIAN_POINT('Ctrl Pts',(-207.413621413596,95.730511049215,2.06580814445599));
#12112=CARTESIAN_POINT('Ctrl Pts',(-207.172005910466,96.5288130466634,2.01283870485455));
#12113=CARTESIAN_POINT('Ctrl Pts',(-206.495078819221,97.1953624361213,1.95986926525312));
#12114=CARTESIAN_POINT('Ctrl Pts',(-205.693139528324,97.4246177066617,1.90689982565168));
#12115=CARTESIAN_POINT('Ctrl Pts',(-204.891200237426,97.6538729772021,1.85393038605024));
#12116=CARTESIAN_POINT('Ctrl Pts',(-203.964248746875,97.4458341288248,1.80096094644881));
#12117=CARTESIAN_POINT('Ctrl Pts',(-203.337194868197,96.8958629307826,1.74799150684737));
#12118=CARTESIAN_POINT('Ctrl Pts',(-202.80287268554,96.4272240770433,1.70285543872891));
#12119=CARTESIAN_POINT('Ctrl Pts',(-202.486306286811,95.7103079983322,1.65771937061044));
#12120=CARTESIAN_POINT('Ctrl Pts',(-202.480282650156,94.9980775783256,1.61258330249198));
#12121=CARTESIAN_POINT('Origin',(-205.,95.,9.));
#12122=CARTESIAN_POINT('',(-202.480223566112,95.0018649480296,0.612583302491977));
#12123=CARTESIAN_POINT('',(-202.485814060779,95.0013541851486,0.887416697508031));
#12124=CARTESIAN_POINT('',(-202.4825,95.,9.));
#12125=CARTESIAN_POINT('',(-206.913465996665,96.6359872033749,0.));
#12126=CARTESIAN_POINT('Ctrl Pts',(-202.480223566112,95.0018649480296,0.612583302491977));
#12127=CARTESIAN_POINT('Ctrl Pts',(-202.486186841973,94.2874533490054,0.567297187132291));
#12128=CARTESIAN_POINT('Ctrl Pts',(-202.805062530183,93.5684800237081,0.522011071772605));
#12129=CARTESIAN_POINT('Ctrl Pts',(-203.342523272204,93.0996259401887,0.476724956412919));
#12130=CARTESIAN_POINT('Ctrl Pts',(-203.971170575831,92.5512252248344,0.423755516811483));
#12131=CARTESIAN_POINT('Ctrl Pts',(-204.898866003489,92.3450148318929,0.370786077210047));
#12132=CARTESIAN_POINT('Ctrl Pts',(-205.70005254405,92.5769535947063,0.317816637608611));
#12133=CARTESIAN_POINT('Ctrl Pts',(-206.501239084611,92.8088923575197,0.264847198007175));
#12134=CARTESIAN_POINT('Ctrl Pts',(-207.175916738074,93.4789802760881,0.211877758405739));
#12135=CARTESIAN_POINT('Ctrl Pts',(-207.415094474449,94.2765455778558,0.158908318804303));
#12136=CARTESIAN_POINT('Ctrl Pts',(-207.654272210825,95.0741108796235,0.105938879202868));
#12137=CARTESIAN_POINT('Ctrl Pts',(-207.457950030113,95.9991535645904,0.0529694396014316));
#12138=CARTESIAN_POINT('Ctrl Pts',(-206.913465996665,96.6359872033749,-4.22296552189629E-15));
#12139=CARTESIAN_POINT('',(-203.082849217755,96.6387883341086,5.92619716121943E-15));
#12140=CARTESIAN_POINT('Origin',(-205.,95.,0.));
#12141=CARTESIAN_POINT('Ctrl Pts',(-203.082846187392,96.6387906377554,3.88578058618805E-15));
#12142=CARTESIAN_POINT('Ctrl Pts',(-203.61481511748,97.259358365042,0.0519060689145041));
#12143=CARTESIAN_POINT('Ctrl Pts',(-204.477409093976,97.5988875826691,0.103812137829004));
#12144=CARTESIAN_POINT('Ctrl Pts',(-205.289479051915,97.5049655305341,0.155718206743504));
#12145=CARTESIAN_POINT('Ctrl Pts',(-206.118185434207,97.4091193496953,0.20868764634494));
#12146=CARTESIAN_POINT('Ctrl Pts',(-206.894276478514,96.8618802331851,0.261657085946376));
#12147=CARTESIAN_POINT('Ctrl Pts',(-207.262506770502,96.113606687757,0.314626525547811));
#12148=CARTESIAN_POINT('Ctrl Pts',(-207.630737062491,95.365333142329,0.367595965149247));
#12149=CARTESIAN_POINT('Ctrl Pts',(-207.591106602161,94.4160251679831,0.420565404750683));
#12150=CARTESIAN_POINT('Ctrl Pts',(-207.161534857641,93.7010772548185,0.473534844352119));
#12151=CARTESIAN_POINT('Ctrl Pts',(-206.731963113121,92.9861293416538,0.526504283953555));
#12152=CARTESIAN_POINT('Ctrl Pts',(-205.912450084411,92.5055414896703,0.57947372355499));
#12153=CARTESIAN_POINT('Ctrl Pts',(-205.078775376487,92.4794977945143,0.632443163156426));
#12154=CARTESIAN_POINT('Ctrl Pts',(-204.245100668563,92.4534540993582,0.685412602757862));
#12155=CARTESIAN_POINT('Ctrl Pts',(-203.397264281424,92.8819545610296,0.738382042359298));
#12156=CARTESIAN_POINT('Ctrl Pts',(-202.923851916981,93.568632431485,0.791351481960734));
#12157=CARTESIAN_POINT('Ctrl Pts',(-202.637658839267,93.9837514015503,0.823373220476499));
#12158=CARTESIAN_POINT('Ctrl Pts',(-202.488302515099,94.4932237151927,0.855394958992265));
#12159=CARTESIAN_POINT('Ctrl Pts',(-202.485814060779,95.0013541851486,0.887416697508031));
#12160=CARTESIAN_POINT('Origin',(-205.,95.,-2.20842344717744));
#12161=CARTESIAN_POINT('',(-201.921316320141,95.0000395558662,16.2084234471775));
#12162=CARTESIAN_POINT('',(-201.931367598206,95.0007780422787,16.2915765528226));
#12163=CARTESIAN_POINT('',(-201.9265,95.0000000000003,-2.20842344717744));
#12164=CARTESIAN_POINT('',(-205.793799282533,92.0307770462543,17.));
#12165=CARTESIAN_POINT('Ctrl Pts',(-201.931367598206,95.0007780422787,16.2915765528226));
#12166=CARTESIAN_POINT('Ctrl Pts',(-201.930437927868,95.4711408136525,16.315839943476));
#12167=CARTESIAN_POINT('Ctrl Pts',(-202.253352122202,96.9670518748459,16.3930727737308));
#12168=CARTESIAN_POINT('Ctrl Pts',(-204.582352684019,98.6092822369636,16.5232750435871));
#12169=CARTESIAN_POINT('Ctrl Pts',(-207.810248235069,97.3070699809007,16.6821833623914));
#12170=CARTESIAN_POINT('Ctrl Pts',(-208.45646174186,93.8848225849406,16.8410916811957));
#12171=CARTESIAN_POINT('Ctrl Pts',(-206.782006578242,92.2949667869871,16.9470305603986));
#12172=CARTESIAN_POINT('Ctrl Pts',(-205.793799282533,92.0307770462543,17.));
#12173=CARTESIAN_POINT('',(-204.206200717467,92.0307770462543,17.));
#12174=CARTESIAN_POINT('Origin',(-205.,95.,17.));
#12175=CARTESIAN_POINT('Ctrl Pts',(-201.921316320141,95.0000395558662,16.2084234471775));
#12176=CARTESIAN_POINT('Ctrl Pts',(-201.921316128699,95.0014817728825,16.2084984707981));
#12177=CARTESIAN_POINT('Ctrl Pts',(-201.92196781021,96.0211820960645,16.2615429340201));
#12178=CARTESIAN_POINT('Ctrl Pts',(-203.036134055811,98.0574883854641,16.3675568368436));
#12179=CARTESIAN_POINT('Ctrl Pts',(-206.506730950831,98.3071022816236,16.5264651556479));
#12180=CARTESIAN_POINT('Ctrl Pts',(-208.595808661615,95.5240011654517,16.6853734744522));
#12181=CARTESIAN_POINT('Ctrl Pts',(-207.39670926564,92.2839837126632,16.8432184225696));
#12182=CARTESIAN_POINT('Ctrl Pts',(-205.168796249957,91.7689270082682,16.9480939310855));
#12183=CARTESIAN_POINT('Ctrl Pts',(-204.204429069408,92.0254062069443,17.));
#12184=CARTESIAN_POINT('Origin',(-205.,95.,-2.20842344717744));
#12185=CARTESIAN_POINT('',(-201.928214587435,95.0026730804178,15.2084234471775));
#12186=CARTESIAN_POINT('',(-201.926872884582,94.997179525272,15.2915765528226));
#12187=CARTESIAN_POINT('',(-201.9265,95.0000000000003,-2.20842344717744));
#12188=CARTESIAN_POINT('Ctrl Pts',(-201.926872884582,94.997179525272,15.2915765528226));
#12189=CARTESIAN_POINT('Ctrl Pts',(-201.933847634293,95.7655075466895,15.3313566392007));
#12190=CARTESIAN_POINT('Ctrl Pts',(-202.614657640989,97.5679292031576,15.4241061651802));
#12191=CARTESIAN_POINT('Ctrl Pts',(-205.64160296068,98.5768482546894,15.5698251307612));
#12192=CARTESIAN_POINT('Ctrl Pts',(-208.354341794396,96.3979033358336,15.7287334495655));
#12193=CARTESIAN_POINT('Ctrl Pts',(-207.991790848075,92.937312201061,15.8876417683699));
#12194=CARTESIAN_POINT('Ctrl Pts',(-204.886537417199,91.367902630111,16.0465500871741));
#12195=CARTESIAN_POINT('Ctrl Pts',(-202.343315689682,92.8593267432967,16.1811950153251));
#12196=CARTESIAN_POINT('Ctrl Pts',(-201.932467492388,94.4442912374762,16.2628705038745));
#12197=CARTESIAN_POINT('Ctrl Pts',(-201.931367598206,95.0007780422787,16.2915765528226));
#12198=CARTESIAN_POINT('Ctrl Pts',(-201.928214587436,95.0026730804178,15.2084234471775));
#12199=CARTESIAN_POINT('Ctrl Pts',(-201.925712666175,95.3041515486696,15.2240151665228));
#12200=CARTESIAN_POINT('Ctrl Pts',(-202.105035887535,96.626924896284,15.2925763254696));
#12201=CARTESIAN_POINT('Ctrl Pts',(-204.001156184096,98.4939765214113,15.4141069240178));
#12202=CARTESIAN_POINT('Ctrl Pts',(-207.396173510293,97.7320213368001,15.573015242822));
#12203=CARTESIAN_POINT('Ctrl Pts',(-208.594403628795,94.4653692735856,15.7319235616264));
#12204=CARTESIAN_POINT('Ctrl Pts',(-206.497329046882,91.688881880511,15.8908318804307));
#12205=CARTESIAN_POINT('Ctrl Pts',(-203.029149056991,91.947824442261,16.0496651756144));
#12206=CARTESIAN_POINT('Ctrl Pts',(-201.9214512941,93.9832234360713,16.1555290311966));
#12207=CARTESIAN_POINT('Ctrl Pts',(-201.921316320141,95.0000395558662,16.2084234471775));
#12208=CARTESIAN_POINT('Origin',(-205.,95.,-2.20842344717744));
#12209=CARTESIAN_POINT('',(-201.93080706636,94.9985876431865,14.2084234471775));
#12210=CARTESIAN_POINT('',(-201.921581992455,95.0008245399417,14.2915765528226));
#12211=CARTESIAN_POINT('',(-201.9265,95.0000000000003,-2.20842344717744));
#12212=CARTESIAN_POINT('Ctrl Pts',(-201.921581992455,95.0008245399417,14.2915765528226));
#12213=CARTESIAN_POINT('Ctrl Pts',(-201.92142212516,95.0455752780765,14.293903895324));
#12214=CARTESIAN_POINT('Ctrl Pts',(-201.942596684159,96.1086813249517,14.3492006774268));
#12215=CARTESIAN_POINT('Ctrl Pts',(-203.167697507449,98.1381902248446,14.4574668991311));
#12216=CARTESIAN_POINT('Ctrl Pts',(-206.645679958249,98.2399547180336,14.6163752179354));
#12217=CARTESIAN_POINT('Ctrl Pts',(-208.614921829979,95.3713653348348,14.7752835367397));
#12218=CARTESIAN_POINT('Ctrl Pts',(-207.270042916896,92.1623115429714,14.934191855544));
#12219=CARTESIAN_POINT('Ctrl Pts',(-203.844015795661,91.5548205083004,15.0931001743483));
#12220=CARTESIAN_POINT('Ctrl Pts',(-202.07012706505,93.4672252077733,15.2122284067745));
#12221=CARTESIAN_POINT('Ctrl Pts',(-201.924560359749,94.7424352401662,15.2783871995992));
#12222=CARTESIAN_POINT('Ctrl Pts',(-201.926872884582,94.997179525272,15.2915765528226));
#12223=CARTESIAN_POINT('Ctrl Pts',(-201.93080706636,94.9985876431865,14.2084234471775));
#12224=CARTESIAN_POINT('Ctrl Pts',(-201.933303438965,95.6013727123389,14.2395318622475));
#12225=CARTESIAN_POINT('Ctrl Pts',(-202.396531802648,97.2340830995271,14.323609716919));
#12226=CARTESIAN_POINT('Ctrl Pts',(-205.05099675704,98.6335890076928,14.4606570111919));
#12227=CARTESIAN_POINT('Ctrl Pts',(-208.082133999653,96.9251026119764,14.6195653299962));
#12228=CARTESIAN_POINT('Ctrl Pts',(-208.287605212672,93.451703526775,14.7784736488005));
#12229=CARTESIAN_POINT('Ctrl Pts',(-205.479036767596,91.3977656146854,14.9373819676048));
#12230=CARTESIAN_POINT('Ctrl Pts',(-202.549953847218,92.5238105299853,15.0806985670638));
#12231=CARTESIAN_POINT('Ctrl Pts',(-201.934212393764,94.2799447141626,15.1710457269214));
#12232=CARTESIAN_POINT('Ctrl Pts',(-201.928214587436,95.0026730804178,15.2084234471775));
#12233=CARTESIAN_POINT('Origin',(-205.,95.,-2.20842344717744));
#12234=CARTESIAN_POINT('',(-201.923038042999,94.9979784085099,13.2084234471775));
#12235=CARTESIAN_POINT('',(-201.92933278587,95.0023490188139,13.2915765528226));
#12236=CARTESIAN_POINT('',(-201.9265,95.0000000000003,-2.20842344717744));
#12237=CARTESIAN_POINT('Ctrl Pts',(-201.92933278587,95.0023490188139,13.2915765528226));
#12238=CARTESIAN_POINT('Ctrl Pts',(-201.926879380047,95.3476951209313,13.3094205910487));
#12239=CARTESIAN_POINT('Ctrl Pts',(-202.140117503338,96.7152487840609,13.3802340688762));
#12240=CARTESIAN_POINT('Ctrl Pts',(-204.150349511013,98.5332229241514,13.5040169863052));
#12241=CARTESIAN_POINT('Ctrl Pts',(-207.50996737673,97.6278572896369,13.6629253051096));
#12242=CARTESIAN_POINT('Ctrl Pts',(-208.568475210139,94.3133014680822,13.8218336239139));
#12243=CARTESIAN_POINT('Ctrl Pts',(-206.355444844063,91.6283031749969,13.9807419427182));
#12244=CARTESIAN_POINT('Ctrl Pts',(-202.95036918439,92.0284906781176,14.1373229190211));
#12245=CARTESIAN_POINT('Ctrl Pts',(-201.925060644632,94.0270653169006,14.2409344557225));
#12246=CARTESIAN_POINT('Ctrl Pts',(-201.921581992455,95.0008245399417,14.2915765528226));
#12247=CARTESIAN_POINT('Ctrl Pts',(-201.923038042999,94.9979784085099,13.2084234471775));
#12248=CARTESIAN_POINT('Ctrl Pts',(-201.929861215503,95.8956190998097,13.2550485579722));
#12249=CARTESIAN_POINT('Ctrl Pts',(-202.817787070614,97.8247938063492,13.3546431083684));
#12250=CARTESIAN_POINT('Ctrl Pts',(-206.096505488088,98.4645700435054,13.5072070983661));
#12251=CARTESIAN_POINT('Ctrl Pts',(-208.506304474045,95.9546720956722,13.6661154171704));
#12252=CARTESIAN_POINT('Ctrl Pts',(-207.701562707091,92.569541439018,13.8250237359747));
#12253=CARTESIAN_POINT('Ctrl Pts',(-204.420058445801,91.4126280298156,13.983932054779));
#12254=CARTESIAN_POINT('Ctrl Pts',(-202.208551988368,93.1272197714318,14.1117319585132));
#12255=CARTESIAN_POINT('Ctrl Pts',(-201.929052773747,94.5749884609644,14.1865624226461));
#12256=CARTESIAN_POINT('Ctrl Pts',(-201.93080706636,94.9985876431865,14.2084234471775));
#12257=CARTESIAN_POINT('Origin',(-205.,95.,-2.20842344717744));
#12258=CARTESIAN_POINT('',(-201.924530362794,95.0025681813082,12.2084234471775));
#12259=CARTESIAN_POINT('',(-201.930073873701,94.9980134193687,12.2915765528226));
#12260=CARTESIAN_POINT('',(-201.9265,95.0000000000003,-2.20842344717744));
#12261=CARTESIAN_POINT('Ctrl Pts',(-201.930073873701,94.9980134193687,12.2915765528226));
#12262=CARTESIAN_POINT('Ctrl Pts',(-201.933893697005,95.6440549307384,12.3249372867734));
#12263=CARTESIAN_POINT('Ctrl Pts',(-202.44913572334,97.3214395549061,12.4112674603257));
#12264=CARTESIAN_POINT('Ctrl Pts',(-205.205169260054,98.628150459449,12.5505670734794));
#12265=CARTESIAN_POINT('Ctrl Pts',(-208.161062843079,96.7925545691908,12.7094753922837));
#12266=CARTESIAN_POINT('Ctrl Pts',(-208.218929342183,93.3135646849756,12.868383711088));
#12267=CARTESIAN_POINT('Ctrl Pts',(-205.325717397541,91.3806798485012,13.0272920298923));
#12268=CARTESIAN_POINT('Ctrl Pts',(-202.492306008035,92.6103936505881,13.1683563104705));
#12269=CARTESIAN_POINT('Ctrl Pts',(-201.934162234404,94.3225465942424,13.2564511514472));
#12270=CARTESIAN_POINT('Ctrl Pts',(-201.92933278587,95.0023490188139,13.2915765528226));
#12271=CARTESIAN_POINT('Ctrl Pts',(-201.924530362794,95.0025681813082,12.2084234471775));
#12272=CARTESIAN_POINT('Ctrl Pts',(-201.922946673736,95.1793804353838,12.2175958140955));
#12273=CARTESIAN_POINT('Ctrl Pts',(-202.017340654133,96.3755745120124,12.279737620615));
#12274=CARTESIAN_POINT('Ctrl Pts',(-203.586712632674,98.3478633022839,12.3948488667359));
#12275=CARTESIAN_POINT('Ctrl Pts',(-207.048879131051,98.0012770914624,12.5537571855402));
#12276=CARTESIAN_POINT('Ctrl Pts',(-208.632656141981,94.9031535878521,12.7126655043445));
#12277=CARTESIAN_POINT('Ctrl Pts',(-206.886054603385,91.8938177924453,12.8715738231489));
#12278=CARTESIAN_POINT('Ctrl Pts',(-203.410339284457,91.7321951278126,13.0304821419532));
#12279=CARTESIAN_POINT('Ctrl Pts',(-201.98420370222,93.734861145707,13.1427653499627));
#12280=CARTESIAN_POINT('Ctrl Pts',(-201.922109606602,94.8758354773988,13.2020791183708));
#12281=CARTESIAN_POINT('Ctrl Pts',(-201.923038042999,94.9979784085099,13.2084234471775));
#12282=CARTESIAN_POINT('Origin',(-205.,95.,-2.20842344717744));
#12283=CARTESIAN_POINT('',(-201.931339695558,95.0005697559146,11.2084234471775));
#12284=CARTESIAN_POINT('',(-201.922093771296,94.9986005590476,11.2915765528226));
#12285=CARTESIAN_POINT('',(-201.9265,95.0000000000003,-2.20842344717744));
#12286=CARTESIAN_POINT('Ctrl Pts',(-201.922093771296,94.9986005590477,11.2915765528226));
#12287=CARTESIAN_POINT('Ctrl Pts',(-201.927419218831,95.9388438143246,11.3404539824981));
#12288=CARTESIAN_POINT('Ctrl Pts',(-202.890883267115,97.9074847478091,11.4423008517751));
#12289=CARTESIAN_POINT('Ctrl Pts',(-206.242562324195,98.4149098161,11.5971171606536));
#12290=CARTESIAN_POINT('Ctrl Pts',(-208.543663659863,95.8049956815827,11.7560254794579));
#12291=CARTESIAN_POINT('Ctrl Pts',(-207.595973758966,92.4570705034615,11.9149337982622));
#12292=CARTESIAN_POINT('Ctrl Pts',(-204.268324130509,91.4404746659679,12.0738421170665));
#12293=CARTESIAN_POINT('Ctrl Pts',(-202.169239397251,93.215538627184,12.19938970192));
#12294=CARTESIAN_POINT('Ctrl Pts',(-201.927828665579,94.6182844285985,12.271967847172));
#12295=CARTESIAN_POINT('Ctrl Pts',(-201.930073873701,94.9980134193687,12.2915765528226));
#12296=CARTESIAN_POINT('Ctrl Pts',(-201.931339695558,95.0005697559146,11.2084234471775));
#12297=CARTESIAN_POINT('Ctrl Pts',(-201.930548312084,95.4791749823821,11.2331125098202));
#12298=CARTESIAN_POINT('Ctrl Pts',(-202.261413021211,96.983573743505,11.3107710120644));
#12299=CARTESIAN_POINT('Ctrl Pts',(-204.612024672262,98.6131765827982,11.4413989539101));
#12300=CARTESIAN_POINT('Ctrl Pts',(-207.827224888828,97.2830613880067,11.6003072727144));
#12301=CARTESIAN_POINT('Ctrl Pts',(-208.450456926625,93.8598610299961,11.7592155915187));
#12302=CARTESIAN_POINT('Ctrl Pts',(-205.910348619136,91.4819273365871,11.918123910323));
#12303=CARTESIAN_POINT('Ctrl Pts',(-202.730434684324,92.2804106896555,12.0678598622093));
#12304=CARTESIAN_POINT('Ctrl Pts',(-201.932092308952,94.1583085466637,12.1646263744941));
#12305=CARTESIAN_POINT('Ctrl Pts',(-201.924530362794,95.0025681813082,12.2084234471775));
#12306=CARTESIAN_POINT('Origin',(-205.,95.,-2.20842344717744));
#12307=CARTESIAN_POINT('',(-201.926625303462,94.9971761042889,10.2084234471775));
#12308=CARTESIAN_POINT('',(-201.925838932402,95.0027879332515,10.2915765528226));
#12309=CARTESIAN_POINT('',(-201.9265,95.0000000000003,-2.20842344717744));
#12310=CARTESIAN_POINT('Ctrl Pts',(-201.925838932402,95.0027879332515,10.2915765528226));
#12311=CARTESIAN_POINT('Ctrl Pts',(-201.923796745295,95.2232588384768,10.3030012386214));
#12312=CARTESIAN_POINT('Ctrl Pts',(-202.046093760276,96.4636737691049,10.3673953640217));
#12313=CARTESIAN_POINT('Ctrl Pts',(-203.730077660409,98.4048300152887,10.4847589290234));
#12314=CARTESIAN_POINT('Ctrl Pts',(-207.174414514723,97.9116132469416,10.6436672478277));
#12315=CARTESIAN_POINT('Ctrl Pts',(-208.625272444921,94.7490619962975,10.802575566632));
#12316=CARTESIAN_POINT('Ctrl Pts',(-206.752521116536,91.8165679027658,10.9614838854363));
#12317=CARTESIAN_POINT('Ctrl Pts',(-203.273078016077,91.802608775416,11.1203922042406));
#12318=CARTESIAN_POINT('Ctrl Pts',(-201.96010201747,93.8226489641406,11.2304230933694));
#12319=CARTESIAN_POINT('Ctrl Pts',(-201.921647925753,94.91988355697,11.2874845428967));
#12320=CARTESIAN_POINT('Ctrl Pts',(-201.922093771296,94.9986005590477,11.2915765528226));
#12321=CARTESIAN_POINT('Ctrl Pts',(-201.926625303462,94.9971761042889,10.2084234471775));
#12322=CARTESIAN_POINT('Ctrl Pts',(-201.933732013081,95.7735654381765,10.248629205545));
#12323=CARTESIAN_POINT('Ctrl Pts',(-202.626469706802,97.5841063658898,10.3418044035139));
#12324=CARTESIAN_POINT('Ctrl Pts',(-205.670290596122,98.5715935365275,10.4879490410842));
#12325=CARTESIAN_POINT('Ctrl Pts',(-208.365431557495,96.3709268052048,10.6468573598885));
#12326=CARTESIAN_POINT('Ctrl Pts',(-207.975182481689,92.9134097014358,10.8057656786928));
#12327=CARTESIAN_POINT('Ctrl Pts',(-204.85731935967,91.3688552620022,10.9646739974972));
#12328=CARTESIAN_POINT('Ctrl Pts',(-202.334353177571,92.8760513997145,11.0988932536587));
#12329=CARTESIAN_POINT('Ctrl Pts',(-201.932246195058,94.4523457745213,11.1801430702188));
#12330=CARTESIAN_POINT('Ctrl Pts',(-201.931339695558,95.0005697559146,11.2084234471775));
#12331=CARTESIAN_POINT('Origin',(-205.,95.,-2.20842344717744));
#12332=CARTESIAN_POINT('',(-201.921683798062,95.0009686894698,9.20842344717747));
#12333=CARTESIAN_POINT('',(-201.931429646185,94.9998541961964,9.29157655282255));
#12334=CARTESIAN_POINT('',(-201.9265,95.0000000000003,-2.20842344717744));
#12335=CARTESIAN_POINT('Ctrl Pts',(-201.931429646185,94.9998541961964,9.29157655282255));
#12336=CARTESIAN_POINT('Ctrl Pts',(-201.931650280968,95.5221595342362,9.31851793434612));
#12337=CARTESIAN_POINT('Ctrl Pts',(-202.306382592467,97.0716662514915,9.39842875547113));
#12338=CARTESIAN_POINT('Ctrl Pts',(-204.765726364391,98.6263874648557,9.53130901619759));
#12339=CARTESIAN_POINT('Ctrl Pts',(-207.92157608408,97.1610098025081,9.69021733500189));
#12340=CARTESIAN_POINT('Ctrl Pts',(-208.398957503736,93.7144425063808,9.84912565380619));
#12341=CARTESIAN_POINT('Ctrl Pts',(-205.760212673412,91.4464599519933,10.0080339726105));
#12342=CARTESIAN_POINT('Ctrl Pts',(-202.664332879748,92.3651571515322,10.155517605616));
#12343=CARTESIAN_POINT('Ctrl Pts',(-201.933265146311,94.2010670247312,10.25003179902));
#12344=CARTESIAN_POINT('Ctrl Pts',(-201.925838932402,95.0027879332515,10.2915765528226));
#12345=CARTESIAN_POINT('Ctrl Pts',(-201.921683798062,95.0009686894698,9.20842344717747));
#12346=CARTESIAN_POINT('Ctrl Pts',(-201.921465439927,95.0539090268706,9.21117646166824));
#12347=CARTESIAN_POINT('Ctrl Pts',(-201.946710182927,96.1252365864707,9.26689891576045));
#12348=CARTESIAN_POINT('Ctrl Pts',(-203.192936169305,98.1527908565597,9.37559080945409));
#12349=CARTESIAN_POINT('Ctrl Pts',(-206.671623315332,98.2266461481009,9.5344991282584));
#12350=CARTESIAN_POINT('Ctrl Pts',(-208.617784889251,95.3423483146199,9.6934074470627));
#12351=CARTESIAN_POINT('Ctrl Pts',(-207.247201711938,92.1441893726518,9.85231576586701));
#12352=CARTESIAN_POINT('Ctrl Pts',(-203.81640912163,91.5642056950316,10.0112240846713));
#12353=CARTESIAN_POINT('Ctrl Pts',(-202.064207753662,93.4838999616225,10.1299266451081));
#12354=CARTESIAN_POINT('Ctrl Pts',(-201.924369214287,94.7507042959325,10.1956597659435));
#12355=CARTESIAN_POINT('Ctrl Pts',(-201.926625303462,94.9971761042889,10.2084234471775));
#12356=CARTESIAN_POINT('Origin',(-205.,95.,-2.20842344717744));
#12357=CARTESIAN_POINT('',(-201.92952365041,95.0022696654447,8.20842344717746));
#12358=CARTESIAN_POINT('',(-201.925302573121,94.9972772020656,8.29157655282255));
#12359=CARTESIAN_POINT('',(-201.9265,95.0000000000003,-2.20842344717744));
#12360=CARTESIAN_POINT('Ctrl Pts',(-201.925302573121,94.9972772020656,8.29157655282255));
#12361=CARTESIAN_POINT('Ctrl Pts',(-201.932850267835,95.8162560531386,8.33403463007084));
#12362=CARTESIAN_POINT('Ctrl Pts',(-202.690770542377,97.6693023124736,8.42946214692058));
#12363=CARTESIAN_POINT('Ctrl Pts',(-205.821273824104,98.5399264805142,8.57785910337175));
#12364=CARTESIAN_POINT('Ctrl Pts',(-208.420584553779,96.2268543075893,8.73676742217604));
#12365=CARTESIAN_POINT('Ctrl Pts',(-207.883941595716,92.7890158177634,8.89567574098036));
#12366=CARTESIAN_POINT('Ctrl Pts',(-204.70333321592,91.3781829144989,9.05458405978466));
#12367=CARTESIAN_POINT('Ctrl Pts',(-202.2878355418,92.9640356234163,9.1865509970654));
#12368=CARTESIAN_POINT('Ctrl Pts',(-201.931216491008,94.4952552148495,9.26554849474469));
#12369=CARTESIAN_POINT('Ctrl Pts',(-201.931429646185,94.9998541961964,9.29157655282255));
#12370=CARTESIAN_POINT('Ctrl Pts',(-201.92952365041,95.0022696654447,8.20842344717746));
#12371=CARTESIAN_POINT('Ctrl Pts',(-201.927106416298,95.3559093360916,8.22669315739296));
#12372=CARTESIAN_POINT('Ctrl Pts',(-202.147009294539,96.7319441344973,8.29793230720989));
#12373=CARTESIAN_POINT('Ctrl Pts',(-204.17872618548,98.5399264392071,8.42214089662825));
#12374=CARTESIAN_POINT('Ctrl Pts',(-207.530971538769,97.6076335907019,8.58104921543256));
#12375=CARTESIAN_POINT('Ctrl Pts',(-208.56285047346,94.2846914112228,8.73995753423687));
#12376=CARTESIAN_POINT('Ctrl Pts',(-206.328347915327,91.6175361510784,8.89886585304118));
#12377=CARTESIAN_POINT('Ctrl Pts',(-202.935840661412,92.0438696918247,9.0550211573547));
#12378=CARTESIAN_POINT('Ctrl Pts',(-201.925666764731,94.0353092287831,9.1582070220668));
#12379=CARTESIAN_POINT('Ctrl Pts',(-201.921683798062,95.0009686894698,9.20842344717747));
#12380=CARTESIAN_POINT('Origin',(-205.,95.,-2.20842344717744));
#12381=CARTESIAN_POINT('',(-201.929907579326,94.9979181687661,7.20842344717746));
#12382=CARTESIAN_POINT('',(-201.922442628529,95.0016691002816,7.29157655282255));
#12383=CARTESIAN_POINT('',(-201.9265,95.0000000000003,-2.20842344717744));
#12384=CARTESIAN_POINT('Ctrl Pts',(-201.922442628529,95.0016691002816,7.29157655282255));
#12385=CARTESIAN_POINT('Ctrl Pts',(-201.921812166908,95.0979843181188,7.29658188619413));
#12386=CARTESIAN_POINT('Ctrl Pts',(-201.96963492335,96.2129306162495,7.35455665916715));
#12387=CARTESIAN_POINT('Ctrl Pts',(-203.328376665162,98.2266461857523,7.46550087174159));
#12388=CARTESIAN_POINT('Ctrl Pts',(-206.807063851782,98.1527908933495,7.6244091905459));
#12389=CARTESIAN_POINT('Ctrl Pts',(-208.629055096267,95.1884921480159,7.78331750935021));
#12390=CARTESIAN_POINT('Ctrl Pts',(-207.123969189693,92.0513859081191,7.94222582815452));
#12391=CARTESIAN_POINT('Ctrl Pts',(-203.671652069173,91.6175361116086,8.10113414695882));
#12392=CARTESIAN_POINT('Ctrl Pts',(-202.034177280902,93.5720648629822,8.21758438851483));
#12393=CARTESIAN_POINT('Ctrl Pts',(-201.923433987467,94.794522296024,8.28106519046941));
#12394=CARTESIAN_POINT('Ctrl Pts',(-201.925302573121,94.9972772020656,8.29157655282255));
#12395=CARTESIAN_POINT('Ctrl Pts',(-201.929907579326,94.9979181687661,7.20842344717746));
#12396=CARTESIAN_POINT('Ctrl Pts',(-201.933975313296,95.6521139982133,7.24220985311768));
#12397=CARTESIAN_POINT('Ctrl Pts',(-202.459390605198,97.3379066754947,7.32896569865933));
#12398=CARTESIAN_POINT('Ctrl Pts',(-205.234273632875,98.6263874225397,7.46869098380241));
#12399=CARTESIAN_POINT('Ctrl Pts',(-208.175343867546,96.7671336101861,7.62759930260672));
#12400=CARTESIAN_POINT('Ctrl Pts',(-208.205294334613,93.2877914549009,7.78650762141103));
#12401=CARTESIAN_POINT('Ctrl Pts',(-205.296666780619,91.3781829567617,7.94541594021533));
#12402=CARTESIAN_POINT('Ctrl Pts',(-202.481733395465,92.6268122018764,8.08605454880414));
#12403=CARTESIAN_POINT('Ctrl Pts',(-201.934114712258,94.3306005077602,8.17372371779152));
#12404=CARTESIAN_POINT('Ctrl Pts',(-201.92952365041,95.0022696654447,8.20842344717746));
#12405=CARTESIAN_POINT('Origin',(-205.,95.,-2.20842344717744));
#12406=CARTESIAN_POINT('',(-201.921949534001,94.9987333291051,6.20842344717746));
#12407=CARTESIAN_POINT('',(-201.930401901847,95.0017670788574,6.29157655282255));
#12408=CARTESIAN_POINT('',(-201.9265,95.0000000000003,-2.20842344717744));
#12409=CARTESIAN_POINT('Ctrl Pts',(-201.930401901847,95.0017670788574,6.29157655282255));
#12410=CARTESIAN_POINT('Ctrl Pts',(-201.928325311163,95.3992893406063,6.31209858191885));
#12411=CARTESIAN_POINT('Ctrl Pts',(-202.184887900799,96.8202798707259,6.38559005061658));
#12412=CARTESIAN_POINT('Ctrl Pts',(-204.329709396056,98.5715935782041,6.51205095891576));
#12413=CARTESIAN_POINT('Ctrl Pts',(-207.639365322875,97.4978632616717,6.67095927772006));
#12414=CARTESIAN_POINT('Ctrl Pts',(-208.529280621322,94.13411982494,6.82986759652437));
#12415=CARTESIAN_POINT('Ctrl Pts',(-206.183590892181,91.5642056549396,6.98877591532867));
#12416=CARTESIAN_POINT('Ctrl Pts',(-202.86086221326,92.1259208703621,7.1426789007614));
#12417=CARTESIAN_POINT('Ctrl Pts',(-201.928484089891,94.0787189195554,7.2436124465927));
#12418=CARTESIAN_POINT('Ctrl Pts',(-201.922442628529,95.0016691002816,7.29157655282255));
#12419=CARTESIAN_POINT('Ctrl Pts',(-201.921949534001,94.9987333291051,6.20842344717746));
#12420=CARTESIAN_POINT('Ctrl Pts',(-201.926887133532,95.9470473025757,6.2577265488424));
#12421=CARTESIAN_POINT('Ctrl Pts',(-202.905053362444,97.9229927262678,6.35999909010877));
#12422=CARTESIAN_POINT('Ctrl Pts',(-206.269922324772,98.4048299755582,6.51524107097657));
#12423=CARTESIAN_POINT('Ctrl Pts',(-208.550008545203,95.7765366716391,6.67414938978089));
#12424=CARTESIAN_POINT('Ctrl Pts',(-207.575486609103,92.4363232263514,6.83305770858518));
#12425=CARTESIAN_POINT('Ctrl Pts',(-204.239787335459,91.4464599934592,6.9919660273895));
#12426=CARTESIAN_POINT('Ctrl Pts',(-202.162081150144,93.2322337929133,7.11708794025358));
#12427=CARTESIAN_POINT('Ctrl Pts',(-201.927598026844,94.6264829637453,7.18924041351624));
#12428=CARTESIAN_POINT('Ctrl Pts',(-201.929907579326,94.9979181687661,7.20842344717746));
#12429=CARTESIAN_POINT('Origin',(-205.,95.,-2.20842344717744));
#12430=CARTESIAN_POINT('',(-201.926089603319,95.0028070295978,5.20842344717746));
#12431=CARTESIAN_POINT('',(-201.928899948926,94.9974995292963,5.29157655282255));
#12432=CARTESIAN_POINT('',(-201.9265,95.0000000000003,-2.20842344717744));
#12433=CARTESIAN_POINT('Ctrl Pts',(-201.928899948926,94.9974995292963,5.29157655282255));
#12434=CARTESIAN_POINT('Ctrl Pts',(-201.934224719147,95.6947303578001,5.32761527764357));
#12435=CARTESIAN_POINT('Ctrl Pts',(-202.515335108225,97.4247770996434,5.41662344206602));
#12436=CARTESIAN_POINT('Ctrl Pts',(-205.387975332266,98.61317662496,5.55860104608992));
#12437=CARTESIAN_POINT('Ctrl Pts',(-208.247484138049,96.6307718892372,5.71750936489422));
#12438=CARTESIAN_POINT('Ctrl Pts',(-208.129735782527,93.1532937122619,5.87641768369853));
#12439=CARTESIAN_POINT('Ctrl Pts',(-205.142680641995,91.3688552196306,6.03532600250283));
#12440=CARTESIAN_POINT('Ctrl Pts',(-202.427470276955,92.7139399969898,6.17371229221084));
#12441=CARTESIAN_POINT('Ctrl Pts',(-201.933685202442,94.3732440438608,6.25912914231741));
#12442=CARTESIAN_POINT('Ctrl Pts',(-201.930401901847,95.0017670788574,6.29157655282255));
#12443=CARTESIAN_POINT('Ctrl Pts',(-201.926089603319,95.0028070295978,5.20842344717746));
#12444=CARTESIAN_POINT('Ctrl Pts',(-201.923973722235,95.2315402412545,5.22027380496568));
#12445=CARTESIAN_POINT('Ctrl Pts',(-202.0517688528,96.4803364748475,5.28509360235534));
#12446=CARTESIAN_POINT('Ctrl Pts',(-203.757437690304,98.4149097762516,5.40288283934642));
#12447=CARTESIAN_POINT('Ctrl Pts',(-207.197706236788,97.8940727651868,5.56179115815073));
#12448=CARTESIAN_POINT('Ctrl Pts',(-208.623142268693,94.7199821894518,5.72069947695504));
#12449=CARTESIAN_POINT('Ctrl Pts',(-206.726921963772,91.8026088127262,5.87960779575934));
#12450=CARTESIAN_POINT('Ctrl Pts',(-203.247478903914,91.8165679399129,6.03851611456365));
#12451=CARTESIAN_POINT('Ctrl Pts',(-201.955769853407,93.8392225784452,6.14812133170302));
#12452=CARTESIAN_POINT('Ctrl Pts',(-201.921582358147,94.9282136380667,6.20475710924096));
#12453=CARTESIAN_POINT('Ctrl Pts',(-201.921949534001,94.9987333291051,6.20842344717746));
#12454=CARTESIAN_POINT('Origin',(-205.,95.,-2.20842344717744));
#12455=CARTESIAN_POINT('',(-201.931412642297,94.9997186182815,4.20842344717746));
#12456=CARTESIAN_POINT('',(-201.921415661854,94.9994934750605,4.29157655282255));
#12457=CARTESIAN_POINT('',(-201.9265,95.0000000000003,-2.20842344717744));
#12458=CARTESIAN_POINT('Ctrl Pts',(-201.921415661854,94.9994934750605,4.29157655282255));
#12459=CARTESIAN_POINT('Ctrl Pts',(-201.923678538513,95.9906708985823,4.34313197336829));
#12460=CARTESIAN_POINT('Ctrl Pts',(-202.981928354028,98.0043611658593,4.44765683351546));
#12461=CARTESIAN_POINT('Ctrl Pts',(-206.413287383817,98.3478633413499,4.60515113326407));
#12462=CARTESIAN_POINT('Ctrl Pts',(-208.579767845133,95.6251658632375,4.76405945206838));
#12463=CARTESIAN_POINT('Ctrl Pts',(-207.464357156355,92.3293233090611,4.92296777087269));
#12464=CARTESIAN_POINT('Ctrl Pts',(-204.089651370241,91.481927295535,5.081876089677));
#12465=CARTESIAN_POINT('Ctrl Pts',(-202.125612719496,93.3205708167562,5.20474568366028));
#12466=CARTESIAN_POINT('Ctrl Pts',(-201.926398412972,94.6699458671693,5.27464583804213));
#12467=CARTESIAN_POINT('Ctrl Pts',(-201.928899948926,94.9974995292963,5.29157655282255));
#12468=CARTESIAN_POINT('Ctrl Pts',(-201.931412642297,94.9997186182815,4.20842344717746));
#12469=CARTESIAN_POINT('Ctrl Pts',(-201.931845298516,95.530268992426,4.2357905006904));
#12470=CARTESIAN_POINT('Ctrl Pts',(-202.31517360758,97.0882951016321,4.31612699380478));
#12471=CARTESIAN_POINT('Ctrl Pts',(-204.79483074234,98.6281504171124,4.44943292652058));
#12472=CARTESIAN_POINT('Ctrl Pts',(-207.938821173194,97.1374985345979,4.60834124532489));
#12473=CARTESIAN_POINT('Ctrl Pts',(-208.388533199045,93.6872118859588,4.76724956412919));
#12474=CARTESIAN_POINT('Ctrl Pts',(-205.731675860954,91.4404747075036,4.92615788293351));
#12475=CARTESIAN_POINT('Ctrl Pts',(-202.652180921301,92.3812593713882,5.07321584394959));
#12476=CARTESIAN_POINT('Ctrl Pts',(-201.933431414338,94.2091348205733,5.16730436536425));
#12477=CARTESIAN_POINT('Ctrl Pts',(-201.926089603319,95.0028070295978,5.20842344717746));
#12478=CARTESIAN_POINT('Origin',(-205.,95.,-2.20842344717744));
#12479=CARTESIAN_POINT('',(-201.925054591669,94.9973187846012,3.20842344717746));
#12480=CARTESIAN_POINT('',(-201.927395875445,95.0027899210604,3.29157655282255));
#12481=CARTESIAN_POINT('',(-201.9265,95.0000000000003,-2.20842344717744));
#12482=CARTESIAN_POINT('Ctrl Pts',(-201.927395875445,95.0027899210604,3.29157655282255));
#12483=CARTESIAN_POINT('Ctrl Pts',(-201.9249848093,95.2752922921681,3.30567922949157));
#12484=CARTESIAN_POINT('Ctrl Pts',(-202.083098781857,96.5685582167107,3.37275134576203));
#12485=CARTESIAN_POINT('Ctrl Pts',(-203.903494499117,98.4645700839332,3.49279290163393));
#12486=CARTESIAN_POINT('Ctrl Pts',(-207.318557500821,97.7981889317011,3.65170122043824));
#12487=CARTESIAN_POINT('Ctrl Pts',(-208.607992899891,94.5664594412711,3.81060953924254));
#12488=CARTESIAN_POINT('Ctrl Pts',(-206.589660734093,91.732195089681,3.96951785804685));
#12489=CARTESIAN_POINT('Ctrl Pts',(-203.113945374607,91.8938177561992,4.12842617685116));
#12490=CARTESIAN_POINT('Ctrl Pts',(-201.934002493894,93.9268197139999,4.23577907510972));
#12491=CARTESIAN_POINT('Ctrl Pts',(-201.921353597562,94.9723082877494,4.29016253376685));
#12492=CARTESIAN_POINT('Ctrl Pts',(-201.921415661854,94.9994934750605,4.29157655282255));
#12493=CARTESIAN_POINT('Ctrl Pts',(-201.925054591669,94.9973187846012,3.20842344717746));
#12494=CARTESIAN_POINT('Ctrl Pts',(-201.93262903552,95.8243366274881,3.25130719641512));
#12495=CARTESIAN_POINT('Ctrl Pts',(-202.703262931463,97.6853195581008,3.34716038525422));
#12496=CARTESIAN_POINT('Ctrl Pts',(-205.849650479072,98.5332228829228,3.49598301369474));
#12497=CARTESIAN_POINT('Ctrl Pts',(-208.430318245301,96.1993692554529,3.65489133249905));
#12498=CARTESIAN_POINT('Ctrl Pts',(-207.866108582956,92.7659473008752,3.81379965130336));
#12499=CARTESIAN_POINT('Ctrl Pts',(-204.67428260626,91.3806798907347,3.97270797010767));
#12500=CARTESIAN_POINT('Ctrl Pts',(-202.27933715358,92.9806849502469,4.10424923539903));
#12501=CARTESIAN_POINT('Ctrl Pts',(-201.93100788438,94.5033789041131,4.18282106108896));
#12502=CARTESIAN_POINT('Ctrl Pts',(-201.931412642297,94.9997186182815,4.20842344717746));
#12503=CARTESIAN_POINT('Origin',(-205.,95.,-2.20842344717744));
#12504=CARTESIAN_POINT('',(-201.922621915119,95.001787031353,2.20842344717746));
#12505=CARTESIAN_POINT('',(-201.931144181024,94.9990189299375,2.29157655282255));
#12506=CARTESIAN_POINT('',(-201.9265,95.0000000000003,-2.20842344717744));
#12507=CARTESIAN_POINT('Ctrl Pts',(-201.931144181024,94.9990189299375,2.29157655282255));
#12508=CARTESIAN_POINT('Ctrl Pts',(-201.932784831847,95.5731085049423,2.32119592521629));
#12509=CARTESIAN_POINT('Ctrl Pts',(-202.363262779912,97.1761484760171,2.40378473721147));
#12510=CARTESIAN_POINT('Ctrl Pts',(-204.949003242364,98.6335890500974,2.53934298880809));
#12511=CARTESIAN_POINT('Ctrl Pts',(-208.026893764665,97.0108417000006,2.69825130761239));
#12512=CARTESIAN_POINT('Ctrl Pts',(-208.329761920824,93.5445771233942,2.8571596264167));
#12513=CARTESIAN_POINT('Ctrl Pts',(-205.579941560967,91.4126279879542,3.01606794522101));
#12514=CARTESIAN_POINT('Ctrl Pts',(-202.589661751538,92.4668685231885,3.16087358735629));
#12515=CARTESIAN_POINT('Ctrl Pts',(-201.93404073716,94.2517775207246,3.25270978989014));
#12516=CARTESIAN_POINT('Ctrl Pts',(-201.927395875445,95.0027899210604,3.29157655282255));
#12517=CARTESIAN_POINT('Ctrl Pts',(-201.922621915119,95.001787031353,2.20842344717746));
#12518=CARTESIAN_POINT('Ctrl Pts',(-201.921899499162,95.1063092901838,2.2138544525384));
#12519=CARTESIAN_POINT('Ctrl Pts',(-201.974189435781,96.2295220789706,2.27225489750078));
#12520=CARTESIAN_POINT('Ctrl Pts',(-203.354320060973,98.2399546801978,2.3836247820646));
#12521=CARTESIAN_POINT('Ctrl Pts',(-206.832302471161,98.13819018824,2.54253310086891));
#12522=CARTESIAN_POINT('Ctrl Pts',(-208.630450654962,95.1593678146252,2.70144141967321));
#12523=CARTESIAN_POINT('Ctrl Pts',(-207.100242158396,92.0344389026441,2.86034973847752));
#12524=CARTESIAN_POINT('Ctrl Pts',(-203.644555171756,91.6283032143389,3.01925805728183));
#12525=CARTESIAN_POINT('Ctrl Pts',(-202.028743648494,93.5887151672915,3.13528262684847));
#12526=CARTESIAN_POINT('Ctrl Pts',(-201.923273182704,94.8028151314237,3.19833775681368));
#12527=CARTESIAN_POINT('Ctrl Pts',(-201.925054591669,94.9973187846012,3.20842344717746));
#12528=CARTESIAN_POINT('Origin',(-205.,95.,-2.20842344717744));
#12529=CARTESIAN_POINT('',(-201.930545984431,95.0016532623852,1.20842344717746));
#12530=CARTESIAN_POINT('',(-201.923792939525,94.9976530037673,1.29157655282255));
#12531=CARTESIAN_POINT('',(-201.9265,95.0000000000003,-2.20842344717744));
#12532=CARTESIAN_POINT('Ctrl Pts',(-201.923792939525,94.9976530037673,1.29157655282255));
#12533=CARTESIAN_POINT('Ctrl Pts',(-201.931146920561,95.8671823765141,1.33671262094101));
#12534=CARTESIAN_POINT('Ctrl Pts',(-202.771183541663,97.7695818819316,1.43481812866091));
#12535=CARTESIAN_POINT('Ctrl Pts',(-205.998843827582,98.4939765624303,1.58589307598225));
#12536=CARTESIAN_POINT('Ctrl Pts',(-208.478131313111,96.0526980537919,1.74480139478655));
#12537=CARTESIAN_POINT('Ctrl Pts',(-207.768707380001,92.6463153370295,1.90370971359086));
#12538=CARTESIAN_POINT('Ctrl Pts',(-204.520963226813,91.3977655726169,2.06261803239517));
#12539=CARTESIAN_POINT('Ctrl Pts',(-202.235891795972,93.0688641894186,2.19190697880573));
#12540=CARTESIAN_POINT('Ctrl Pts',(-201.929850794166,94.5464424883642,2.26822648561486));
#12541=CARTESIAN_POINT('Ctrl Pts',(-201.931144181024,94.9990189299375,2.29157655282255));
#12542=CARTESIAN_POINT('Ctrl Pts',(-201.930545984431,95.0016532623852,1.20842344717746));
#12543=CARTESIAN_POINT('Ctrl Pts',(-201.928558586322,95.4074704507228,1.22937114826312));
#12544=CARTESIAN_POINT('Ctrl Pts',(-202.192304342945,96.8369841963156,1.30328828895022));
#12545=CARTESIAN_POINT('Ctrl Pts',(-204.35839704753,98.5768482113765,1.43017486923876));
#12546=CARTESIAN_POINT('Ctrl Pts',(-207.659317996079,97.4766096293226,1.58908318804307));
#12547=CARTESIAN_POINT('Ctrl Pts',(-208.522221537982,94.105828029106,1.74799150684737));
#12548=CARTESIAN_POINT('Ctrl Pts',(-206.155984190728,91.5548205487187,1.90689982565168));
#12549=CARTESIAN_POINT('Ctrl Pts',(-202.847048345562,92.141549371385,2.06037713909504));
#12550=CARTESIAN_POINT('Ctrl Pts',(-201.928945334298,94.0868874505449,2.16088501293697));
#12551=CARTESIAN_POINT('Ctrl Pts',(-201.922621915119,95.001787031353,2.20842344717746));
#12552=CARTESIAN_POINT('Origin',(-205.,95.,-2.20842344717744));
#12553=CARTESIAN_POINT('',(-201.929615821727,94.9968993793473,0.208423447177457));
#12554=CARTESIAN_POINT('',(-201.923720806533,95.0022768293025,0.291576552822547));
#12555=CARTESIAN_POINT('',(-201.9265,95.0000000000003,-2.20842344717744));
#12556=CARTESIAN_POINT('',(-204.206200717467,92.0307770462543,0.));
#12557=CARTESIAN_POINT('Ctrl Pts',(-204.206200717467,92.0307770462543,-1.66533453693773E-15));
#12558=CARTESIAN_POINT('Ctrl Pts',(-203.217993421758,92.294966786987,0.0529694396014339));
#12559=CARTESIAN_POINT('Ctrl Pts',(-202.119889397913,93.3375904473839,0.12244392199392));
#12560=CARTESIAN_POINT('Ctrl Pts',(-201.927197935628,94.6776695912699,0.191918404386406));
#12561=CARTESIAN_POINT('Ctrl Pts',(-201.929615821727,94.9968993793473,0.208423447177457));
#12562=CARTESIAN_POINT('',(-205.795569479788,92.0254105888435,-2.77270672666423E-16));
#12563=CARTESIAN_POINT('Origin',(-205.,95.,0.));
#12564=CARTESIAN_POINT('Ctrl Pts',(-205.79557093555,92.025406175614,7.42000861794767E-16));
#12565=CARTESIAN_POINT('Ctrl Pts',(-204.831203783408,91.7689270056451,0.0519060689144966));
#12566=CARTESIAN_POINT('Ctrl Pts',(-202.766510651225,92.2462498650741,0.149098253188679));
#12567=CARTESIAN_POINT('Ctrl Pts',(-201.931001095851,94.1300845553796,0.246290437462861));
#12568=CARTESIAN_POINT('Ctrl Pts',(-201.923720806533,95.0022768293025,0.291576552822547));
#12569=CARTESIAN_POINT('Origin',(-205.,-95.,9.));
#12570=CARTESIAN_POINT('',(-202.486486965975,-94.9993627239001,16.612583302492));
#12571=CARTESIAN_POINT('',(-202.484598105996,-95.003732732209,16.887416697508));
#12572=CARTESIAN_POINT('',(-202.4825,-95.,9.));
#12573=CARTESIAN_POINT('',(-203.086534003335,-93.3640127966251,17.));
#12574=CARTESIAN_POINT('Ctrl Pts',(-202.484598105996,-95.003732732209,16.887416697508));
#12575=CARTESIAN_POINT('Ctrl Pts',(-202.489779960202,-94.411044798617,16.9249444650054));
#12576=CARTESIAN_POINT('Ctrl Pts',(-202.700778171916,-93.8151964396957,
16.9624722325027));
#12577=CARTESIAN_POINT('Ctrl Pts',(-203.086534003335,-93.3640127966251,
17.));
#12578=CARTESIAN_POINT('',(-202.4825,-95.,17.));
#12579=CARTESIAN_POINT('Origin',(-205.,-95.,17.));
#12580=CARTESIAN_POINT('',(-202.4825,-95.,18.));
#12581=CARTESIAN_POINT('',(-202.4825,-95.,9.));
#12582=CARTESIAN_POINT('Origin',(-205.,-95.,18.));
#12583=CARTESIAN_POINT('',(-206.91715084711,-93.3612115975349,17.));
#12584=CARTESIAN_POINT('Origin',(-205.,-95.,17.));
#12585=CARTESIAN_POINT('Ctrl Pts',(-206.917153877181,-93.3612092940951,
17.));
#12586=CARTESIAN_POINT('Ctrl Pts',(-206.38518496824,-92.7406416843865,16.9480939310855));
#12587=CARTESIAN_POINT('Ctrl Pts',(-205.522590942761,-92.4011122774809,
16.896187862171));
#12588=CARTESIAN_POINT('Ctrl Pts',(-204.710520941543,-92.4950342974083,
16.8442817932565));
#12589=CARTESIAN_POINT('Ctrl Pts',(-203.881814515085,-92.5908804453796,
16.7913123536551));
#12590=CARTESIAN_POINT('Ctrl Pts',(-203.10572343255,-93.1381196925948,16.7383429140536));
#12591=CARTESIAN_POINT('Ctrl Pts',(-202.737493126959,-93.8863932946479,
16.6853734744522));
#12592=CARTESIAN_POINT('Ctrl Pts',(-202.568820099224,-94.229150455359,16.6611100837988));
#12593=CARTESIAN_POINT('Ctrl Pts',(-202.48572547236,-94.614089163254,16.6368466931454));
#12594=CARTESIAN_POINT('Ctrl Pts',(-202.486486965975,-94.9993627239001,
16.612583302492));
#12595=CARTESIAN_POINT('Origin',(-205.,-95.,9.));
#12596=CARTESIAN_POINT('',(-202.482805352586,-95.0023102474081,15.612583302492));
#12597=CARTESIAN_POINT('',(-202.478253974141,-94.9999676034812,15.887416697508));
#12598=CARTESIAN_POINT('',(-202.4825,-95.,9.));
#12599=CARTESIAN_POINT('Ctrl Pts',(-202.478253974141,-94.9999676034812,
15.887416697508));
#12600=CARTESIAN_POINT('Ctrl Pts',(-202.478143102466,-94.1647321275155,
15.9404611607301));
#12601=CARTESIAN_POINT('Ctrl Pts',(-202.934422645956,-93.3296312577737,
15.9935056239521));
#12602=CARTESIAN_POINT('Ctrl Pts',(-203.637201829229,-92.8782275063029,
16.0465500871742));
#12603=CARTESIAN_POINT('Ctrl Pts',(-204.338987034326,-92.4274621992942,
16.0995195267756));
#12604=CARTESIAN_POINT('Ctrl Pts',(-205.28657426302,-92.3593094099306,16.152488966377));
#12605=CARTESIAN_POINT('Ctrl Pts',(-206.045561366399,-92.7051721137283,
16.2054584059785));
#12606=CARTESIAN_POINT('Ctrl Pts',(-206.804548469777,-93.051034817526,16.2584278455799));
#12607=CARTESIAN_POINT('Ctrl Pts',(-207.374935447839,-93.8109130144851,
16.3113972851814));
#12608=CARTESIAN_POINT('Ctrl Pts',(-207.495329357382,-94.6361476632023,
16.3643667247828));
#12609=CARTESIAN_POINT('Ctrl Pts',(-207.615723266924,-95.4613823119195,
16.4173361643842));
#12610=CARTESIAN_POINT('Ctrl Pts',(-207.286124107946,-96.3519734123947,
16.4703056039857));
#12611=CARTESIAN_POINT('Ctrl Pts',(-206.657476777652,-96.9003741267467,
16.5232750435871));
#12612=CARTESIAN_POINT('Ctrl Pts',(-206.028829447358,-97.4487748410986,
16.5762444831885));
#12613=CARTESIAN_POINT('Ctrl Pts',(-205.101133945748,-97.6549851693273,
16.62921392279));
#12614=CARTESIAN_POINT('Ctrl Pts',(-204.299947451515,-97.42304645291,16.6821833623914));
#12615=CARTESIAN_POINT('Ctrl Pts',(-203.498760957281,-97.1911077364927,
16.7351528019928));
#12616=CARTESIAN_POINT('Ctrl Pts',(-202.824083470424,-96.5210199754295,
16.7881222415943));
#12617=CARTESIAN_POINT('Ctrl Pts',(-202.584905723576,-95.7234546501587,
16.8410916811957));
#12618=CARTESIAN_POINT('Ctrl Pts',(-202.515180531668,-95.4909480892605,
16.8565333532998));
#12619=CARTESIAN_POINT('Ctrl Pts',(-202.482465911653,-95.2476079569009,
16.8719750254039));
#12620=CARTESIAN_POINT('Ctrl Pts',(-202.484598105996,-95.003732732209,16.887416697508));
#12621=CARTESIAN_POINT('Ctrl Pts',(-202.486486965975,-94.9993627239001,
16.612583302492));
#12622=CARTESIAN_POINT('Ctrl Pts',(-202.487387890058,-95.4551803731427,
16.5838772535439));
#12623=CARTESIAN_POINT('Ctrl Pts',(-202.605664630852,-95.9114667253842,
16.5551712045959));
#12624=CARTESIAN_POINT('Ctrl Pts',(-202.83846505618,-96.2989227836093,16.5264651556479));
#12625=CARTESIAN_POINT('Ctrl Pts',(-203.268036819641,-97.0138707136265,
16.4734957160464));
#12626=CARTESIAN_POINT('Ctrl Pts',(-204.087549875211,-97.4944586167699,
16.420526276445));
#12627=CARTESIAN_POINT('Ctrl Pts',(-204.921224617056,-97.5205023202695,
16.3675568368436));
#12628=CARTESIAN_POINT('Ctrl Pts',(-205.7548993589,-97.5465460237691,16.3145873972421));
#12629=CARTESIAN_POINT('Ctrl Pts',(-206.602735787018,-97.1180455276249,
16.2616179576407));
#12630=CARTESIAN_POINT('Ctrl Pts',(-207.076148172397,-96.4313676243484,
16.2086485180393));
#12631=CARTESIAN_POINT('Ctrl Pts',(-207.549560557776,-95.7446897210719,
16.1556790784378));
#12632=CARTESIAN_POINT('Ctrl Pts',(-207.648548900416,-94.7998344106631,
16.1027096388364));
#12633=CARTESIAN_POINT('Ctrl Pts',(-207.327709564386,-94.0299449024905,
16.049740199235));
#12634=CARTESIAN_POINT('Ctrl Pts',(-207.006870228356,-93.2600553943178,
15.9967707596335));
#12635=CARTESIAN_POINT('Ctrl Pts',(-206.266203213656,-92.6651316883815,
15.9438013200321));
#12636=CARTESIAN_POINT('Ctrl Pts',(-205.445239651077,-92.5178705169809,
15.8908318804307));
#12637=CARTESIAN_POINT('Ctrl Pts',(-204.624276088498,-92.3706093455804,
15.8378624408292));
#12638=CARTESIAN_POINT('Ctrl Pts',(-203.723015978041,-92.6710107087159,
15.7848930012278));
#12639=CARTESIAN_POINT('Ctrl Pts',(-203.154585383115,-93.2813785734586,
15.7319235616263));
#12640=CARTESIAN_POINT('Ctrl Pts',(-202.72769360672,-93.7397652689682,15.6921434752482));
#12641=CARTESIAN_POINT('Ctrl Pts',(-202.48851836135,-94.3729737086458,15.6523633888701));
#12642=CARTESIAN_POINT('Ctrl Pts',(-202.482805352586,-95.0023102474081,
15.612583302492));
#12643=CARTESIAN_POINT('Origin',(-205.,-95.,9.));
#12644=CARTESIAN_POINT('',(-202.478471589337,-94.9993246203416,14.612583302492));
#12645=CARTESIAN_POINT('',(-202.483904335665,-94.997810483196,14.887416697508));
#12646=CARTESIAN_POINT('',(-202.4825,-95.,9.));
#12647=CARTESIAN_POINT('Ctrl Pts',(-202.483904335665,-94.997810483196,14.887416697508));
#12648=CARTESIAN_POINT('Ctrl Pts',(-202.481855015029,-94.7508698395785,
14.9030084168534));
#12649=CARTESIAN_POINT('Ctrl Pts',(-202.515258260586,-94.5044716173505,
14.9186001361987));
#12650=CARTESIAN_POINT('Ctrl Pts',(-202.586378537099,-94.2694889359093,
14.934191855544));
#12651=CARTESIAN_POINT('Ctrl Pts',(-202.82799404516,-93.4711869221089,14.9871612951455));
#12652=CARTESIAN_POINT('Ctrl Pts',(-203.504921150218,-92.804637518854,15.0401307347469));
#12653=CARTESIAN_POINT('Ctrl Pts',(-204.30686045751,-92.5753822437128,15.0931001743483));
#12654=CARTESIAN_POINT('Ctrl Pts',(-205.108799764801,-92.3461269685716,
15.1460696139498));
#12655=CARTESIAN_POINT('Ctrl Pts',(-206.035751274325,-92.5541658215442,
15.1990390535512));
#12656=CARTESIAN_POINT('Ctrl Pts',(-206.662805165788,-93.1041370306651,
15.2520084931526));
#12657=CARTESIAN_POINT('Ctrl Pts',(-207.289859057251,-93.6541082397861,
15.3049779327541));
#12658=CARTESIAN_POINT('Ctrl Pts',(-207.617015330653,-94.5460118050555,
15.3579473723555));
#12659=CARTESIAN_POINT('Ctrl Pts',(-207.494308264464,-95.3709998251231,
15.410916811957));
#12660=CARTESIAN_POINT('Ctrl Pts',(-207.371601198275,-96.1959878451908,
15.4638862515584));
#12661=CARTESIAN_POINT('Ctrl Pts',(-206.799030792495,-96.9540603200567,
15.5168556911598));
#12662=CARTESIAN_POINT('Ctrl Pts',(-206.03905828976,-97.2977299359365,15.5698251307613));
#12663=CARTESIAN_POINT('Ctrl Pts',(-205.279085787025,-97.6413995518163,
15.6227945703627));
#12664=CARTESIAN_POINT('Ctrl Pts',(-204.331711187336,-97.57066630871,15.6757640099641));
#12665=CARTESIAN_POINT('Ctrl Pts',(-203.631209499739,-97.1179355866594,
15.7287334495656));
#12666=CARTESIAN_POINT('Ctrl Pts',(-202.9316999724,-96.6658460927997,15.7816278655464));
#12667=CARTESIAN_POINT('Ctrl Pts',(-202.478364532193,-95.8328404430598,
15.8345222815272));
#12668=CARTESIAN_POINT('Ctrl Pts',(-202.478253974141,-94.9999676034812,
15.887416697508));
#12669=CARTESIAN_POINT('Ctrl Pts',(-202.482805352586,-95.0023102474081,
15.612583302492));
#12670=CARTESIAN_POINT('Ctrl Pts',(-202.480911166388,-95.2109709784878,
15.5993939492687));
#12671=CARTESIAN_POINT('Ctrl Pts',(-202.504681444081,-95.4192060721596,
15.5862045960454));
#12672=CARTESIAN_POINT('Ctrl Pts',(-202.555783523722,-95.6205025079985,
15.573015242822));
#12673=CARTESIAN_POINT('Ctrl Pts',(-202.761013338649,-96.4289242114456,
15.5200458032206));
#12674=CARTESIAN_POINT('Ctrl Pts',(-203.407074047896,-97.1254332519901,
15.4670763636192));
#12675=CARTESIAN_POINT('Ctrl Pts',(-204.197813504076,-97.3907552453631,
15.4141069240177));
#12676=CARTESIAN_POINT('Ctrl Pts',(-204.988552960257,-97.6560772387361,
15.3611374844163));
#12677=CARTESIAN_POINT('Ctrl Pts',(-205.923971163369,-97.4902121849378,
15.3081680448149));
#12678=CARTESIAN_POINT('Ctrl Pts',(-206.575278375994,-96.9691909878947,
15.2551986052134));
#12679=CARTESIAN_POINT('Ctrl Pts',(-207.226585588618,-96.4481697908517,
15.202229165612));
#12680=CARTESIAN_POINT('Ctrl Pts',(-207.593781810755,-95.5719924505639,
15.1492597260106));
#12681=CARTESIAN_POINT('Ctrl Pts',(-207.508545988586,-94.7422941067118,
15.0962902864091));
#12682=CARTESIAN_POINT('Ctrl Pts',(-207.423310166418,-93.9125957628597,
15.0433208468077));
#12683=CARTESIAN_POINT('Ctrl Pts',(-206.885642299945,-93.1293764154432,
14.9903514072062));
#12684=CARTESIAN_POINT('Ctrl Pts',(-206.142006507432,-92.7516592703233,
14.9373819676048));
#12685=CARTESIAN_POINT('Ctrl Pts',(-205.398370714919,-92.3739421252033,
14.8844125280034));
#12686=CARTESIAN_POINT('Ctrl Pts',(-204.448766996366,-92.40172718238,14.8314430884019));
#12687=CARTESIAN_POINT('Ctrl Pts',(-203.728488305932,-92.8222780072335,
14.7784736488005));
#12688=CARTESIAN_POINT('Ctrl Pts',(-203.008209615498,-93.2428288320871,
14.7255042091991));
#12689=CARTESIAN_POINT('Ctrl Pts',(-202.517255953184,-94.0561454246176,
14.6725347695976));
#12690=CARTESIAN_POINT('Ctrl Pts',(-202.480677774616,-94.8894079650979,
14.6195653299962));
#12691=CARTESIAN_POINT('Ctrl Pts',(-202.479070622449,-94.9260194025585,
14.6172379874948));
#12692=CARTESIAN_POINT('Ctrl Pts',(-202.478340642232,-94.9626693456751,
14.6149106449934));
#12693=CARTESIAN_POINT('Ctrl Pts',(-202.478471589337,-94.9993246203416,
14.612583302492));
#12694=CARTESIAN_POINT('Origin',(-205.,-95.,9.));
#12695=CARTESIAN_POINT('',(-202.484820254705,-94.9980759215734,13.612583302492));
#12696=CARTESIAN_POINT('',(-202.486027831966,-95.0011568597348,13.887416697508));
#12697=CARTESIAN_POINT('',(-202.4825,-95.,9.));
#12698=CARTESIAN_POINT('Ctrl Pts',(-202.486027831966,-95.0011568597348,
13.887416697508));
#12699=CARTESIAN_POINT('Ctrl Pts',(-202.488072607706,-94.5074163488195,
13.9185251125781));
#12700=CARTESIAN_POINT('Ctrl Pts',(-202.628459862778,-94.012602672555,13.9496335276481));
#12701=CARTESIAN_POINT('Ctrl Pts',(-202.899511290069,-93.6045924957187,
13.9807419427182));
#12702=CARTESIAN_POINT('Ctrl Pts',(-203.361040499271,-92.9098585991177,
14.0337113823196));
#12703=CARTESIAN_POINT('Ctrl Pts',(-204.201405940211,-92.4667951494829,
14.0866808219211));
#12704=CARTESIAN_POINT('Ctrl Pts',(-205.035388793712,-92.4784999432582,
14.1396502615225));
#12705=CARTESIAN_POINT('Ctrl Pts',(-205.869371647213,-92.4902047370334,
14.1926197011239));
#12706=CARTESIAN_POINT('Ctrl Pts',(-206.696971913274,-92.9566777742187,
14.2455891407254));
#12707=CARTESIAN_POINT('Ctrl Pts',(-207.138822249404,-93.6640904479811,
14.2985585803268));
#12708=CARTESIAN_POINT('Ctrl Pts',(-207.580672585535,-94.3715031217434,
14.3515280199282));
#12709=CARTESIAN_POINT('Ctrl Pts',(-207.636772991736,-95.3198554320829,
14.4044974595297));
#12710=CARTESIAN_POINT('Ctrl Pts',(-207.281407366659,-96.0744279247623,
14.4574668991311));
#12711=CARTESIAN_POINT('Ctrl Pts',(-206.926041741582,-96.8290004174418,
14.5104363387325));
#12712=CARTESIAN_POINT('Ctrl Pts',(-206.159210085227,-97.3897930924613,
14.563405778334));
#12713=CARTESIAN_POINT('Ctrl Pts',(-205.332423720056,-97.4997418351244,
14.6163752179354));
#12714=CARTESIAN_POINT('Ctrl Pts',(-204.505637354885,-97.6096905777875,
14.6693446575369));
#12715=CARTESIAN_POINT('Ctrl Pts',(-203.618896280897,-97.2687953880943,
14.7223140971383));
#12716=CARTESIAN_POINT('Ctrl Pts',(-203.078677699436,-96.6333204810748,
14.7752835367397));
#12717=CARTESIAN_POINT('Ctrl Pts',(-202.697474138156,-96.1848995900276,
14.8126612569958));
#12718=CARTESIAN_POINT('Ctrl Pts',(-202.488817131473,-95.5897964016549,
14.8500389772519));
#12719=CARTESIAN_POINT('Ctrl Pts',(-202.483904335665,-94.997810483196,14.887416697508));
#12720=CARTESIAN_POINT('Ctrl Pts',(-202.478471589337,-94.9993246203416,
14.612583302492));
#12721=CARTESIAN_POINT('Ctrl Pts',(-202.481320949066,-95.7969296044664,
14.5619412053919));
#12722=CARTESIAN_POINT('Ctrl Pts',(-202.891803231304,-96.5970589773882,
14.5112991082919));
#12723=CARTESIAN_POINT('Ctrl Pts',(-203.5425537207,-97.0579274461484,14.4606570111919));
#12724=CARTESIAN_POINT('Ctrl Pts',(-204.223210540176,-97.5399758982885,
14.4076875715905));
#12725=CARTESIAN_POINT('Ctrl Pts',(-205.166726873948,-97.6508643141388,
14.354718131989));
#12726=CARTESIAN_POINT('Ctrl Pts',(-205.940600116827,-97.339762054474,14.3017486923876));
#12727=CARTESIAN_POINT('Ctrl Pts',(-206.714473359706,-97.0286597948092,
14.2487792527862));
#12728=CARTESIAN_POINT('Ctrl Pts',(-207.318703511691,-96.2955668596293,
14.1958098131847));
#12729=CARTESIAN_POINT('Ctrl Pts',(-207.476314843211,-95.4765289580023,
14.1428403735833));
#12730=CARTESIAN_POINT('Ctrl Pts',(-207.633926174731,-94.6574910563753,
14.0898709339818));
#12731=CARTESIAN_POINT('Ctrl Pts',(-207.344918685787,-93.7525081883012,
14.0369014943804));
#12732=CARTESIAN_POINT('Ctrl Pts',(-206.741771796435,-93.1764194409759,
13.983932054779));
#12733=CARTESIAN_POINT('Ctrl Pts',(-206.138624907084,-92.6003306936505,
13.9309626151775));
#12734=CARTESIAN_POINT('Ctrl Pts',(-205.221338617327,-92.353136067074,13.8779931755761));
#12735=CARTESIAN_POINT('Ctrl Pts',(-204.410391835157,-92.5481481976757,
13.8250237359747));
#12736=CARTESIAN_POINT('Ctrl Pts',(-203.599445052987,-92.7431603282774,
13.7720542963732));
#12737=CARTESIAN_POINT('Ctrl Pts',(-202.894837778405,-93.3803792160573,
13.7190848567718));
#12738=CARTESIAN_POINT('Ctrl Pts',(-202.619558048972,-94.1677072833915,
13.6661154171704));
#12739=CARTESIAN_POINT('Ctrl Pts',(-202.526823407038,-94.4329378056649,
13.6482713789442));
#12740=CARTESIAN_POINT('Ctrl Pts',(-202.482810673008,-94.7152033533037,
13.6304273407181));
#12741=CARTESIAN_POINT('Ctrl Pts',(-202.484820254705,-94.9980759215734,
13.612583302492));
#12742=CARTESIAN_POINT('Origin',(-205.,-95.,9.));
#12743=CARTESIAN_POINT('',(-202.485427278837,-95.0016272057563,12.612583302492));
#12744=CARTESIAN_POINT('',(-202.479664234459,-95.0016558831106,12.887416697508));
#12745=CARTESIAN_POINT('',(-202.4825,-95.,9.));
#12746=CARTESIAN_POINT('Ctrl Pts',(-202.479664234459,-95.0016558831106,
12.887416697508));
#12747=CARTESIAN_POINT('Ctrl Pts',(-202.48525308669,-94.2663994936904,12.9340418083028));
#12748=CARTESIAN_POINT('Ctrl Pts',(-202.825737534307,-93.526637293353,12.9806669190976));
#12749=CARTESIAN_POINT('Ctrl Pts',(-203.391055573645,-93.0582191799,13.0272920298924));
#12750=CARTESIAN_POINT('Ctrl Pts',(-204.033297044601,-92.5260629116183,
13.0802614694938));
#12751=CARTESIAN_POINT('Ctrl Pts',(-204.965721672596,-92.3441189188828,
13.1332309090952));
#12752=CARTESIAN_POINT('Ctrl Pts',(-205.76091121895,-92.5957893110237,13.1862003486967));
#12753=CARTESIAN_POINT('Ctrl Pts',(-206.556100765303,-92.8474597031646,
13.2391697882981));
#12754=CARTESIAN_POINT('Ctrl Pts',(-207.214055230015,-93.5327444801819,
13.2921392278995));
#12755=CARTESIAN_POINT('Ctrl Pts',(-207.433171963302,-94.3375129302743,
13.345108667501));
#12756=CARTESIAN_POINT('Ctrl Pts',(-207.652288696588,-95.1422813803668,
13.3980781071024));
#12757=CARTESIAN_POINT('Ctrl Pts',(-207.43256769845,-96.0665335035343,13.4510475467038));
#12758=CARTESIAN_POINT('Ctrl Pts',(-206.87472784669,-96.6865972909008,13.5040169863053));
#12759=CARTESIAN_POINT('Ctrl Pts',(-206.31688799493,-97.3066610782673,13.5569864259067));
#12760=CARTESIAN_POINT('Ctrl Pts',(-205.420929289549,-97.6225365298328,
13.6099558655081));
#12761=CARTESIAN_POINT('Ctrl Pts',(-204.59755419382,-97.4894281052916,13.6629253051096));
#12762=CARTESIAN_POINT('Ctrl Pts',(-203.774179098092,-97.3563196807503,
13.715894744711));
#12763=CARTESIAN_POINT('Ctrl Pts',(-203.023387612016,-96.7742273801023,
13.7688641843124));
#12764=CARTESIAN_POINT('Ctrl Pts',(-202.689338357709,-96.0099790579946,
13.8218336239139));
#12765=CARTESIAN_POINT('Ctrl Pts',(-202.551472845104,-95.6945660303437,
13.8436946484453));
#12766=CARTESIAN_POINT('Ctrl Pts',(-202.484590893038,-95.3481264304106,
13.8655556729767));
#12767=CARTESIAN_POINT('Ctrl Pts',(-202.486027831966,-95.0011568597348,
13.887416697508));
#12768=CARTESIAN_POINT('Ctrl Pts',(-202.484820254705,-94.9980759215734,
13.612583302492));
#12769=CARTESIAN_POINT('Ctrl Pts',(-202.48877605007,-95.5549012529596,13.5774579011167));
#12770=CARTESIAN_POINT('Ctrl Pts',(-202.671061992949,-96.1140787058531,
13.5423324997413));
#12771=CARTESIAN_POINT('Ctrl Pts',(-203.011086838027,-96.5503030290954,
13.507207098366));
#12772=CARTESIAN_POINT('Ctrl Pts',(-203.523847540798,-97.2081334605764,
13.4542376587646));
#12773=CARTESIAN_POINT('Ctrl Pts',(-204.395321130623,-97.5863570766498,
13.4012682191632));
#12774=CARTESIAN_POINT('Ctrl Pts',(-205.226028984189,-97.5115982852547,
13.3482987795617));
#12775=CARTESIAN_POINT('Ctrl Pts',(-206.056736837754,-97.4368394938597,
13.2953293399603));
#12776=CARTESIAN_POINT('Ctrl Pts',(-206.846678955059,-96.9090982949961,
13.2423599003589));
#12777=CARTESIAN_POINT('Ctrl Pts',(-207.233750283983,-96.1702883050523,
13.1893904607574));
#12778=CARTESIAN_POINT('Ctrl Pts',(-207.620821612906,-95.4314783151084,
13.136421021156));
#12779=CARTESIAN_POINT('Ctrl Pts',(-207.605022153448,-94.4815995340844,
13.0834515815546));
#12780=CARTESIAN_POINT('Ctrl Pts',(-207.193594289559,-93.7560710868749,
13.0304821419531));
#12781=CARTESIAN_POINT('Ctrl Pts',(-206.782166425669,-93.0305426396654,
12.9775127023517));
#12782=CARTESIAN_POINT('Ctrl Pts',(-205.975110157349,-92.5293645262705,
12.9245432627503));
#12783=CARTESIAN_POINT('Ctrl Pts',(-205.14237556783,-92.4822739931015,12.8715738231488));
#12784=CARTESIAN_POINT('Ctrl Pts',(-204.309640978312,-92.4351834599324,
12.8186043835474));
#12785=CARTESIAN_POINT('Ctrl Pts',(-203.451228067597,-92.8421805069893,
12.765634943946));
#12786=CARTESIAN_POINT('Ctrl Pts',(-202.960628516811,-93.5166999623558,
12.7126655043445));
#12787=CARTESIAN_POINT('Ctrl Pts',(-202.651643539561,-93.9415197124696,
12.6793047703937));
#12788=CARTESIAN_POINT('Ctrl Pts',(-202.488556091416,-94.4724553969259,
12.6459440364428));
#12789=CARTESIAN_POINT('Ctrl Pts',(-202.485427278837,-95.0016272057563,
12.612583302492));
#12790=CARTESIAN_POINT('Origin',(-205.,-95.,9.));
#12791=CARTESIAN_POINT('',(-202.478890786754,-95.001146280366,11.612583302492));
#12792=CARTESIAN_POINT('',(-202.480886591773,-94.9978964058402,11.887416697508));
#12793=CARTESIAN_POINT('',(-202.4825,-95.,9.));
#12794=CARTESIAN_POINT('Ctrl Pts',(-202.480886591773,-94.9978964058402,
11.887416697508));
#12795=CARTESIAN_POINT('Ctrl Pts',(-202.479589394008,-94.853069705361,11.8965890644261));
#12796=CARTESIAN_POINT('Ctrl Pts',(-202.491001823839,-94.7084473374192,
11.9057614313441));
#12797=CARTESIAN_POINT('Ctrl Pts',(-202.515848746476,-94.5661711513124,
11.9149337982622));
#12798=CARTESIAN_POINT('Ctrl Pts',(-202.659337071752,-93.7445413676335,
11.9679032378636));
#12799=CARTESIAN_POINT('Ctrl Pts',(-203.250857561182,-93.001155321196,12.0208726774651));
#12800=CARTESIAN_POINT('Ctrl Pts',(-204.019260528061,-92.6767770213518,
12.0738421170665));
#12801=CARTESIAN_POINT('Ctrl Pts',(-204.78766349494,-92.3523987215075,12.1268115566679));
#12802=CARTESIAN_POINT('Ctrl Pts',(-205.732948939268,-92.4470281682566,
12.1797809962694));
#12803=CARTESIAN_POINT('Ctrl Pts',(-206.421803295997,-92.9172877520339,
12.2327504358708));
#12804=CARTESIAN_POINT('Ctrl Pts',(-207.110657652725,-93.3875473358113,
12.2857198754723));
#12805=CARTESIAN_POINT('Ctrl Pts',(-207.543080921853,-94.2334370566169,
12.3386893150737));
#12806=CARTESIAN_POINT('Ctrl Pts',(-207.520852693365,-95.0672057936051,
12.3916587546751));
#12807=CARTESIAN_POINT('Ctrl Pts',(-207.498624464876,-95.9009745305933,
12.4446281942766));
#12808=CARTESIAN_POINT('Ctrl Pts',(-207.021744738771,-96.7226222837642,
12.497597633878));
#12809=CARTESIAN_POINT('Ctrl Pts',(-206.308812516505,-97.1555103147487,
12.5505670734794));
#12810=CARTESIAN_POINT('Ctrl Pts',(-205.595880294238,-97.5883983457332,
12.6035365130809));
#12811=CARTESIAN_POINT('Ctrl Pts',(-204.64689557581,-97.6325266545312,12.6565059526823));
#12812=CARTESIAN_POINT('Ctrl Pts',(-203.896867652842,-97.267667071015,12.7094753922837));
#12813=CARTESIAN_POINT('Ctrl Pts',(-203.146839729873,-96.9028074874987,
12.7624448318852));
#12814=CARTESIAN_POINT('Ctrl Pts',(-202.595768602363,-96.1289600116682,
12.8154142714866));
#12815=CARTESIAN_POINT('Ctrl Pts',(-202.496262195567,-95.3008520018389,
12.868383711088));
#12816=CARTESIAN_POINT('Ctrl Pts',(-202.484343976915,-95.2016667066702,
12.8747280398947));
#12817=CARTESIAN_POINT('Ctrl Pts',(-202.478903753345,-95.1017030081934,
12.8810723687014));
#12818=CARTESIAN_POINT('Ctrl Pts',(-202.479664234459,-95.0016558831106,
12.887416697508));
#12819=CARTESIAN_POINT('Ctrl Pts',(-202.485427278837,-95.0016272057563,
12.612583302492));
#12820=CARTESIAN_POINT('Ctrl Pts',(-202.483588231621,-95.3126627559102,
12.5929745968414));
#12821=CARTESIAN_POINT('Ctrl Pts',(-202.537012171023,-95.6230889170507,
12.5733658911908));
#12822=CARTESIAN_POINT('Ctrl Pts',(-202.648554447949,-95.9109988275815,
12.5537571855402));
#12823=CARTESIAN_POINT('Ctrl Pts',(-202.949866120729,-96.6887363737646,
12.5007877459388));
#12824=CARTESIAN_POINT('Ctrl Pts',(-203.675275657147,-97.302169602455,12.4478183063373));
#12825=CARTESIAN_POINT('Ctrl Pts',(-204.492259379585,-97.4701041497275,
12.3948488667359));
#12826=CARTESIAN_POINT('Ctrl Pts',(-205.309243102023,-97.638038697,12.3418794271345));
#12827=CARTESIAN_POINT('Ctrl Pts',(-206.217801010483,-97.3604745628546,
12.288909987533));
#12828=CARTESIAN_POINT('Ctrl Pts',(-206.801455237106,-96.764645595246,12.2359405479316));
#12829=CARTESIAN_POINT('Ctrl Pts',(-207.38510946373,-96.1688166276373,12.1829711083302));
#12830=CARTESIAN_POINT('Ctrl Pts',(-207.643860008518,-95.2547228265654,
12.1300016687287));
#12831=CARTESIAN_POINT('Ctrl Pts',(-207.459097067741,-94.4413796821223,
12.0770322291273));
#12832=CARTESIAN_POINT('Ctrl Pts',(-207.274334126964,-93.6280365376793,
12.0240627895259));
#12833=CARTESIAN_POINT('Ctrl Pts',(-206.646057700621,-92.9154440498653,
11.9710933499244));
#12834=CARTESIAN_POINT('Ctrl Pts',(-205.86226619149,-92.6302506328449,11.918123910323));
#12835=CARTESIAN_POINT('Ctrl Pts',(-205.07847468236,-92.3450572158246,11.8651544707215));
#12836=CARTESIAN_POINT('Ctrl Pts',(-204.139168090441,-92.4872628695979,
11.8121850311201));
#12837=CARTESIAN_POINT('Ctrl Pts',(-203.474919308252,-92.9916813171766,
11.7592155915187));
#12838=CARTESIAN_POINT('Ctrl Pts',(-202.861985258302,-93.457132290117,11.7103381618431));
#12839=CARTESIAN_POINT('Ctrl Pts',(-202.483252854292,-94.2309941842871,
11.6614607321675));
#12840=CARTESIAN_POINT('Ctrl Pts',(-202.478890786754,-95.001146280366,11.612583302492));
#12841=CARTESIAN_POINT('Origin',(-205.,-95.,9.));
#12842=CARTESIAN_POINT('',(-202.481958443618,-94.9977164072965,10.612583302492));
#12843=CARTESIAN_POINT('',(-202.486464107889,-94.9995333136293,10.887416697508));
#12844=CARTESIAN_POINT('',(-202.4825,-95.,9.));
#12845=CARTESIAN_POINT('Ctrl Pts',(-202.486464107889,-94.9995333136293,
10.887416697508));
#12846=CARTESIAN_POINT('Ctrl Pts',(-202.485815886657,-94.6075083595682,
10.9121057601508));
#12847=CARTESIAN_POINT('Ctrl Pts',(-202.571975216773,-94.2157531015706,
10.9367948227936));
#12848=CARTESIAN_POINT('Ctrl Pts',(-202.746434366323,-93.8683388956723,
10.9614838854364));
#12849=CARTESIAN_POINT('Ctrl Pts',(-203.12072979903,-93.1229750046945,11.0144533250378));
#12850=CARTESIAN_POINT('Ctrl Pts',(-203.901469841937,-92.5817132483756,
11.0674227646392));
#12851=CARTESIAN_POINT('Ctrl Pts',(-204.730767622461,-92.4926649910269,
11.1203922042407));
#12852=CARTESIAN_POINT('Ctrl Pts',(-205.560065402984,-92.4036167336781,
11.1733616438421));
#12853=CARTESIAN_POINT('Ctrl Pts',(-206.437920921125,-92.7667819752994,
11.2263310834435));
#12854=CARTESIAN_POINT('Ctrl Pts',(-206.961930113172,-93.415687798643,11.279300523045));
#12855=CARTESIAN_POINT('Ctrl Pts',(-207.485939305218,-94.0645936219866,
11.3322699626464));
#12856=CARTESIAN_POINT('Ctrl Pts',(-207.656102171171,-94.9992400270525,
11.3852394022478));
#12857=CARTESIAN_POINT('Ctrl Pts',(-207.394417004214,-95.7911903249334,
11.4382088418493));
#12858=CARTESIAN_POINT('Ctrl Pts',(-207.132731837258,-96.5831406228142,
11.4911782814507));
#12859=CARTESIAN_POINT('Ctrl Pts',(-206.439198637392,-97.2323948135099,
11.5441477210522));
#12860=CARTESIAN_POINT('Ctrl Pts',(-205.631729147697,-97.4413384042955,
11.5971171606536));
#12861=CARTESIAN_POINT('Ctrl Pts',(-204.824259658002,-97.650281995081,11.650086600255));
#12862=CARTESIAN_POINT('Ctrl Pts',(-203.902853878478,-97.4189149859564,
11.7030560398565));
#12863=CARTESIAN_POINT('Ctrl Pts',(-203.289879069277,-96.853294720934,11.7560254794579));
#12864=CARTESIAN_POINT('Ctrl Pts',(-202.783049046652,-96.3856191698091,
11.7998225521413));
#12865=CARTESIAN_POINT('Ctrl Pts',(-202.487080572597,-95.6894284372179,
11.8436196248246));
#12866=CARTESIAN_POINT('Ctrl Pts',(-202.480886591773,-94.9978964058402,
11.887416697508));
#12867=CARTESIAN_POINT('Ctrl Pts',(-202.478890786754,-95.001146280366,11.612583302492));
#12868=CARTESIAN_POINT('Ctrl Pts',(-202.478525595217,-95.0656232801284,
11.6084912925661));
#12869=CARTESIAN_POINT('Ctrl Pts',(-202.480784368861,-95.1300742778814,
11.6043992826402));
#12870=CARTESIAN_POINT('Ctrl Pts',(-202.485749357697,-95.1943161233581,
11.6003072727144));
#12871=CARTESIAN_POINT('Ctrl Pts',(-202.550019161789,-96.0259012405764,
11.5473378331129));
#12872=CARTESIAN_POINT('Ctrl Pts',(-203.067749742433,-96.8224402336289,
11.4943683935115));
#12873=CARTESIAN_POINT('Ctrl Pts',(-203.801616294745,-97.218804079476,11.4413989539101));
#12874=CARTESIAN_POINT('Ctrl Pts',(-204.535482847057,-97.615167925323,11.3884295143086));
#12875=CARTESIAN_POINT('Ctrl Pts',(-205.485485371038,-97.6113566239648,
11.3354600747072));
#12876=CARTESIAN_POINT('Ctrl Pts',(-206.216148018684,-97.2091172546447,
11.2824906351058));
#12877=CARTESIAN_POINT('Ctrl Pts',(-206.946810666331,-96.8068778853247,
11.2295211955043));
#12878=CARTESIAN_POINT('Ctrl Pts',(-207.458133437644,-96.0062104480429,
11.1765517559029));
#12879=CARTESIAN_POINT('Ctrl Pts',(-207.515728831729,-95.1741364216021,
11.1235823163015));
#12880=CARTESIAN_POINT('Ctrl Pts',(-207.573324225813,-94.3420623951613,
11.0706128767));
#12881=CARTESIAN_POINT('Ctrl Pts',(-207.177192242668,-93.4785817795614,
11.0176434370986));
#12882=CARTESIAN_POINT('Ctrl Pts',(-206.508917569625,-92.9795092635214,
10.9646739974971));
#12883=CARTESIAN_POINT('Ctrl Pts',(-205.840642896582,-92.4804367474813,
10.9117045578957));
#12884=CARTESIAN_POINT('Ctrl Pts',(-204.900225533641,-92.3457723310011,
10.8587351182943));
#12885=CARTESIAN_POINT('Ctrl Pts',(-204.118747544549,-92.6372454300371,
10.8057656786928));
#12886=CARTESIAN_POINT('Ctrl Pts',(-203.337269555457,-92.9287185290731,
10.7527962390914));
#12887=CARTESIAN_POINT('Ctrl Pts',(-202.714730940213,-93.6463291436252,
10.69982679949));
#12888=CARTESIAN_POINT('Ctrl Pts',(-202.536499921054,-94.4611285782756,
10.6468573598885));
#12889=CARTESIAN_POINT('Ctrl Pts',(-202.498058257166,-94.6368681669895,
10.6354326740897));
#12890=CARTESIAN_POINT('Ctrl Pts',(-202.480285690666,-94.8171289594943,
10.6240079882908));
#12891=CARTESIAN_POINT('Ctrl Pts',(-202.481958443618,-94.9977164072965,
10.612583302492));
#12892=CARTESIAN_POINT('Origin',(-205.,-95.,9.));
#12893=CARTESIAN_POINT('',(-202.486537790415,-95.0001194277165,9.61258330249196));
#12894=CARTESIAN_POINT('',(-202.482602555105,-95.0023130495141,9.88741669750803));
#12895=CARTESIAN_POINT('',(-202.4825,-95.,9.));
#12896=CARTESIAN_POINT('Ctrl Pts',(-202.482602555105,-95.0023130495141,
9.88741669750803));
#12897=CARTESIAN_POINT('Ctrl Pts',(-202.488423652239,-94.3663734982534,
9.92762245587553));
#12898=CARTESIAN_POINT('Ctrl Pts',(-202.733269661135,-93.7264433715794,
9.96782821424302));
#12899=CARTESIAN_POINT('Ctrl Pts',(-203.168433552404,-93.2666277755833,
10.0080339726105));
#12900=CARTESIAN_POINT('Ctrl Pts',(-203.741744152458,-92.66083956442,10.061003412212));
#12901=CARTESIAN_POINT('Ctrl Pts',(-204.645389178865,-92.3676758393408,
10.1139728518134));
#12902=CARTESIAN_POINT('Ctrl Pts',(-205.465142801446,-92.5215212136069,
10.1669422914148));
#12903=CARTESIAN_POINT('Ctrl Pts',(-206.284896424028,-92.675366587873,10.2199117310163));
#12904=CARTESIAN_POINT('Ctrl Pts',(-207.020758642784,-93.2762210614844,
10.2728811706177));
#12905=CARTESIAN_POINT('Ctrl Pts',(-207.335414328927,-94.0486563015507,
10.3258506102191));
#12906=CARTESIAN_POINT('Ctrl Pts',(-207.65007001507,-94.821091541617,10.3788200498206));
#12907=CARTESIAN_POINT('Ctrl Pts',(-207.543519168601,-95.7651075481382,
10.431789489422));
#12908=CARTESIAN_POINT('Ctrl Pts',(-207.064604102091,-96.4479726592609,
10.4847589290234));
#12909=CARTESIAN_POINT('Ctrl Pts',(-206.585689035581,-97.1308377703837,
10.5377283686249));
#12910=CARTESIAN_POINT('Ctrl Pts',(-205.734409749032,-97.5525519861079,
10.5906978082263));
#12911=CARTESIAN_POINT('Ctrl Pts',(-204.900987910111,-97.5198038666518,
10.6436672478277));
#12912=CARTESIAN_POINT('Ctrl Pts',(-204.06756607119,-97.4870557471958,10.6966366874292));
#12913=CARTESIAN_POINT('Ctrl Pts',(-203.252001679897,-96.9998452925596,
10.7496061270306));
#12914=CARTESIAN_POINT('Ctrl Pts',(-202.828144895504,-96.2815070524231,
10.8025755666321));
#12915=CARTESIAN_POINT('Ctrl Pts',(-202.601847813085,-95.8979863588357,
10.8308559435907));
#12916=CARTESIAN_POINT('Ctrl Pts',(-202.487206620518,-95.4485829044729,
10.8591363205494));
#12917=CARTESIAN_POINT('Ctrl Pts',(-202.486464107889,-94.9995333136293,
10.887416697508));
#12918=CARTESIAN_POINT('Ctrl Pts',(-202.481958443618,-94.9977164072965,
10.612583302492));
#12919=CARTESIAN_POINT('Ctrl Pts',(-202.488041246315,-95.6544050192081,
10.5710385486894));
#12920=CARTESIAN_POINT('Ctrl Pts',(-202.751257709045,-96.3154131318815,
10.5294937948868));
#12921=CARTESIAN_POINT('Ctrl Pts',(-203.212761635906,-96.7790430230964,
10.4879490410842));
#12922=CARTESIAN_POINT('Ctrl Pts',(-203.801177792993,-97.3701697785185,
10.4349796014828));
#12923=CARTESIAN_POINT('Ctrl Pts',(-204.711933530243,-97.6404350346142,
10.3820101618814));
#12924=CARTESIAN_POINT('Ctrl Pts',(-205.527543507365,-97.4659507083387,
10.3290407222799));
#12925=CARTESIAN_POINT('Ctrl Pts',(-206.343153484488,-97.2914663820631,
10.2760712826785));
#12926=CARTESIAN_POINT('Ctrl Pts',(-207.063617701482,-96.6722324734162,
10.223101843077));
#12927=CARTESIAN_POINT('Ctrl Pts',(-207.358679387517,-95.8921023455972,
10.1701324034756));
#12928=CARTESIAN_POINT('Ctrl Pts',(-207.653741073553,-95.1119722177781,
10.1171629638742));
#12929=CARTESIAN_POINT('Ctrl Pts',(-207.52340022863,-94.1709458707869,10.0641935242727));
#12930=CARTESIAN_POINT('Ctrl Pts',(-207.027404367665,-93.5003845232557,
10.0112240846713));
#12931=CARTESIAN_POINT('Ctrl Pts',(-206.5314085067,-92.8298231757246,9.95825464506987));
#12932=CARTESIAN_POINT('Ctrl Pts',(-205.669757629693,-92.4297268276535,
9.90528520546843));
#12933=CARTESIAN_POINT('Ctrl Pts',(-204.837427683417,-92.4834974091013,
9.852315765867));
#12934=CARTESIAN_POINT('Ctrl Pts',(-204.005097737141,-92.537267990549,9.79934632626556));
#12935=CARTESIAN_POINT('Ctrl Pts',(-203.202088721596,-93.0449055015156,
9.74637688666412));
#12936=CARTESIAN_POINT('Ctrl Pts',(-202.796495481975,-93.7737117438536,
9.69340744706269));
#12937=CARTESIAN_POINT('Ctrl Pts',(-202.590202149551,-94.1443980712782,
9.66646606553911));
#12938=CARTESIAN_POINT('Ctrl Pts',(-202.486718512095,-94.5722997665523,
9.63952468401554));
#12939=CARTESIAN_POINT('Ctrl Pts',(-202.486537790415,-95.0001194277165,
9.61258330249196));
#12940=CARTESIAN_POINT('Origin',(-205.,-95.,9.));
#12941=CARTESIAN_POINT('',(-202.48151911239,-95.0022302404453,8.61258330249196));
#12942=CARTESIAN_POINT('',(-202.478554974092,-94.9992065476435,8.88741669750803));
#12943=CARTESIAN_POINT('',(-202.4825,-95.,9.));
#12944=CARTESIAN_POINT('Ctrl Pts',(-202.478554974092,-94.9992065476435,
8.88741669750803));
#12945=CARTESIAN_POINT('Ctrl Pts',(-202.478376117211,-94.9558431822019,
8.89016971199881));
#12946=CARTESIAN_POINT('Ctrl Pts',(-202.47939772805,-94.9124884193367,8.89292272648959));
#12947=CARTESIAN_POINT('Ctrl Pts',(-202.481646252911,-94.8691973820566,
8.89567574098037));
#12948=CARTESIAN_POINT('Ctrl Pts',(-202.524909048014,-94.0362551682876,
8.94864518058181));
#12949=CARTESIAN_POINT('Ctrl Pts',(-203.022372640194,-93.2269040220556,
9.00161462018325));
#12950=CARTESIAN_POINT('Ctrl Pts',(-203.74600249882,-92.8121459858182,9.05458405978468));
#12951=CARTESIAN_POINT('Ctrl Pts',(-204.469632357446,-92.3973879495807,
9.10755349938612));
#12952=CARTESIAN_POINT('Ctrl Pts',(-205.419428482518,-92.3772230233378,
9.16052293898755));
#12953=CARTESIAN_POINT('Ctrl Pts',(-206.16000963814,-92.7608946965896,9.21349237858899));
#12954=CARTESIAN_POINT('Ctrl Pts',(-206.900590793762,-93.1445663698413,
9.26646181819042));
#12955=CARTESIAN_POINT('Ctrl Pts',(-207.431956979935,-93.9320746425879,
9.31943125779186));
#12956=CARTESIAN_POINT('Ctrl Pts',(-207.510532906401,-94.7624301235107,
9.3724006973933));
#12957=CARTESIAN_POINT('Ctrl Pts',(-207.589108832868,-95.5927856044335,
9.42537013699473));
#12958=CARTESIAN_POINT('Ctrl Pts',(-207.214894499628,-96.4659882935325,
9.47833957659616));
#12959=CARTESIAN_POINT('Ctrl Pts',(-206.559427665781,-96.9817669579278,
9.5313090161976));
#12960=CARTESIAN_POINT('Ctrl Pts',(-205.903960831934,-97.497545622323,9.58427845579904));
#12961=CARTESIAN_POINT('Ctrl Pts',(-204.96724149748,-97.6559002620145,9.63724789540048));
#12962=CARTESIAN_POINT('Ctrl Pts',(-204.178656570574,-97.3842419951162,
9.69021733500191));
#12963=CARTESIAN_POINT('Ctrl Pts',(-203.390071643667,-97.1125837282179,
9.74318677460335));
#12964=CARTESIAN_POINT('Ctrl Pts',(-202.749621124308,-96.4109125547298,
9.79615621420478));
#12965=CARTESIAN_POINT('Ctrl Pts',(-202.550883951478,-95.600870619362,9.84912565380621));
#12966=CARTESIAN_POINT('Ctrl Pts',(-202.502995622993,-95.4056803902987,
9.86188933504015));
#12967=CARTESIAN_POINT('Ctrl Pts',(-202.480754595229,-95.2041978054776,
9.87465301627409));
#12968=CARTESIAN_POINT('Ctrl Pts',(-202.482602555105,-95.0023130495141,
9.88741669750803));
#12969=CARTESIAN_POINT('Ctrl Pts',(-202.486537790415,-95.0001194277165,
9.61258330249196));
#12970=CARTESIAN_POINT('Ctrl Pts',(-202.486363195271,-95.4134358338514,
9.5865552444141));
#12971=CARTESIAN_POINT('Ctrl Pts',(-202.582606216335,-95.826675673577,9.56052718633624));
#12972=CARTESIAN_POINT('Ctrl Pts',(-202.775711594544,-96.1881734458707,
9.53449912825838));
#12973=CARTESIAN_POINT('Ctrl Pts',(-203.168698410431,-96.9238539318402,
9.48152968865694));
#12974=CARTESIAN_POINT('Ctrl Pts',(-203.962849505901,-97.4452399300696,
9.4285602490555));
#12975=CARTESIAN_POINT('Ctrl Pts',(-204.794130456823,-97.5133310126825,
9.37559080945407));
#12976=CARTESIAN_POINT('Ctrl Pts',(-205.625411407745,-97.5814220952953,
9.32262136985264));
#12977=CARTESIAN_POINT('Ctrl Pts',(-206.493822214119,-97.1962182622914,
9.26965193025121));
#12978=CARTESIAN_POINT('Ctrl Pts',(-207.001288215326,-96.5342947980481,
9.21668249064977));
#12979=CARTESIAN_POINT('Ctrl Pts',(-207.508754216533,-95.8723713338047,
9.16371305104833));
#12980=CARTESIAN_POINT('Ctrl Pts',(-207.655275412574,-94.9337282383218,
9.11074361144689));
#12981=CARTESIAN_POINT('Ctrl Pts',(-207.373687306002,-94.1486342610589,
9.05777417184546));
#12982=CARTESIAN_POINT('Ctrl Pts',(-207.092099199431,-93.363540283796,9.00480473224402));
#12983=CARTESIAN_POINT('Ctrl Pts',(-206.382401790246,-92.7319954247531,
8.95183529264259));
#12984=CARTESIAN_POINT('Ctrl Pts',(-205.569916404748,-92.5434963179922,
8.89886585304116));
#12985=CARTESIAN_POINT('Ctrl Pts',(-204.75743101925,-92.3549972112313,8.84589641343972));
#12986=CARTESIAN_POINT('Ctrl Pts',(-203.842157657439,-92.6095438567524,
8.79292697383828));
#12987=CARTESIAN_POINT('Ctrl Pts',(-203.243652513459,-93.1904534947564,
8.73995753423685));
#12988=CARTESIAN_POINT('Ctrl Pts',(-202.763915936522,-93.6560862533854,
8.69749945698855));
#12989=CARTESIAN_POINT('Ctrl Pts',(-202.487701419864,-94.3314056689759,
8.65504137974025));
#12990=CARTESIAN_POINT('Ctrl Pts',(-202.48151911239,-95.0022302404453,8.61258330249196));
#12991=CARTESIAN_POINT('Origin',(-205.,-95.,9.));
#12992=CARTESIAN_POINT('',(-202.479176535286,-94.9986328420086,7.61258330249196));
#12993=CARTESIAN_POINT('',(-202.484976587536,-94.9981409198179,7.88741669750803));
#12994=CARTESIAN_POINT('',(-202.4825,-95.,9.));
#12995=CARTESIAN_POINT('Ctrl Pts',(-202.484976587536,-94.9981409198179,
7.88741669750803));
#12996=CARTESIAN_POINT('Ctrl Pts',(-202.482996634039,-94.7084750992777,
7.90568640772353));
#12997=CARTESIAN_POINT('Ctrl Pts',(-202.529190054397,-94.4194213389179,
7.92395611793903));
#12998=CARTESIAN_POINT('Ctrl Pts',(-202.626312717846,-94.1486342696126,
7.94222582815454));
#12999=CARTESIAN_POINT('Ctrl Pts',(-202.907900821589,-93.3635403002374,
7.99519526775597));
#13000=CARTESIAN_POINT('Ctrl Pts',(-203.617598223643,-92.7319954475396,
8.04816470735741));
#13001=CARTESIAN_POINT('Ctrl Pts',(-204.430083600978,-92.5434963426725,
8.10113414695884));
#13002=CARTESIAN_POINT('Ctrl Pts',(-205.242568978313,-92.3549972378055,
8.15410358656028));
#13003=CARTESIAN_POINT('Ctrl Pts',(-206.157842330928,-92.6095438807692,
8.20707302616171));
#13004=CARTESIAN_POINT('Ctrl Pts',(-206.756347468895,-93.1904535129367,
8.26004246576315));
#13005=CARTESIAN_POINT('Ctrl Pts',(-207.354852606863,-93.7713631451043,
8.31301190536458));
#13006=CARTESIAN_POINT('Ctrl Pts',(-207.636589530182,-94.6786357664758,
8.36598134496602));
#13007=CARTESIAN_POINT('Ctrl Pts',(-207.472411607662,-95.4963826776137,
8.41895078456746));
#13008=CARTESIAN_POINT('Ctrl Pts',(-207.308233685142,-96.3141295887515,
8.47192022416889));
#13009=CARTESIAN_POINT('Ctrl Pts',(-206.698140916782,-97.0423507896557,
8.52488966377032));
#13010=CARTESIAN_POINT('Ctrl Pts',(-205.921796418158,-97.3472337514208,
8.57785910337176));
#13011=CARTESIAN_POINT('Ctrl Pts',(-205.145451919534,-97.6521167131859,
8.6308285429732));
#13012=CARTESIAN_POINT('Ctrl Pts',(-204.202855690646,-97.5336614358119,
8.68379798257464));
#13013=CARTESIAN_POINT('Ctrl Pts',(-203.526088575214,-97.0461671564718,
8.73676742217607));
#13014=CARTESIAN_POINT('Ctrl Pts',(-202.884495509002,-96.5840097284425,
8.78698384728673));
#13015=CARTESIAN_POINT('Ctrl Pts',(-202.481817417207,-95.7901770276534,
8.83720027239738));
#13016=CARTESIAN_POINT('Ctrl Pts',(-202.478554974092,-94.9992065476435,
8.88741669750803));
#13017=CARTESIAN_POINT('Ctrl Pts',(-202.48151911239,-95.0022302404453,8.61258330249196));
#13018=CARTESIAN_POINT('Ctrl Pts',(-202.479988556174,-95.1683065350657,
8.60207194013882));
#13019=CARTESIAN_POINT('Ctrl Pts',(-202.495008569329,-95.334107335775,8.59156057778568));
#13020=CARTESIAN_POINT('Ctrl Pts',(-202.527588367498,-95.4963826826008,
8.58104921543254));
#13021=CARTESIAN_POINT('Ctrl Pts',(-202.691766291667,-96.3141296019545,
8.5280797758311));
#13022=CARTESIAN_POINT('Ctrl Pts',(-203.301859066157,-97.0423508101752,
8.47511033622967));
#13023=CARTESIAN_POINT('Ctrl Pts',(-204.078203572581,-97.3472337750034,
8.42214089662823));
#13024=CARTESIAN_POINT('Ctrl Pts',(-204.854548079005,-97.6521167398316,
8.36917145702679));
#13025=CARTESIAN_POINT('Ctrl Pts',(-205.797144317363,-97.5336614612674,
8.31620201742536));
#13026=CARTESIAN_POINT('Ctrl Pts',(-206.473911439594,-97.0461671770295,
8.26323257782393));
#13027=CARTESIAN_POINT('Ctrl Pts',(-207.150678561825,-96.5586728927915,
8.21026313822249));
#13028=CARTESIAN_POINT('Ctrl Pts',(-207.561616567928,-95.70213960288,8.15729369862105));
#13029=CARTESIAN_POINT('Ctrl Pts',(-207.518353772391,-94.8691973807424,
8.10432425901962));
#13030=CARTESIAN_POINT('Ctrl Pts',(-207.475090976853,-94.0362551586049,
8.05135481941818));
#13031=CARTESIAN_POINT('Ctrl Pts',(-206.977627379675,-93.2269040042414,
7.99838537981675));
#13032=CARTESIAN_POINT('Ctrl Pts',(-206.253997513779,-92.8121459638369,
7.94541594021531));
#13033=CARTESIAN_POINT('Ctrl Pts',(-205.530367647883,-92.3973879234324,
7.89244650061388));
#13034=CARTESIAN_POINT('Ctrl Pts',(-204.580571513268,-92.3772229969869,
7.83947706101244));
#13035=CARTESIAN_POINT('Ctrl Pts',(-203.839990350206,-92.7608946740935,
7.78650762141101));
#13036=CARTESIAN_POINT('Ctrl Pts',(-203.099409187143,-93.1445663512,7.73353818180957));
#13037=CARTESIAN_POINT('Ctrl Pts',(-202.568042995632,-93.9320746318586,
7.68056874220814));
#13038=CARTESIAN_POINT('Ctrl Pts',(-202.489467068376,-94.7624301211239,
7.6275993026067));
#13039=CARTESIAN_POINT('Ctrl Pts',(-202.482042056636,-94.8408943463822,
7.62259396923512));
#13040=CARTESIAN_POINT('Ctrl Pts',(-202.478660124946,-94.9197411653224,
7.61758863586354));
#13041=CARTESIAN_POINT('Ctrl Pts',(-202.479176535286,-94.9986328420086,
7.61258330249196));
#13042=CARTESIAN_POINT('Origin',(-205.,-95.,9.));
#13043=CARTESIAN_POINT('',(-202.485695966289,-94.9985525878773,6.61258330249196));
#13044=CARTESIAN_POINT('',(-202.48529106324,-95.001705225411,6.88741669750803));
#13045=CARTESIAN_POINT('',(-202.4825,-95.,9.));
#13046=CARTESIAN_POINT('Ctrl Pts',(-202.48529106324,-95.001705225411,6.88741669750803));
#13047=CARTESIAN_POINT('Ctrl Pts',(-202.488622939146,-94.465854223785,6.92120310344825));
#13048=CARTESIAN_POINT('Ctrl Pts',(-202.656226110927,-93.9281001765914,
6.95498950938847));
#13049=CARTESIAN_POINT('Ctrl Pts',(-202.972595652704,-93.5003845383223,
6.9887759153287));
#13050=CARTESIAN_POINT('Ctrl Pts',(-203.468591508686,-92.8298231975282,
7.04174535493013));
#13051=CARTESIAN_POINT('Ctrl Pts',(-204.330242377036,-92.429726853477,7.09471479453157));
#13052=CARTESIAN_POINT('Ctrl Pts',(-205.162572314949,-92.4834974343845,
7.14768423413301));
#13053=CARTESIAN_POINT('Ctrl Pts',(-205.994902252863,-92.537268015292,7.20065367373444));
#13054=CARTESIAN_POINT('Ctrl Pts',(-206.797911260341,-93.0449055211583,
7.25362311333587));
#13055=CARTESIAN_POINT('Ctrl Pts',(-207.203504495887,-93.773711756174,7.30659255293731));
#13056=CARTESIAN_POINT('Ctrl Pts',(-207.609097731433,-94.5025179911897,
7.35956199253874));
#13057=CARTESIAN_POINT('Ctrl Pts',(-207.617275195047,-95.452492955355,7.41253143214018));
#13058=CARTESIAN_POINT('Ctrl Pts',(-207.224288383109,-96.1881734339332,
7.46550087174162));
#13059=CARTESIAN_POINT('Ctrl Pts',(-206.83130157117,-96.9238539125113,7.51847031134306));
#13060=CARTESIAN_POINT('Ctrl Pts',(-206.037150483679,-97.4452399055024,
7.57143975094449));
#13061=CARTESIAN_POINT('Ctrl Pts',(-205.205869541108,-97.5133309874311,
7.62440919054592));
#13062=CARTESIAN_POINT('Ctrl Pts',(-204.374588598538,-97.5814220693598,
7.67737863014736));
#13063=CARTESIAN_POINT('Ctrl Pts',(-203.50617780089,-97.1962182402261,7.7303480697488));
#13064=CARTESIAN_POINT('Ctrl Pts',(-202.998711804781,-96.5342947826331,
7.78331750935023));
#13065=CARTESIAN_POINT('Ctrl Pts',(-202.666276104686,-96.1006756047542,
7.81801723873617));
#13066=CARTESIAN_POINT('Ctrl Pts',(-202.488737120666,-95.5483043031743,
7.8527169681221));
#13067=CARTESIAN_POINT('Ctrl Pts',(-202.484976587536,-94.9981409198179,
7.88741669750803));
#13068=CARTESIAN_POINT('Ctrl Pts',(-202.479176535286,-94.9986328420086,
7.61258330249196));
#13069=CARTESIAN_POINT('Ctrl Pts',(-202.484125088871,-95.7546202019532,
7.5646191962621));
#13070=CARTESIAN_POINT('Ctrl Pts',(-202.847043646147,-96.514726679039,7.51665509003225));
#13071=CARTESIAN_POINT('Ctrl Pts',(-203.440572318551,-96.9817669778385,
7.46869098380239));
#13072=CARTESIAN_POINT('Ctrl Pts',(-204.096039158984,-97.4975456474158,
7.41572154420096));
#13073=CARTESIAN_POINT('Ctrl Pts',(-205.032758502849,-97.6559002886982,
7.36275210459952));
#13074=CARTESIAN_POINT('Ctrl Pts',(-205.821343437678,-97.3842420190706,
7.30978266499809));
#13075=CARTESIAN_POINT('Ctrl Pts',(-206.609928372508,-97.1125837494429,
7.25681322539665));
#13076=CARTESIAN_POINT('Ctrl Pts',(-207.250378898302,-96.4109125689051,
7.20384378579521));
#13077=CARTESIAN_POINT('Ctrl Pts',(-207.449116073128,-95.6008706253988,
7.15087434619378));
#13078=CARTESIAN_POINT('Ctrl Pts',(-207.647853247953,-94.7908286818925,
7.09790490659234));
#13079=CARTESIAN_POINT('Ctrl Pts',(-207.404877071811,-93.8724159754179,
7.04493546699091));
#13080=CARTESIAN_POINT('Ctrl Pts',(-206.831566465997,-93.2666277581682,
6.99196602738948));
#13081=CARTESIAN_POINT('Ctrl Pts',(-206.258255860184,-92.6608395409186,
6.93899658778804));
#13082=CARTESIAN_POINT('Ctrl Pts',(-205.354610824698,-92.367675812894,6.8860271481866));
#13083=CARTESIAN_POINT('Ctrl Pts',(-204.53485719388,-92.5215211887057,6.83305770858517));
#13084=CARTESIAN_POINT('Ctrl Pts',(-203.715103563063,-92.6753665645175,
6.78008826898373));
#13085=CARTESIAN_POINT('Ctrl Pts',(-202.979241336913,-93.2762210441657,
6.72711882938229));
#13086=CARTESIAN_POINT('Ctrl Pts',(-202.664585647609,-94.0486562919927,
6.67414938978086));
#13087=CARTESIAN_POINT('Ctrl Pts',(-202.542678123954,-94.3479220337145,
6.65362736068456));
#13088=CARTESIAN_POINT('Ctrl Pts',(-202.48399503341,-94.6729425913092,6.63310533158826));
#13089=CARTESIAN_POINT('Ctrl Pts',(-202.485695966289,-94.9985525878773,
6.61258330249196));
#13090=CARTESIAN_POINT('Origin',(-205.,-95.,9.));
#13091=CARTESIAN_POINT('',(-202.484465718496,-95.0020481324837,5.61258330249196));
#13092=CARTESIAN_POINT('',(-202.478772638074,-95.0010375285769,5.88741669750803));
#13093=CARTESIAN_POINT('',(-202.4825,-95.,9.));
#13094=CARTESIAN_POINT('Ctrl Pts',(-202.478772638074,-95.0010375285769,
5.88741669750803));
#13095=CARTESIAN_POINT('Ctrl Pts',(-202.482817019795,-94.2242747158738,
5.93671979917297));
#13096=CARTESIAN_POINT('Ctrl Pts',(-202.869063144179,-93.4440379428825,
5.98602290083791));
#13097=CARTESIAN_POINT('Ctrl Pts',(-203.491082445535,-92.9795092838211,
6.03532600250286));
#13098=CARTESIAN_POINT('Ctrl Pts',(-204.159357111864,-92.4804367727953,
6.08829544210429));
#13099=CARTESIAN_POINT('Ctrl Pts',(-205.099774465356,-92.345772357668,6.14126488170573));
#13100=CARTESIAN_POINT('Ctrl Pts',(-205.881252446597,-92.6372454537756,
6.19423432130716));
#13101=CARTESIAN_POINT('Ctrl Pts',(-206.662730427838,-92.9287185498831,
6.2472037609086));
#13102=CARTESIAN_POINT('Ctrl Pts',(-207.285269036827,-93.6463291572254,
6.30017320051003));
#13103=CARTESIAN_POINT('Ctrl Pts',(-207.463500054196,-94.4611285836895,
6.35314264011147));
#13104=CARTESIAN_POINT('Ctrl Pts',(-207.641731071564,-95.2759280101535,
6.4061120797129));
#13105=CARTESIAN_POINT('Ctrl Pts',(-207.375654497314,-96.1879162557393,
6.45908151931434));
#13106=CARTESIAN_POINT('Ctrl Pts',(-206.787238346138,-96.7790430052224,
6.51205095891577));
#13107=CARTESIAN_POINT('Ctrl Pts',(-206.198822194963,-97.3701697547055,
6.56502039851721));
#13108=CARTESIAN_POINT('Ctrl Pts',(-205.288066466863,-97.6404350080859,
6.61798983811865));
#13109=CARTESIAN_POINT('Ctrl Pts',(-204.472456497935,-97.4659506835634,
6.67095927772009));
#13110=CARTESIAN_POINT('Ctrl Pts',(-203.656846529007,-97.2914663590408,
6.72392871732152));
#13111=CARTESIAN_POINT('Ctrl Pts',(-202.936382319251,-96.6722324566154,
6.77689815692296));
#13112=CARTESIAN_POINT('Ctrl Pts',(-202.64132063618,-95.8921023366343,6.82986759652439));
#13113=CARTESIAN_POINT('Ctrl Pts',(-202.534463205913,-95.6095759881524,
6.84905063018561));
#13114=CARTESIAN_POINT('Ctrl Pts',(-202.483399311635,-95.305947346333,6.86823366384682));
#13115=CARTESIAN_POINT('Ctrl Pts',(-202.48529106324,-95.001705225411,6.88741669750803));
#13116=CARTESIAN_POINT('Ctrl Pts',(-202.485695966289,-94.9985525878773,
6.61258330249196));
#13117=CARTESIAN_POINT('Ctrl Pts',(-202.488385313776,-95.5133750342175,
6.58013589198682));
#13118=CARTESIAN_POINT('Ctrl Pts',(-202.642027587202,-96.0296710083661,
6.54768848148169));
#13119=CARTESIAN_POINT('Ctrl Pts',(-202.935395877166,-96.4479726738087,
6.51524107097655));
#13120=CARTESIAN_POINT('Ctrl Pts',(-203.414310948487,-97.1308377917921,
6.46227163137512));
#13121=CARTESIAN_POINT('Ctrl Pts',(-204.26559024359,-97.5525520117532,6.40930219177368));
#13122=CARTESIAN_POINT('Ctrl Pts',(-205.099012090884,-97.5198038919682,
6.35633275217224));
#13123=CARTESIAN_POINT('Ctrl Pts',(-205.932433938178,-97.4870557721831,
6.30336331257081));
#13124=CARTESIAN_POINT('Ctrl Pts',(-206.747998337665,-96.9998453126519,
6.25039387296938));
#13125=CARTESIAN_POINT('Ctrl Pts',(-207.171855126317,-96.2815070652983,
6.19742443336794));
#13126=CARTESIAN_POINT('Ctrl Pts',(-207.595711914969,-95.5631688179448,
6.14445499376651));
#13127=CARTESIAN_POINT('Ctrl Pts',(-207.627861092786,-94.6137027827689,
6.09148555416507));
#13128=CARTESIAN_POINT('Ctrl Pts',(-207.253565656318,-93.8683388843025,
6.03851611456364));
#13129=CARTESIAN_POINT('Ctrl Pts',(-206.879270219851,-93.1229749858362,
5.9855466749622));
#13130=CARTESIAN_POINT('Ctrl Pts',(-206.0985301691,-92.5817132240792,5.93257723536076));
#13131=CARTESIAN_POINT('Ctrl Pts',(-205.269232380244,-92.4926649658358,
5.87960779575933));
#13132=CARTESIAN_POINT('Ctrl Pts',(-204.439934591389,-92.4036167075924,
5.82663835615789));
#13133=CARTESIAN_POINT('Ctrl Pts',(-203.562079064428,-92.7667819528624,
5.77366891655646));
#13134=CARTESIAN_POINT('Ctrl Pts',(-203.038069867117,-93.4156877827256,
5.72069947695502));
#13135=CARTESIAN_POINT('Ctrl Pts',(-202.681550647588,-93.8571827053293,
5.684660752134));
#13136=CARTESIAN_POINT('Ctrl Pts',(-202.488827231246,-94.430947216833,5.64862202731298));
#13137=CARTESIAN_POINT('Ctrl Pts',(-202.484465718496,-95.0020481324837,
5.61258330249196));
#13138=CARTESIAN_POINT('Origin',(-205.,-95.,9.));
#13139=CARTESIAN_POINT('',(-202.478335348143,-95.0004148939562,4.61258330249195));
#13140=CARTESIAN_POINT('',(-202.482163763775,-94.997700765499,4.88741669750803));
#13141=CARTESIAN_POINT('',(-202.4825,-95.,9.));
#13142=CARTESIAN_POINT('Ctrl Pts',(-202.482163763775,-94.997700765499,4.88741669750803));
#13143=CARTESIAN_POINT('Ctrl Pts',(-202.480430648174,-94.8103456723384,
4.89926705529626));
#13144=CARTESIAN_POINT('Ctrl Pts',(-202.499567671021,-94.6233413479286,
4.91111741308448));
#13145=CARTESIAN_POINT('Ctrl Pts',(-202.540902956965,-94.4413796877348,
4.92296777087271));
#13146=CARTESIAN_POINT('Ctrl Pts',(-202.725665895886,-93.6280365514634,
4.97593721047414));
#13147=CARTESIAN_POINT('Ctrl Pts',(-203.353942315917,-92.9154440708087,
5.02890665007558));
#13148=CARTESIAN_POINT('Ctrl Pts',(-204.137733817173,-92.6302506566537,
5.08187608967701));
#13149=CARTESIAN_POINT('Ctrl Pts',(-204.921525318429,-92.3450572424987,
5.13484552927845));
#13150=CARTESIAN_POINT('Ctrl Pts',(-205.86083190091,-92.4872628948432,5.18781496887989));
#13151=CARTESIAN_POINT('Ctrl Pts',(-206.525080676425,-92.9916813373541,
5.24078440848132));
#13152=CARTESIAN_POINT('Ctrl Pts',(-207.189329451941,-93.496099779865,5.29375384808276));
#13153=CARTESIAN_POINT('Ctrl Pts',(-207.578520420489,-94.3627310125423,
5.34672328768419));
#13154=CARTESIAN_POINT('Ctrl Pts',(-207.514250617043,-95.1943161214058,
5.39969272728563));
#13155=CARTESIAN_POINT('Ctrl Pts',(-207.449980813596,-96.0259012302693,
5.45266216688706));
#13156=CARTESIAN_POINT('Ctrl Pts',(-206.932250238154,-96.8224402153189,
5.5056316064885));
#13157=CARTESIAN_POINT('Ctrl Pts',(-206.198383693215,-97.2188040571838,
5.55860104608993));
#13158=CARTESIAN_POINT('Ctrl Pts',(-205.464517148276,-97.6151678990486,
5.61157048569137));
#13159=CARTESIAN_POINT('Ctrl Pts',(-204.51451463384,-97.6113565977286,5.66453992529281));
#13160=CARTESIAN_POINT('Ctrl Pts',(-203.783851993534,-97.2091172324499,
5.71750936489424));
#13161=CARTESIAN_POINT('Ctrl Pts',(-203.053189353228,-96.8068778671711,
5.77047880449568));
#13162=CARTESIAN_POINT('Ctrl Pts',(-202.541866587052,-96.0062104379335,
5.82344824409711));
#13163=CARTESIAN_POINT('Ctrl Pts',(-202.484271193547,-95.1741364198525,
5.87641768369855));
#13164=CARTESIAN_POINT('Ctrl Pts',(-202.48028466513,-95.1165435028532,5.88008402163504));
#13165=CARTESIAN_POINT('Ctrl Pts',(-202.478471884782,-95.0588001210244,
5.88375035957154));
#13166=CARTESIAN_POINT('Ctrl Pts',(-202.478772638074,-95.0010375285769,
5.88741669750803));
#13167=CARTESIAN_POINT('Ctrl Pts',(-202.484465718496,-95.0020481324837,
5.61258330249196));
#13168=CARTESIAN_POINT('Ctrl Pts',(-202.482416713467,-95.2703469350006,
5.59565258771154));
#13169=CARTESIAN_POINT('Ctrl Pts',(-202.521940082511,-95.5380578691583,
5.57872187293113));
#13170=CARTESIAN_POINT('Ctrl Pts',(-202.605582971729,-95.7911903328824,
5.56179115815071));
#13171=CARTESIAN_POINT('Ctrl Pts',(-202.867268141315,-96.5831406387199,
5.50882171854928));
#13172=CARTESIAN_POINT('Ctrl Pts',(-203.560801348149,-97.2323948359386,
5.45585227894784));
#13173=CARTESIAN_POINT('Ctrl Pts',(-204.368270845956,-97.4413384288235,
5.40288283934641));
#13174=CARTESIAN_POINT('Ctrl Pts',(-205.175740343764,-97.6502820217083,
5.34991339974497));
#13175=CARTESIAN_POINT('Ctrl Pts',(-206.097146132545,-97.4189150102591,
5.29694396014354));
#13176=CARTESIAN_POINT('Ctrl Pts',(-206.710120947904,-96.8532947395539,
5.2439745205421));
#13177=CARTESIAN_POINT('Ctrl Pts',(-207.323095763263,-96.2876744688487,
5.19100508094066));
#13178=CARTESIAN_POINT('Ctrl Pts',(-207.6276396052,-95.3878009388875,5.13803564133923));
#13179=CARTESIAN_POINT('Ctrl Pts',(-207.484151278482,-94.5661711469537,
5.08506620173779));
#13180=CARTESIAN_POINT('Ctrl Pts',(-207.340662951764,-93.74454135502,5.03209676213636));
#13181=CARTESIAN_POINT('Ctrl Pts',(-206.749142456392,-93.0011553011137,
4.97912732253492));
#13182=CARTESIAN_POINT('Ctrl Pts',(-205.980739481793,-92.6767769980105,
4.92615788293349));
#13183=CARTESIAN_POINT('Ctrl Pts',(-205.212336507194,-92.3523986949072,
4.87318844333205));
#13184=CARTESIAN_POINT('Ctrl Pts',(-204.267051053368,-92.447028142607,4.82021900373062));
#13185=CARTESIAN_POINT('Ctrl Pts',(-203.578196689718,-92.917287731109,4.76724956412918));
#13186=CARTESIAN_POINT('Ctrl Pts',(-202.907731291558,-93.3749937410897,
4.71569414358344));
#13187=CARTESIAN_POINT('Ctrl Pts',(-202.480188867636,-94.1885426831987,
4.6641387230377));
#13188=CARTESIAN_POINT('Ctrl Pts',(-202.478335348143,-95.0004148939562,
4.61258330249195));
#13189=CARTESIAN_POINT('Origin',(-205.,-95.,9.));
#13190=CARTESIAN_POINT('',(-202.483233733754,-94.9977147790846,3.61258330249195));
#13191=CARTESIAN_POINT('',(-202.486523858474,-95.0002304794208,3.88741669750803));
#13192=CARTESIAN_POINT('',(-202.4825,-95.,9.));
#13193=CARTESIAN_POINT('Ctrl Pts',(-202.486523858474,-95.0002304794208,
3.88741669750803));
#13194=CARTESIAN_POINT('Ctrl Pts',(-202.486878246653,-94.5656573186005,
3.91478375102098));
#13195=CARTESIAN_POINT('Ctrl Pts',(-202.593838479751,-94.1309207445616,
3.94215080453392));
#13196=CARTESIAN_POINT('Ctrl Pts',(-202.80640573248,-93.7560710993726,3.96951785804687));
#13197=CARTESIAN_POINT('Ctrl Pts',(-203.217833592236,-93.0305426594524,
4.02248729764831));
#13198=CARTESIAN_POINT('Ctrl Pts',(-204.024889852448,-92.5293645510928,
4.07545673724974));
#13199=CARTESIAN_POINT('Ctrl Pts',(-204.8576244336,-92.4822740183969,4.12842617685117));
#13200=CARTESIAN_POINT('Ctrl Pts',(-205.690359014752,-92.435183485701,4.18139561645261));
#13201=CARTESIAN_POINT('Ctrl Pts',(-206.548771916843,-92.8421805286688,
4.23436505605405));
#13202=CARTESIAN_POINT('Ctrl Pts',(-207.0393714627,-93.5166999772584,4.28733449565548));
#13203=CARTESIAN_POINT('Ctrl Pts',(-207.529971008557,-94.1912194258479,
4.34030393525692));
#13204=CARTESIAN_POINT('Ctrl Pts',(-207.65275719818,-95.1332612800593,4.39327337485835));
#13205=CARTESIAN_POINT('Ctrl Pts',(-207.351445528426,-95.9109988184287,
4.44624281445978));
#13206=CARTESIAN_POINT('Ctrl Pts',(-207.050133858673,-96.688736356798,4.49921225406122));
#13207=CARTESIAN_POINT('Ctrl Pts',(-206.324724329544,-97.3021695793252,
4.55218169366266));
#13208=CARTESIAN_POINT('Ctrl Pts',(-205.507740615314,-97.4701041249105,
4.6051511332641));
#13209=CARTESIAN_POINT('Ctrl Pts',(-204.690756901084,-97.6380386704957,
4.65812057286553));
#13210=CARTESIAN_POINT('Ctrl Pts',(-203.782199001753,-97.3604745391391,
4.71109001246697));
#13211=CARTESIAN_POINT('Ctrl Pts',(-203.198544780993,-96.7646455775167,
4.7640594520684));
#13212=CARTESIAN_POINT('Ctrl Pts',(-202.745466065518,-96.3021158621945,
4.80517853388161));
#13213=CARTESIAN_POINT('Ctrl Pts',(-202.488177432177,-95.6477966985894,
4.84629761569482));
#13214=CARTESIAN_POINT('Ctrl Pts',(-202.482163763775,-94.997700765499,4.88741669750803));
#13215=CARTESIAN_POINT('Ctrl Pts',(-202.478335348143,-95.0004148939562,
4.61258330249195));
#13216=CARTESIAN_POINT('Ctrl Pts',(-202.478284511357,-95.0226822475079,
4.61116928343626));
#13217=CARTESIAN_POINT('Ctrl Pts',(-202.478553898799,-95.0449483397394,
4.60975526438057));
#13218=CARTESIAN_POINT('Ctrl Pts',(-202.479147281308,-95.0672057942804,
4.60834124532487));
#13219=CARTESIAN_POINT('Ctrl Pts',(-202.50137551002,-95.9009745396454,4.55537180572344));
#13220=CARTESIAN_POINT('Ctrl Pts',(-202.978255240917,-96.7226223010713,
4.502402366122));
#13221=CARTESIAN_POINT('Ctrl Pts',(-203.691187470346,-97.155510336405,4.44943292652057));
#13222=CARTESIAN_POINT('Ctrl Pts',(-204.404119699775,-97.5883983717386,
4.39646348691913));
#13223=CARTESIAN_POINT('Ctrl Pts',(-205.353104427737,-97.6325266809801,
4.34349404731769));
#13224=CARTESIAN_POINT('Ctrl Pts',(-206.103132358242,-97.2676670937981,
4.29052460771626));
#13225=CARTESIAN_POINT('Ctrl Pts',(-206.853160288746,-96.9028075066161,
4.23755516811482));
#13226=CARTESIAN_POINT('Ctrl Pts',(-207.404231421792,-96.1289600230108,
4.18458572851339));
#13227=CARTESIAN_POINT('Ctrl Pts',(-207.503737829587,-95.3008520048615,
4.13161628891195));
#13228=CARTESIAN_POINT('Ctrl Pts',(-207.603244237383,-94.4727439867123,
4.07864684931052));
#13229=CARTESIAN_POINT('Ctrl Pts',(-207.251185919929,-93.5903754340193,
4.02567740970908));
#13230=CARTESIAN_POINT('Ctrl Pts',(-206.60894444252,-93.058219160391,3.97270797010765));
#13231=CARTESIAN_POINT('Ctrl Pts',(-205.966702965111,-92.5260628867627,
3.91973853050621));
#13232=CARTESIAN_POINT('Ctrl Pts',(-205.034278327748,-92.3441188921993,
3.86676909090478));
#13233=CARTESIAN_POINT('Ctrl Pts',(-204.239088773406,-92.5957892868688,
3.81379965130334));
#13234=CARTESIAN_POINT('Ctrl Pts',(-203.443899219063,-92.8474596815382,
3.7608302117019));
#13235=CARTESIAN_POINT('Ctrl Pts',(-202.78594474774,-93.5327444654406,3.70786077210047));
#13236=CARTESIAN_POINT('Ctrl Pts',(-202.566828012252,-94.3375129236185,
3.65489133249903));
#13237=CARTESIAN_POINT('Ctrl Pts',(-202.508489987599,-94.5517758919359,
3.64078865583001));
#13238=CARTESIAN_POINT('Ctrl Pts',(-202.481258832434,-94.7745084214562,
3.62668597916098));
#13239=CARTESIAN_POINT('Ctrl Pts',(-202.483233733754,-94.9977147790846,
3.61258330249195));
#13240=CARTESIAN_POINT('Origin',(-205.,-95.,9.));
#13241=CARTESIAN_POINT('',(-202.486303966252,-95.0008035932749,2.61258330249195));
#13242=CARTESIAN_POINT('',(-202.481315987002,-95.0021961802459,2.88741669750803));
#13243=CARTESIAN_POINT('',(-202.4825,-95.,9.));
#13244=CARTESIAN_POINT('Ctrl Pts',(-202.481315987002,-95.0021961802459,
2.88741669750803));
#13245=CARTESIAN_POINT('Ctrl Pts',(-202.487520204672,-94.3247868793523,
2.9303004467457));
#13246=CARTESIAN_POINT('Ctrl Pts',(-202.769924023565,-93.6428175431098,
2.97318419598336));
#13247=CARTESIAN_POINT('Ctrl Pts',(-203.258228221064,-93.1764194592973,
3.01606794522103));
#13248=CARTESIAN_POINT('Ctrl Pts',(-203.861375104355,-92.6003307177601,
3.06903738482246));
#13249=CARTESIAN_POINT('Ctrl Pts',(-204.778661384897,-92.353136093667,3.1220068244239));
#13250=CARTESIAN_POINT('Ctrl Pts',(-205.589608158919,-92.5481482223093,
3.17497626402534));
#13251=CARTESIAN_POINT('Ctrl Pts',(-206.400554932941,-92.7431603509516,
3.22794570362677));
#13252=CARTESIAN_POINT('Ctrl Pts',(-207.105162200444,-93.3803792323294,
3.28091514322821));
#13253=CARTESIAN_POINT('Ctrl Pts',(-207.380441927112,-94.1677072917534,
3.33388458282964));
#13254=CARTESIAN_POINT('Ctrl Pts',(-207.655721653779,-94.9550353511775,
3.38685402243108));
#13255=CARTESIAN_POINT('Ctrl Pts',(-207.50167383961,-95.8924725886478,3.43982346203251));
#13256=CARTESIAN_POINT('Ctrl Pts',(-206.988913141991,-96.5503030135196,
3.49279290163395));
#13257=CARTESIAN_POINT('Ctrl Pts',(-206.476152444371,-97.2081334383915,
3.54576234123538));
#13258=CARTESIAN_POINT('Ctrl Pts',(-205.604678863301,-97.5863570506648,
3.59873178083682));
#13259=CARTESIAN_POINT('Ctrl Pts',(-204.773971018082,-97.5115982600209,
3.65170122043826));
#13260=CARTESIAN_POINT('Ctrl Pts',(-203.943263172863,-97.4368394693769,
3.70467066003969));
#13261=CARTESIAN_POINT('Ctrl Pts',(-203.153321063494,-96.9090982758155,
3.75764009964112));
#13262=CARTESIAN_POINT('Ctrl Pts',(-202.766249738459,-96.1702882932945,
3.81060953924256));
#13263=CARTESIAN_POINT('Ctrl Pts',(-202.57916168199,-95.8131899633733,3.83621192533105));
#13264=CARTESIAN_POINT('Ctrl Pts',(-202.486192321761,-95.4067817306088,
3.86181431141954));
#13265=CARTESIAN_POINT('Ctrl Pts',(-202.486523858474,-95.0002304794208,
3.88741669750803));
#13266=CARTESIAN_POINT('Ctrl Pts',(-202.483233733754,-94.9977147790846,
3.61258330249195));
#13267=CARTESIAN_POINT('Ctrl Pts',(-202.488676531827,-95.6128681141961,
3.57371653955955));
#13268=CARTESIAN_POINT('Ctrl Pts',(-202.715952540883,-96.2316203881349,
3.53484977662714));
#13269=CARTESIAN_POINT('Ctrl Pts',(-203.125272134475,-96.6865973078459,
3.49598301369473));
#13270=CARTESIAN_POINT('Ctrl Pts',(-203.683111991839,-97.3066611014422,
3.44301357409329));
#13271=CARTESIAN_POINT('Ctrl Pts',(-204.579070706222,-97.6225365561815,
3.39004413449185));
#13272=CARTESIAN_POINT('Ctrl Pts',(-205.402445810223,-97.4894281303028,
3.33707469489042));
#13273=CARTESIAN_POINT('Ctrl Pts',(-206.225820914224,-97.3563197044241,
3.28410525528898));
#13274=CARTESIAN_POINT('Ctrl Pts',(-206.976612407843,-96.7742273979274,
3.23113581568755));
#13275=CARTESIAN_POINT('Ctrl Pts',(-207.310661665506,-96.0099790681416,
3.17816637608611));
#13276=CARTESIAN_POINT('Ctrl Pts',(-207.644710923168,-95.2457307383558,
3.12519693648468));
#13277=CARTESIAN_POINT('Ctrl Pts',(-207.562017944873,-94.2993263852809,
3.07222749688324));
#13278=CARTESIAN_POINT('Ctrl Pts',(-207.100488731034,-93.6045924816996,
3.01925805728181));
#13279=CARTESIAN_POINT('Ctrl Pts',(-206.638959517195,-92.9098585781182,
2.96628861768037));
#13280=CARTESIAN_POINT('Ctrl Pts',(-205.798594067812,-92.4667951240303,
2.91331917807893));
#13281=CARTESIAN_POINT('Ctrl Pts',(-204.964611205932,-92.4784999179239,
2.8603497384775));
#13282=CARTESIAN_POINT('Ctrl Pts',(-204.130628344053,-92.4902047118176,
2.80738029887606));
#13283=CARTESIAN_POINT('Ctrl Pts',(-203.303028069677,-92.9566777536927,
2.75441085927463));
#13284=CARTESIAN_POINT('Ctrl Pts',(-202.861177729107,-93.6640904345609,
2.70144141967319));
#13285=CARTESIAN_POINT('Ctrl Pts',(-202.614104513341,-94.0596604044974,
2.67182204727945));
#13286=CARTESIAN_POINT('Ctrl Pts',(-202.487647821326,-94.5305675271913,
2.6422026748857));
#13287=CARTESIAN_POINT('Ctrl Pts',(-202.486303966252,-95.0008035932749,
2.61258330249195));
#13288=CARTESIAN_POINT('Origin',(-205.,-95.,9.));
#13289=CARTESIAN_POINT('',(-202.480282573446,-95.0019224211138,1.61258330249195));
#13290=CARTESIAN_POINT('',(-202.479323384637,-94.9985362448309,1.88741669750803));
#13291=CARTESIAN_POINT('',(-202.4825,-95.,9.));
#13292=CARTESIAN_POINT('Ctrl Pts',(-202.479323384637,-94.9985362448309,
1.88741669750803));
#13293=CARTESIAN_POINT('Ctrl Pts',(-202.478731654615,-94.9129221908085,
1.89284770286898));
#13294=CARTESIAN_POINT('Ctrl Pts',(-202.482714729456,-94.8273638427469,
1.89827870822993));
#13295=CARTESIAN_POINT('Ctrl Pts',(-202.49145403661,-94.7422941092908,1.90370971359088));
#13296=CARTESIAN_POINT('Ctrl Pts',(-202.576689857917,-93.912595773765,1.95667915319232));
#13297=CARTESIAN_POINT('Ctrl Pts',(-203.114357719001,-93.1293764342375,
2.00964859279375));
#13298=CARTESIAN_POINT('Ctrl Pts',(-203.857993504046,-92.7516592929174,
2.06261803239519));
#13299=CARTESIAN_POINT('Ctrl Pts',(-204.60162928909,-92.3739421515973,2.11558747199662));
#13300=CARTESIAN_POINT('Ctrl Pts',(-205.551232998096,-92.4017272084846,
2.16855691159806));
#13301=CARTESIAN_POINT('Ctrl Pts',(-206.271511681291,-92.8222780291104,
2.22152635119949));
#13302=CARTESIAN_POINT('Ctrl Pts',(-206.991790364487,-93.2428288497361,
2.27449579080093));
#13303=CARTESIAN_POINT('Ctrl Pts',(-207.482744021872,-94.0561454341005,
2.32746523040236));
#13304=CARTESIAN_POINT('Ctrl Pts',(-207.519322200074,-94.8894079662103,
2.3804346700038));
#13305=CARTESIAN_POINT('Ctrl Pts',(-207.555900378275,-95.7226704983201,
2.43340410960524));
#13306=CARTESIAN_POINT('Ctrl Pts',(-207.138103077293,-96.5758789781754,
2.48637354920667));
#13307=CARTESIAN_POINT('Ctrl Pts',(-206.457446264656,-97.0579274254718,
2.53934298880811));
#13308=CARTESIAN_POINT('Ctrl Pts',(-205.776789452019,-97.5399758727682,
2.59231242840954));
#13309=CARTESIAN_POINT('Ctrl Pts',(-204.833273127727,-97.6508642875058,
2.64528186801098));
#13310=CARTESIAN_POINT('Ctrl Pts',(-204.059399892623,-97.3397620309669,
2.69825130761241));
#13311=CARTESIAN_POINT('Ctrl Pts',(-203.28552665752,-97.028659774428,2.75122074721385));
#13312=CARTESIAN_POINT('Ctrl Pts',(-202.681296511605,-96.2955668466128,
2.80419018681529));
#13313=CARTESIAN_POINT('Ctrl Pts',(-202.523685181668,-95.4765289532145,
2.85715962641672));
#13314=CARTESIAN_POINT('Ctrl Pts',(-202.493675064825,-95.3205793594267,
2.86724531678049));
#13315=CARTESIAN_POINT('Ctrl Pts',(-202.479856837104,-95.1615138840336,
2.87733100714426));
#13316=CARTESIAN_POINT('Ctrl Pts',(-202.481315987002,-95.0021961802459,
2.88741669750803));
#13317=CARTESIAN_POINT('Ctrl Pts',(-202.486303966252,-95.0008035932749,
2.61258330249195));
#13318=CARTESIAN_POINT('Ctrl Pts',(-202.485244554665,-95.371508400945,2.58923323528426));
#13319=CARTESIAN_POINT('Ctrl Pts',(-202.561939805054,-95.7417961628412,
2.56588316807658));
#13320=CARTESIAN_POINT('Ctrl Pts',(-202.71859261042,-96.074427935554,2.54253310086889));
#13321=CARTESIAN_POINT('Ctrl Pts',(-203.073958239067,-96.8290004358175,
2.48956366126745));
#13322=CARTESIAN_POINT('Ctrl Pts',(-203.840789903126,-97.3897931164833,
2.43659422166602));
#13323=CARTESIAN_POINT('Ctrl Pts',(-204.667576276604,-97.4997418602453,
2.38362478206458));
#13324=CARTESIAN_POINT('Ctrl Pts',(-205.494362650082,-97.6096906040073,
2.33065534246314));
#13325=CARTESIAN_POINT('Ctrl Pts',(-206.38110373298,-97.2687954108656,2.27768590286171));
#13326=CARTESIAN_POINT('Ctrl Pts',(-206.921322319868,-96.6333204974726,
2.22471646326027));
#13327=CARTESIAN_POINT('Ctrl Pts',(-207.461540906757,-95.9978455840796,
2.17174702365884));
#13328=CARTESIAN_POINT('Ctrl Pts',(-207.655236997636,-95.0677909504354,
2.1187775840574));
#13329=CARTESIAN_POINT('Ctrl Pts',(-207.41362148715,-94.2694889285932,2.06580814445597));
#13330=CARTESIAN_POINT('Ctrl Pts',(-207.172005976663,-93.4711869067511,
2.01283870485453));
#13331=CARTESIAN_POINT('Ctrl Pts',(-206.495078864811,-92.8046374967111,
1.9598692652531));
#13332=CARTESIAN_POINT('Ctrl Pts',(-205.693139549457,-92.5753822193073,
1.90689982565166));
#13333=CARTESIAN_POINT('Ctrl Pts',(-204.891200234104,-92.3461269419034,
1.85393038605022));
#13334=CARTESIAN_POINT('Ctrl Pts',(-203.964248715248,-92.5541657971357,
1.80096094644879));
#13335=CARTESIAN_POINT('Ctrl Pts',(-203.337194817498,-93.1041370117052,
1.74799150684735));
#13336=CARTESIAN_POINT('Ctrl Pts',(-202.802872618589,-93.5727758795276,
1.70285543872889));
#13337=CARTESIAN_POINT('Ctrl Pts',(-202.48630621031,-94.2896919793449,1.65771937061042));
#13338=CARTESIAN_POINT('Ctrl Pts',(-202.480282573446,-95.0019224211138,
1.61258330249195));
#13339=CARTESIAN_POINT('Origin',(-205.,-95.,9.));
#13340=CARTESIAN_POINT('',(-202.480223490507,-94.9981350405341,0.612583302491955));
#13341=CARTESIAN_POINT('',(-202.485813979692,-94.9986458132734,0.887416697508031));
#13342=CARTESIAN_POINT('',(-202.4825,-95.,9.));
#13343=CARTESIAN_POINT('',(-206.913465996665,-93.3640127966251,0.));
#13344=CARTESIAN_POINT('Ctrl Pts',(-202.480223490507,-94.9981350405341,
0.612583302491955));
#13345=CARTESIAN_POINT('Ctrl Pts',(-202.486186751135,-95.7125466839347,
0.56729718713227));
#13346=CARTESIAN_POINT('Ctrl Pts',(-202.805062421801,-96.431520077419,0.522011071772584));
#13347=CARTESIAN_POINT('Ctrl Pts',(-203.34252319783,-96.9003741596628,0.476724956412899));
#13348=CARTESIAN_POINT('Ctrl Pts',(-203.971170541235,-97.4487748735251,
0.423755516811463));
#13349=CARTESIAN_POINT('Ctrl Pts',(-204.8988660792,-97.6549851699424,0.370786077210027));
#13350=CARTESIAN_POINT('Ctrl Pts',(-205.700052550654,-97.4230464763398,
0.317816637608592));
#13351=CARTESIAN_POINT('Ctrl Pts',(-206.501239022107,-97.1911077827372,
0.264847198007156));
#13352=CARTESIAN_POINT('Ctrl Pts',(-207.175916427048,-96.5210200991147,
0.21187775840572));
#13353=CARTESIAN_POINT('Ctrl Pts',(-207.41509417905,-95.7234547622828,0.158908318804285));
#13354=CARTESIAN_POINT('Ctrl Pts',(-207.654271931051,-94.9258894254509,
0.105938879202849));
#13355=CARTESIAN_POINT('Ctrl Pts',(-207.457950030113,-94.0008464354096,
0.052969439601414));
#13356=CARTESIAN_POINT('Ctrl Pts',(-206.913465996665,-93.3640127966251,
-2.14147317656561E-14));
#13357=CARTESIAN_POINT('',(-203.08284916835,-93.3612116138494,1.21293810816754E-15));
#13358=CARTESIAN_POINT('Origin',(-205.,-95.,0.));
#13359=CARTESIAN_POINT('Ctrl Pts',(-203.082846138209,-93.3612093103599,
7.63278329429795E-16));
#13360=CARTESIAN_POINT('Ctrl Pts',(-203.61481505219,-92.7406416726252,0.0519060689145028));
#13361=CARTESIAN_POINT('Ctrl Pts',(-204.477409065994,-92.4011123108223,
0.103812137829005));
#13362=CARTESIAN_POINT('Ctrl Pts',(-205.289479056896,-92.4950343384225,
0.155718206743507));
#13363=CARTESIAN_POINT('Ctrl Pts',(-206.118185472827,-92.5908804942238,
0.208687646344942));
#13364=CARTESIAN_POINT('Ctrl Pts',(-206.894276546249,-93.1381197102899,
0.261657085946378));
#13365=CARTESIAN_POINT('Ctrl Pts',(-207.262506848597,-93.886393298846,0.314626525547813));
#13366=CARTESIAN_POINT('Ctrl Pts',(-207.630737150946,-94.6346668874021,
0.367595965149249));
#13367=CARTESIAN_POINT('Ctrl Pts',(-207.591106682221,-95.5839748484483,
0.420565404750684));
#13368=CARTESIAN_POINT('Ctrl Pts',(-207.161534923276,-96.2989227744467,
0.47353484435212));
#13369=CARTESIAN_POINT('Ctrl Pts',(-206.73196316433,-97.0138707004452,0.526504283953556));
#13370=CARTESIAN_POINT('Ctrl Pts',(-205.912450115163,-97.4944585913958,
0.579473723554992));
#13371=CARTESIAN_POINT('Ctrl Pts',(-205.078775381405,-97.5205022929071,
0.632443163156427));
#13372=CARTESIAN_POINT('Ctrl Pts',(-204.245100647647,-97.5465459944184,
0.685412602757863));
#13373=CARTESIAN_POINT('Ctrl Pts',(-203.397264229298,-97.1180455064903,
0.738382042359298));
#13374=CARTESIAN_POINT('Ctrl Pts',(-202.92385184891,-96.4313676110377,0.791351481960734));
#13375=CARTESIAN_POINT('Ctrl Pts',(-202.637658761556,-96.0162486258607,
0.823373220476499));
#13376=CARTESIAN_POINT('Ctrl Pts',(-202.488302433328,-95.5067762975669,
0.855394958992265));
#13377=CARTESIAN_POINT('Ctrl Pts',(-202.485813979692,-94.9986458132734,
0.887416697508031));
#13378=CARTESIAN_POINT('Origin',(-205.,-95.,-2.20842344717744));
#13379=CARTESIAN_POINT('',(-201.921316222253,-94.9999604485794,16.2084234471775));
#13380=CARTESIAN_POINT('',(-201.931367503445,-94.9992219789103,16.2915765528226));
#13381=CARTESIAN_POINT('',(-201.9265,-94.9999999999997,-2.20842344717744));
#13382=CARTESIAN_POINT('',(-205.793799282533,-97.9692229537457,17.));
#13383=CARTESIAN_POINT('Ctrl Pts',(-201.931367503445,-94.9992219789103,
16.2915765528226));
#13384=CARTESIAN_POINT('Ctrl Pts',(-201.930437830903,-94.5288592028842,
16.315839943476));
#13385=CARTESIAN_POINT('Ctrl Pts',(-202.253352028229,-93.0329481124781,
16.3930727737308));
#13386=CARTESIAN_POINT('Ctrl Pts',(-204.582352673002,-91.390717466756,16.5232750435871));
#13387=CARTESIAN_POINT('Ctrl Pts',(-207.810248356741,-92.6929302430059,
16.6821833623914));
#13388=CARTESIAN_POINT('Ctrl Pts',(-208.456461600838,-96.1151764142335,
16.8410916811957));
#13389=CARTESIAN_POINT('Ctrl Pts',(-206.782006578242,-97.7050332130129,
16.9470305603986));
#13390=CARTESIAN_POINT('Ctrl Pts',(-205.793799282533,-97.9692229537457,
17.));
#13391=CARTESIAN_POINT('',(-204.206200717467,-97.9692229537457,17.));
#13392=CARTESIAN_POINT('Origin',(-205.,-95.,17.));
#13393=CARTESIAN_POINT('Ctrl Pts',(-201.921316222253,-94.9999604485793,
16.2084234471775));
#13394=CARTESIAN_POINT('Ctrl Pts',(-201.921316030809,-94.9985182315119,
16.2084984707981));
#13395=CARTESIAN_POINT('Ctrl Pts',(-201.921967711053,-93.9788178721187,
16.2615429340201));
#13396=CARTESIAN_POINT('Ctrl Pts',(-203.036133983161,-91.9425114866494,
16.3675568368436));
#13397=CARTESIAN_POINT('Ctrl Pts',(-206.506731020769,-91.6928976656653,
16.5264651556479));
#13398=CARTESIAN_POINT('Ctrl Pts',(-208.595808729299,-94.4759987242795,
16.6853734744522));
#13399=CARTESIAN_POINT('Ctrl Pts',(-207.396709451193,-97.716016535546,16.8432184225696));
#13400=CARTESIAN_POINT('Ctrl Pts',(-205.16879615822,-98.2310729989852,16.9480939310855));
#13401=CARTESIAN_POINT('Ctrl Pts',(-204.204429055805,-97.9745938792693,
17.));
#13402=CARTESIAN_POINT('Origin',(-205.,-95.,-2.20842344717744));
#13403=CARTESIAN_POINT('',(-201.928214488845,-94.9973269196036,15.2084234471775));
#13404=CARTESIAN_POINT('',(-201.926872790932,-95.0028204748396,15.2915765528226));
#13405=CARTESIAN_POINT('',(-201.9265,-94.9999999999997,-2.20842344717744));
#13406=CARTESIAN_POINT('Ctrl Pts',(-201.926872790932,-95.0028204748396,
15.2915765528226));
#13407=CARTESIAN_POINT('Ctrl Pts',(-201.933847540659,-94.2344924303963,
15.3313566392007));
#13408=CARTESIAN_POINT('Ctrl Pts',(-202.614657567475,-92.4320707201956,
15.4241061651802));
#13409=CARTESIAN_POINT('Ctrl Pts',(-205.641602982121,-91.4231516321926,
15.5698251307612));
#13410=CARTESIAN_POINT('Ctrl Pts',(-208.35434189336,-93.6020966294465,15.7287334495655));
#13411=CARTESIAN_POINT('Ctrl Pts',(-207.991790944675,-97.0626878467749,
15.8876417683698));
#13412=CARTESIAN_POINT('Ctrl Pts',(-204.886537405266,-98.6320975090182,
16.0465500871742));
#13413=CARTESIAN_POINT('Ctrl Pts',(-202.34331561747,-97.1406732810359,16.1811950153251));
#13414=CARTESIAN_POINT('Ctrl Pts',(-201.932467400235,-95.555708789217,16.2628705038745));
#13415=CARTESIAN_POINT('Ctrl Pts',(-201.931367503445,-94.9992219789103,
16.2915765528226));
#13416=CARTESIAN_POINT('Ctrl Pts',(-201.928214488845,-94.9973269196036,
15.2084234471775));
#13417=CARTESIAN_POINT('Ctrl Pts',(-201.925712567505,-94.6958484416858,
15.2240151665228));
#13418=CARTESIAN_POINT('Ctrl Pts',(-202.105035794616,-93.3730750516054,
15.2925763254696));
#13419=CARTESIAN_POINT('Ctrl Pts',(-204.001156151974,-91.5060233657571,
15.4141069240177));
#13420=CARTESIAN_POINT('Ctrl Pts',(-207.396173587353,-92.2679785768132,
15.5730152428221));
#13421=CARTESIAN_POINT('Ctrl Pts',(-208.594403743819,-95.5346307410897,
15.7319235616264));
#13422=CARTESIAN_POINT('Ctrl Pts',(-206.497329095757,-98.3111182304646,
15.8908318804307));
#13423=CARTESIAN_POINT('Ctrl Pts',(-203.02914899186,-98.0521756469229,16.0496651756144));
#13424=CARTESIAN_POINT('Ctrl Pts',(-201.921451197495,-96.0167766044663,
16.1555290311966));
#13425=CARTESIAN_POINT('Ctrl Pts',(-201.921316222253,-94.9999604485793,
16.2084234471775));
#13426=CARTESIAN_POINT('Origin',(-205.,-95.,-2.20842344717744));
#13427=CARTESIAN_POINT('',(-201.930806967845,-95.0014123568597,14.2084234471775));
#13428=CARTESIAN_POINT('',(-201.921581898641,-94.9991754600276,14.2915765528226));
#13429=CARTESIAN_POINT('',(-201.9265,-94.9999999999997,-2.20842344717744));
#13430=CARTESIAN_POINT('Ctrl Pts',(-201.921581898641,-94.9991754600276,
14.2915765528226));
#13431=CARTESIAN_POINT('Ctrl Pts',(-201.921422031341,-94.9544247205291,
14.293903895324));
#13432=CARTESIAN_POINT('Ctrl Pts',(-201.942596590982,-93.891318641259,14.3492006774268));
#13433=CARTESIAN_POINT('Ctrl Pts',(-203.167697451582,-91.8618096795541,
14.4574668991311));
#13434=CARTESIAN_POINT('Ctrl Pts',(-206.64568000845,-91.7600451831499,14.6163752179354));
#13435=CARTESIAN_POINT('Ctrl Pts',(-208.614921940056,-94.6286346539956,
14.7752835367397));
#13436=CARTESIAN_POINT('Ctrl Pts',(-207.270042986249,-97.8376885432202,
14.934191855544));
#13437=CARTESIAN_POINT('Ctrl Pts',(-203.844015760112,-98.4451795972611,
15.0931001743483));
#13438=CARTESIAN_POINT('Ctrl Pts',(-202.070126976119,-96.5327748382561,
15.2122284067745));
#13439=CARTESIAN_POINT('Ctrl Pts',(-201.924560266095,-95.2575647675798,
15.2783871995992));
#13440=CARTESIAN_POINT('Ctrl Pts',(-201.926872790932,-95.0028204748396,
15.2915765528226));
#13441=CARTESIAN_POINT('Ctrl Pts',(-201.930806967845,-95.0014123568597,
14.2084234471775));
#13442=CARTESIAN_POINT('Ctrl Pts',(-201.93330334053,-94.39862726836,14.2395318622475));
#13443=CARTESIAN_POINT('Ctrl Pts',(-202.396531719082,-92.765916828767,14.323609716919));
#13444=CARTESIAN_POINT('Ctrl Pts',(-205.050996758677,-91.3664108756636,
14.4606570111919));
#13445=CARTESIAN_POINT('Ctrl Pts',(-208.082134098584,-93.0748973262563,
14.6195653299962));
#13446=CARTESIAN_POINT('Ctrl Pts',(-208.287605318196,-96.548296522874,14.7784736488005));
#13447=CARTESIAN_POINT('Ctrl Pts',(-205.479036782975,-98.6022345010335,
14.9373819676048));
#13448=CARTESIAN_POINT('Ctrl Pts',(-202.549953768568,-97.4761895493396,
15.0806985670638));
#13449=CARTESIAN_POINT('Ctrl Pts',(-201.934212295366,-95.7200553090311,
15.1710457269214));
#13450=CARTESIAN_POINT('Ctrl Pts',(-201.928214488845,-94.9973269196036,
15.2084234471775));
#13451=CARTESIAN_POINT('Origin',(-205.,-95.,-2.20842344717744));
#13452=CARTESIAN_POINT('',(-201.923037944235,-95.0020215915549,13.2084234471775));
#13453=CARTESIAN_POINT('',(-201.929332692288,-94.9976509811143,13.2915765528226));
#13454=CARTESIAN_POINT('',(-201.9265,-94.9999999999997,-2.20842344717744));
#13455=CARTESIAN_POINT('Ctrl Pts',(-201.929332692288,-94.9976509811143,
13.2915765528226));
#13456=CARTESIAN_POINT('Ctrl Pts',(-201.926879286391,-94.6523048684722,
13.3094205910487));
#13457=CARTESIAN_POINT('Ctrl Pts',(-202.14011741618,-93.2847511636649,13.3802340688763));
#13458=CARTESIAN_POINT('Ctrl Pts',(-204.150349485118,-91.4667769681704,
13.5040169863052));
#13459=CARTESIAN_POINT('Ctrl Pts',(-207.509967453225,-92.3721426302753,
13.6629253051096));
#13460=CARTESIAN_POINT('Ctrl Pts',(-208.568475318891,-95.6866985528482,
13.8218336239139));
#13461=CARTESIAN_POINT('Ctrl Pts',(-206.355444885374,-98.3716969277542,
13.9807419427182));
#13462=CARTESIAN_POINT('Ctrl Pts',(-202.950369121919,-97.9715094124519,
14.1373229190211));
#13463=CARTESIAN_POINT('Ctrl Pts',(-201.925060550926,-95.9729347127417,
14.2409344557225));
#13464=CARTESIAN_POINT('Ctrl Pts',(-201.921581898641,-94.9991754600276,
14.2915765528226));
#13465=CARTESIAN_POINT('Ctrl Pts',(-201.923037944235,-95.0020215915549,
13.2084234471775));
#13466=CARTESIAN_POINT('Ctrl Pts',(-201.929861116958,-94.1043808714426,
13.2550485579722));
#13467=CARTESIAN_POINT('Ctrl Pts',(-202.817787000569,-92.1752061029806,
13.3546431083684));
#13468=CARTESIAN_POINT('Ctrl Pts',(-206.096505523284,-91.5354298452884,
13.5072070983661));
#13469=CARTESIAN_POINT('Ctrl Pts',(-208.506304586591,-94.045327873685,13.6661154171704));
#13470=CARTESIAN_POINT('Ctrl Pts',(-207.701562793806,-97.4304586389942,
13.8250237359747));
#13471=CARTESIAN_POINT('Ctrl Pts',(-204.420058427186,-98.5873720853337,
13.983932054779));
#13472=CARTESIAN_POINT('Ctrl Pts',(-202.208551898768,-96.8727802886784,
14.1117319585132));
#13473=CARTESIAN_POINT('Ctrl Pts',(-201.929052675175,-95.4250115526778,
14.1865624226461));
#13474=CARTESIAN_POINT('Ctrl Pts',(-201.930806967845,-95.0014123568597,
14.2084234471775));
#13475=CARTESIAN_POINT('Origin',(-205.,-95.,-2.20842344717744));
#13476=CARTESIAN_POINT('',(-201.924530264077,-94.9974318186093,12.2084234471775));
#13477=CARTESIAN_POINT('',(-201.930073780141,-95.0019865806918,12.2915765528226));
#13478=CARTESIAN_POINT('',(-201.9265,-94.9999999999997,-2.20842344717744));
#13479=CARTESIAN_POINT('Ctrl Pts',(-201.930073780141,-95.0019865806918,
12.2915765528226));
#13480=CARTESIAN_POINT('Ctrl Pts',(-201.933893603562,-94.3559450496333,
12.3249372867734));
#13481=CARTESIAN_POINT('Ctrl Pts',(-202.4491356456,-92.6785603743455,12.4112674603257));
#13482=CARTESIAN_POINT('Ctrl Pts',(-205.205169266307,-91.3718494299793,
12.5505670734794));
#13483=CARTESIAN_POINT('Ctrl Pts',(-208.161062939416,-93.2074453761791,
12.7094753922837));
#13484=CARTESIAN_POINT('Ctrl Pts',(-208.218929440283,-96.6864353664204,
12.868383711088));
#13485=CARTESIAN_POINT('Ctrl Pts',(-205.325717407468,-98.6193202618013,
13.0272920298923));
#13486=CARTESIAN_POINT('Ctrl Pts',(-202.49230593161,-97.3896064222378,13.1683563104705));
#13487=CARTESIAN_POINT('Ctrl Pts',(-201.93416214097,-95.6774534264036,13.2564511514473));
#13488=CARTESIAN_POINT('Ctrl Pts',(-201.929332692288,-94.9976509811143,
13.2915765528226));
#13489=CARTESIAN_POINT('Ctrl Pts',(-201.924530264077,-94.9974318186092,
12.2084234471775));
#13490=CARTESIAN_POINT('Ctrl Pts',(-201.922946574968,-94.8206195588585,
12.2175958140955));
#13491=CARTESIAN_POINT('Ctrl Pts',(-202.017340558395,-93.6244254438343,
12.279737620615));
#13492=CARTESIAN_POINT('Ctrl Pts',(-203.58671258731,-91.6521365902563,12.3948488667359));
#13493=CARTESIAN_POINT('Ctrl Pts',(-207.048879196816,-91.9987228122024,
12.5537571855402));
#13494=CARTESIAN_POINT('Ctrl Pts',(-208.632656258583,-95.0968464152565,
12.7126655043445));
#13495=CARTESIAN_POINT('Ctrl Pts',(-206.886054663924,-98.1061823072572,
12.8715738231488));
#13496=CARTESIAN_POINT('Ctrl Pts',(-203.410339233432,-98.2678049770775,
13.0304821419532));
#13497=CARTESIAN_POINT('Ctrl Pts',(-201.984203605419,-96.2651388949014,
13.1427653499627));
#13498=CARTESIAN_POINT('Ctrl Pts',(-201.922109507808,-95.1241645265866,
13.2020791183708));
#13499=CARTESIAN_POINT('Ctrl Pts',(-201.923037944235,-95.0020215915549,
13.2084234471775));
#13500=CARTESIAN_POINT('Origin',(-205.,-95.,-2.20842344717744));
#13501=CARTESIAN_POINT('',(-201.93133959706,-94.9994302440671,11.2084234471775));
#13502=CARTESIAN_POINT('',(-201.922093677493,-95.0013994409948,11.2915765528226));
#13503=CARTESIAN_POINT('',(-201.9265,-94.9999999999997,-2.20842344717744));
#13504=CARTESIAN_POINT('Ctrl Pts',(-201.922093677493,-95.0013994409948,
11.2915765528226));
#13505=CARTESIAN_POINT('Ctrl Pts',(-201.927419125191,-94.061156157063,11.3404539824981));
#13506=CARTESIAN_POINT('Ctrl Pts',(-202.890883202837,-92.0925151635822,
11.4423008517751));
#13507=CARTESIAN_POINT('Ctrl Pts',(-206.242562362063,-91.5850900798271,
11.5971171606536));
#13508=CARTESIAN_POINT('Ctrl Pts',(-208.54366376786,-94.1950042938844,11.7560254794579));
#13509=CARTESIAN_POINT('Ctrl Pts',(-207.595973838081,-97.542929574037,11.9149337982622));
#13510=CARTESIAN_POINT('Ctrl Pts',(-204.26832410821,-98.5595254425124,12.0738421170665));
#13511=CARTESIAN_POINT('Ctrl Pts',(-202.16923931098,-96.7844614271993,12.19938970192));
#13512=CARTESIAN_POINT('Ctrl Pts',(-201.927828571951,-95.3817155830347,
12.271967847172));
#13513=CARTESIAN_POINT('Ctrl Pts',(-201.930073780141,-95.0019865806918,
12.2915765528226));
#13514=CARTESIAN_POINT('Ctrl Pts',(-201.93133959706,-94.9994302440671,11.2084234471775));
#13515=CARTESIAN_POINT('Ctrl Pts',(-201.930548213561,-94.5208250022373,
11.2331125098202));
#13516=CARTESIAN_POINT('Ctrl Pts',(-202.261412933308,-93.0164261928261,
11.3107710120644));
#13517=CARTESIAN_POINT('Ctrl Pts',(-204.612024659808,-91.3868233012261,
11.4413989539101));
#13518=CARTESIAN_POINT('Ctrl Pts',(-207.827224979576,-92.7169385387114,
11.6003072727144));
#13519=CARTESIAN_POINT('Ctrl Pts',(-208.450457037378,-96.1401390066001,
11.7592155915187));
#13520=CARTESIAN_POINT('Ctrl Pts',(-205.910348648356,-98.5180727763361,
11.918123910323));
#13521=CARTESIAN_POINT('Ctrl Pts',(-202.730434611476,-97.7195893976379,
12.0678598622093));
#13522=CARTESIAN_POINT('Ctrl Pts',(-201.932092210478,-95.8416914803529,
12.1646263744941));
#13523=CARTESIAN_POINT('Ctrl Pts',(-201.924530264077,-94.9974318186092,
12.2084234471775));
#13524=CARTESIAN_POINT('Origin',(-205.,-95.,-2.20842344717744));
#13525=CARTESIAN_POINT('',(-201.926625204813,-95.0028238958017,10.2084234471775));
#13526=CARTESIAN_POINT('',(-201.925838838714,-94.9972120666634,10.2915765528226));
#13527=CARTESIAN_POINT('',(-201.9265,-94.9999999999997,-2.20842344717744));
#13528=CARTESIAN_POINT('Ctrl Pts',(-201.925838838714,-94.9972120666634,
10.2915765528226));
#13529=CARTESIAN_POINT('Ctrl Pts',(-201.923796651544,-94.7767411547191,
10.3030012386214));
#13530=CARTESIAN_POINT('Ctrl Pts',(-202.046093670253,-93.536326186288,10.3673953640217));
#13531=CARTESIAN_POINT('Ctrl Pts',(-203.730077621707,-91.5951698809454,
10.4847589290234));
#13532=CARTESIAN_POINT('Ctrl Pts',(-207.174414580991,-92.0883866643241,
10.6436672478277));
#13533=CARTESIAN_POINT('Ctrl Pts',(-208.625272555405,-95.2509380113502,
10.802575566632));
#13534=CARTESIAN_POINT('Ctrl Pts',(-206.752521169945,-98.1834321942526,
10.9614838854363));
#13535=CARTESIAN_POINT('Ctrl Pts',(-203.273077963447,-98.1973913220278,
11.1203922042406));
#13536=CARTESIAN_POINT('Ctrl Pts',(-201.960101924826,-96.1773510717403,
11.2304230933694));
#13537=CARTESIAN_POINT('Ctrl Pts',(-201.921647831937,-95.0801164454715,
11.2874845428967));
#13538=CARTESIAN_POINT('Ctrl Pts',(-201.922093677493,-95.0013994409948,
11.2915765528226));
#13539=CARTESIAN_POINT('Ctrl Pts',(-201.926625204813,-95.0028238958017,
10.2084234471775));
#13540=CARTESIAN_POINT('Ctrl Pts',(-201.93373191466,-94.2264345369936,10.248629205545));
#13541=CARTESIAN_POINT('Ctrl Pts',(-202.626469630616,-92.4158935511655,
10.3418044035139));
#13542=CARTESIAN_POINT('Ctrl Pts',(-205.670290617637,-91.4284063488314,
10.4879490410842));
#13543=CARTESIAN_POINT('Ctrl Pts',(-208.365431665519,-93.6290731507911,
10.6468573598885));
#13544=CARTESIAN_POINT('Ctrl Pts',(-207.975182577187,-97.0865903655397,
10.8057656786929));
#13545=CARTESIAN_POINT('Ctrl Pts',(-204.85731935509,-98.6311448545504,10.9646739974972));
#13546=CARTESIAN_POINT('Ctrl Pts',(-202.334353092009,-97.1239486684601,
11.0988932536587));
#13547=CARTESIAN_POINT('Ctrl Pts',(-201.932246096589,-95.5476542430574,
11.1801430702188));
#13548=CARTESIAN_POINT('Ctrl Pts',(-201.93133959706,-94.9994302440671,11.2084234471775));
#13549=CARTESIAN_POINT('Origin',(-205.,-95.,-2.20842344717744));
#13550=CARTESIAN_POINT('',(-201.921683699254,-94.9990313104991,9.20842344717747));
#13551=CARTESIAN_POINT('',(-201.931429552667,-95.000145803808,9.29157655282255));
#13552=CARTESIAN_POINT('',(-201.9265,-94.9999999999997,-2.20842344717744));
#13553=CARTESIAN_POINT('Ctrl Pts',(-201.931429552667,-95.000145803808,9.29157655282255));
#13554=CARTESIAN_POINT('Ctrl Pts',(-201.931650187457,-94.4778404498504,
9.31851793434612));
#13555=CARTESIAN_POINT('Ctrl Pts',(-202.306382510376,-92.9283336853723,
9.39842875547113));
#13556=CARTESIAN_POINT('Ctrl Pts',(-204.765726357252,-91.3736124246263,
9.53130901619759));
#13557=CARTESIAN_POINT('Ctrl Pts',(-207.921576173118,-92.8389901316329,
9.69021733500189));
#13558=CARTESIAN_POINT('Ctrl Pts',(-208.398957607323,-96.2855575327979,
9.84912565380619));
#13559=CARTESIAN_POINT('Ctrl Pts',(-205.76021269658,-98.5535401563045,10.0080339726105));
#13560=CARTESIAN_POINT('Ctrl Pts',(-202.664332808566,-97.6348429287674,
10.155517605616));
#13561=CARTESIAN_POINT('Ctrl Pts',(-201.933265052849,-95.798932999617,10.25003179902));
#13562=CARTESIAN_POINT('Ctrl Pts',(-201.925838838714,-94.9972120666634,
10.2915765528226));
#13563=CARTESIAN_POINT('Ctrl Pts',(-201.921683699254,-94.9990313104991,
9.20842344717747));
#13564=CARTESIAN_POINT('Ctrl Pts',(-201.921465341112,-94.9460909713989,
9.21117646166824));
#13565=CARTESIAN_POINT('Ctrl Pts',(-201.946710084923,-93.8747633774113,
9.26689891576045));
#13566=CARTESIAN_POINT('Ctrl Pts',(-203.192936111301,-91.8472090422419,
9.3755908094541));
#13567=CARTESIAN_POINT('Ctrl Pts',(-206.671623368988,-91.7733537483301,
9.53449912825839));
#13568=CARTESIAN_POINT('Ctrl Pts',(-208.617785005374,-94.6576516743914,
9.69340744706271));
#13569=CARTESIAN_POINT('Ctrl Pts',(-207.247201784069,-97.8558107190141,
9.85231576586701));
#13570=CARTESIAN_POINT('Ctrl Pts',(-203.816409083639,-98.4357944152506,
10.0112240846713));
#13571=CARTESIAN_POINT('Ctrl Pts',(-202.064207659429,-96.5161000870413,
10.1299266451081));
#13572=CARTESIAN_POINT('Ctrl Pts',(-201.924369115566,-95.2492957120694,
10.1956597659435));
#13573=CARTESIAN_POINT('Ctrl Pts',(-201.926625204813,-95.0028238958017,
10.2084234471775));
#13574=CARTESIAN_POINT('Origin',(-205.,-95.,-2.20842344717744));
#13575=CARTESIAN_POINT('',(-201.929523551853,-94.9977303344825,8.20842344717746));
#13576=CARTESIAN_POINT('',(-201.925302479416,-95.0027227980173,8.29157655282255));
#13577=CARTESIAN_POINT('',(-201.9265,-94.9999999999997,-2.20842344717744));
#13578=CARTESIAN_POINT('Ctrl Pts',(-201.925302479416,-95.0027227980173,
8.29157655282255));
#13579=CARTESIAN_POINT('Ctrl Pts',(-201.93285017436,-94.1837439219852,8.33403463007085));
#13580=CARTESIAN_POINT('Ctrl Pts',(-202.690770472001,-92.3306976061766,
8.42946214692058));
#13581=CARTESIAN_POINT('Ctrl Pts',(-205.821273849133,-91.4600734116028,
8.57785910337174));
#13582=CARTESIAN_POINT('Ctrl Pts',(-208.420584658025,-93.7731456550212,
8.73676742217605));
#13583=CARTESIAN_POINT('Ctrl Pts',(-207.883941683608,-97.2109842496187,
8.89567574098036));
#13584=CARTESIAN_POINT('Ctrl Pts',(-204.703333206878,-98.6218171958797,
9.05458405978466));
#13585=CARTESIAN_POINT('Ctrl Pts',(-202.287835459144,-97.0359644386318,
9.1865509970654));
#13586=CARTESIAN_POINT('Ctrl Pts',(-201.931216397484,-95.5047448005331,
9.26554849474469));
#13587=CARTESIAN_POINT('Ctrl Pts',(-201.931429552667,-95.000145803808,9.29157655282255));
#13588=CARTESIAN_POINT('Ctrl Pts',(-201.929523551853,-94.9977303344825,
8.20842344717746));
#13589=CARTESIAN_POINT('Ctrl Pts',(-201.927106317664,-94.6440906524844,
8.22669315739296));
#13590=CARTESIAN_POINT('Ctrl Pts',(-202.147009202964,-93.2680558099108,
8.29793230720989));
#13591=CARTESIAN_POINT('Ctrl Pts',(-204.178726159118,-91.4600734471682,
8.42214089662825));
#13592=CARTESIAN_POINT('Ctrl Pts',(-207.530971620008,-92.3923663255981,
8.58104921543255));
#13593=CARTESIAN_POINT('Ctrl Pts',(-208.562850587821,-95.7153086117373,
8.73995753423687));
#13594=CARTESIAN_POINT('Ctrl Pts',(-206.328347957964,-98.382463957492,8.89886585304117));
#13595=CARTESIAN_POINT('Ctrl Pts',(-202.935840595157,-97.9561304030613,
9.05502115735471));
#13596=CARTESIAN_POINT('Ctrl Pts',(-201.925666666051,-95.9646908021815,
9.1582070220668));
#13597=CARTESIAN_POINT('Ctrl Pts',(-201.921683699254,-94.9990313104991,
9.20842344717747));
#13598=CARTESIAN_POINT('Origin',(-205.,-95.,-2.20842344717744));
#13599=CARTESIAN_POINT('',(-201.929907480782,-95.0020818313008,7.20842344717746));
#13600=CARTESIAN_POINT('',(-201.922442534737,-94.9983308996675,7.29157655282255));
#13601=CARTESIAN_POINT('',(-201.9265,-94.9999999999997,-2.20842344717744));
#13602=CARTESIAN_POINT('Ctrl Pts',(-201.922442534737,-94.9983308996675,
7.29157655282255));
#13603=CARTESIAN_POINT('Ctrl Pts',(-201.921812073097,-94.902015678895,7.29658188619413));
#13604=CARTESIAN_POINT('Ctrl Pts',(-201.969634830997,-93.7870693467852,
7.35455665916715));
#13605=CARTESIAN_POINT('Ctrl Pts',(-203.328376614218,-91.7733537159122,
7.46550087174159));
#13606=CARTESIAN_POINT('Ctrl Pts',(-206.807063906854,-91.847209010566,7.62440919054591));
#13607=CARTESIAN_POINT('Ctrl Pts',(-208.629055206866,-94.8115078462396,
7.7833175093502));
#13608=CARTESIAN_POINT('Ctrl Pts',(-207.123969254423,-97.9486141817431,
7.94222582815452));
#13609=CARTESIAN_POINT('Ctrl Pts',(-203.67165202869,-98.3824639914755,8.10113414695881));
#13610=CARTESIAN_POINT('Ctrl Pts',(-202.034177190516,-96.4279351805356,
8.21758438851483));
#13611=CARTESIAN_POINT('Ctrl Pts',(-201.923433893705,-95.2054777102381,
8.28106519046941));
#13612=CARTESIAN_POINT('Ctrl Pts',(-201.925302479416,-95.0027227980173,
8.29157655282255));
#13613=CARTESIAN_POINT('Ctrl Pts',(-201.929907480782,-95.0020818313008,
7.20842344717746));
#13614=CARTESIAN_POINT('Ctrl Pts',(-201.933975214882,-94.3478859808551,
7.24220985311768));
#13615=CARTESIAN_POINT('Ctrl Pts',(-202.459390523649,-92.662093249463,7.32896569865933));
#13616=CARTESIAN_POINT('Ctrl Pts',(-205.234273640395,-91.3736124610605,
7.46869098380241));
#13617=CARTESIAN_POINT('Ctrl Pts',(-208.175343969469,-93.2328663330924,
7.62759930260672));
#13618=CARTESIAN_POINT('Ctrl Pts',(-208.205294437497,-96.7122086000577,
7.78650762141102));
#13619=CARTESIAN_POINT('Ctrl Pts',(-205.296666790141,-98.6218171594914,
7.94541594021533));
#13620=CARTESIAN_POINT('Ctrl Pts',(-202.481733314634,-97.3731878742982,
8.08605454880414));
#13621=CARTESIAN_POINT('Ctrl Pts',(-201.934114613849,-95.6693995137262,
8.17372371779152));
#13622=CARTESIAN_POINT('Ctrl Pts',(-201.929523551853,-94.9977303344825,
8.20842344717746));
#13623=CARTESIAN_POINT('Origin',(-205.,-95.,-2.20842344717744));
#13624=CARTESIAN_POINT('',(-201.921949435201,-95.0012666709355,6.20842344717746));
#13625=CARTESIAN_POINT('',(-201.930401808297,-94.9982329210887,6.29157655282255));
#13626=CARTESIAN_POINT('',(-201.9265,-94.9999999999997,-2.20842344717744));
#13627=CARTESIAN_POINT('Ctrl Pts',(-201.930401808297,-94.9982329210887,
6.29157655282255));
#13628=CARTESIAN_POINT('Ctrl Pts',(-201.928325217551,-94.6007106472249,
6.31209858191885));
#13629=CARTESIAN_POINT('Ctrl Pts',(-202.184887815006,-93.1797200737991,
6.38559005061659));
#13630=CARTESIAN_POINT('Ctrl Pts',(-204.329709375628,-91.4284063129477,
6.51205095891576));
#13631=CARTESIAN_POINT('Ctrl Pts',(-207.639365403312,-92.5021366622034,
6.67095927772007));
#13632=CARTESIAN_POINT('Ctrl Pts',(-208.529280728881,-95.8658802014486,
6.82986759652437));
#13633=CARTESIAN_POINT('Ctrl Pts',(-206.183590928253,-98.4357944497699,
6.98877591532868));
#13634=CARTESIAN_POINT('Ctrl Pts',(-202.860862148067,-97.8740792172285,
7.1426789007614));
#13635=CARTESIAN_POINT('Ctrl Pts',(-201.928483996284,-95.9212811085216,
7.2436124465927));
#13636=CARTESIAN_POINT('Ctrl Pts',(-201.922442534737,-94.9983308996675,
7.29157655282255));
#13637=CARTESIAN_POINT('Ctrl Pts',(-201.921949435201,-95.0012666709355,
6.20842344717746));
#13638=CARTESIAN_POINT('Ctrl Pts',(-201.926887034891,-94.0529526670259,
6.2577265488424));
#13639=CARTESIAN_POINT('Ctrl Pts',(-202.905053295201,-92.0770071799099,
6.35999909010877));
#13640=CARTESIAN_POINT('Ctrl Pts',(-206.269922365534,-91.5951699151535,
6.51524107097657));
#13641=CARTESIAN_POINT('Ctrl Pts',(-208.550008659151,-94.2234633034355,
6.67414938978088));
#13642=CARTESIAN_POINT('Ctrl Pts',(-207.575486691771,-97.5636768559377,
6.83305770858518));
#13643=CARTESIAN_POINT('Ctrl Pts',(-204.239787311058,-98.5535401206023,
6.9919660273895));
#13644=CARTESIAN_POINT('Ctrl Pts',(-202.162081059052,-96.7677662638285,
7.11708794025358));
#13645=CARTESIAN_POINT('Ctrl Pts',(-201.927597928226,-95.3735170482439,
7.18924041351624));
#13646=CARTESIAN_POINT('Ctrl Pts',(-201.929907480782,-95.0020818313008,
7.20842344717746));
#13647=CARTESIAN_POINT('Origin',(-205.,-95.,-2.20842344717744));
#13648=CARTESIAN_POINT('',(-201.926089504652,-94.997192970312,5.20842344717746));
#13649=CARTESIAN_POINT('',(-201.928899855331,-95.0025004707799,5.29157655282255));
#13650=CARTESIAN_POINT('',(-201.9265,-94.9999999999997,-2.20842344717744));
#13651=CARTESIAN_POINT('Ctrl Pts',(-201.928899855331,-95.0025004707799,
5.29157655282255));
#13652=CARTESIAN_POINT('Ctrl Pts',(-201.934224625714,-94.3052696210272,
5.32761527764357));
#13653=CARTESIAN_POINT('Ctrl Pts',(-202.515335032503,-92.5752228264589,
5.41662344206603));
#13654=CARTESIAN_POINT('Ctrl Pts',(-205.38797534409,-91.3868232649246,5.55860104608991));
#13655=CARTESIAN_POINT('Ctrl Pts',(-208.247484237019,-93.3692280610634,
5.71750936489423));
#13656=CARTESIAN_POINT('Ctrl Pts',(-208.129735877909,-96.8467063440184,
5.87641768369853));
#13657=CARTESIAN_POINT('Ctrl Pts',(-205.142680646343,-98.6311448910324,
6.03532600250284));
#13658=CARTESIAN_POINT('Ctrl Pts',(-202.427470198555,-97.2860600726802,
6.17371229221084));
#13659=CARTESIAN_POINT('Ctrl Pts',(-201.933685108993,-95.6267559752403,
6.25912914231742));
#13660=CARTESIAN_POINT('Ctrl Pts',(-201.930401808297,-94.9982329210887,
6.29157655282255));
#13661=CARTESIAN_POINT('Ctrl Pts',(-201.926089504652,-94.997192970312,5.20842344717746));
#13662=CARTESIAN_POINT('Ctrl Pts',(-201.9239736235,-94.7684597513135,5.22027380496568));
#13663=CARTESIAN_POINT('Ctrl Pts',(-202.051768758167,-93.5196634776365,
5.28509360235533));
#13664=CARTESIAN_POINT('Ctrl Pts',(-203.75743765042,-91.5850901141365,5.40288283934643));
#13665=CARTESIAN_POINT('Ctrl Pts',(-207.19770630733,-92.1059271419192,5.56179115815073));
#13666=CARTESIAN_POINT('Ctrl Pts',(-208.623142384989,-95.2800178195362,
5.72069947695504));
#13667=CARTESIAN_POINT('Ctrl Pts',(-206.726922019203,-98.1973912899037,
5.87960779575934));
#13668=CARTESIAN_POINT('Ctrl Pts',(-203.247478847662,-98.1834321622689,
6.03851611456366));
#13669=CARTESIAN_POINT('Ctrl Pts',(-201.955769755693,-96.1607774588135,
6.14812133170303));
#13670=CARTESIAN_POINT('Ctrl Pts',(-201.921582259335,-95.0717863642375,
6.20475710924096));
#13671=CARTESIAN_POINT('Ctrl Pts',(-201.921949435201,-95.0012666709355,
6.20842344717746));
#13672=CARTESIAN_POINT('Origin',(-205.,-95.,-2.20842344717744));
#13673=CARTESIAN_POINT('',(-201.931412543801,-95.0002813817275,4.20842344717746));
#13674=CARTESIAN_POINT('',(-201.921415568031,-95.0005065249549,4.29157655282255));
#13675=CARTESIAN_POINT('',(-201.9265,-94.9999999999997,-2.20842344717744));
#13676=CARTESIAN_POINT('Ctrl Pts',(-201.921415568031,-95.0005065249549,
4.29157655282255));
#13677=CARTESIAN_POINT('Ctrl Pts',(-201.923678444759,-94.0093290712259,
4.34313197336829));
#13678=CARTESIAN_POINT('Ctrl Pts',(-202.981928292525,-91.9956387425796,
4.44765683351546));
#13679=CARTESIAN_POINT('Ctrl Pts',(-206.413287426889,-91.6521365566204,
4.60515113326408));
#13680=CARTESIAN_POINT('Ctrl Pts',(-208.57976795423,-94.3748341177099,4.76405945206838));
#13681=CARTESIAN_POINT('Ctrl Pts',(-207.464357231459,-97.6706767723307,
4.92296777087269));
#13682=CARTESIAN_POINT('Ctrl Pts',(-204.089651342497,-98.5180728116819,
5.081876089677));
#13683=CARTESIAN_POINT('Ctrl Pts',(-202.125612631896,-96.6794292344261,
5.20474568366028));
#13684=CARTESIAN_POINT('Ctrl Pts',(-201.926398319301,-95.3300541428894,
5.27464583804213));
#13685=CARTESIAN_POINT('Ctrl Pts',(-201.928899855331,-95.0025004707799,
5.29157655282255));
#13686=CARTESIAN_POINT('Ctrl Pts',(-201.931412543801,-95.0002813817275,
4.20842344717746));
#13687=CARTESIAN_POINT('Ctrl Pts',(-201.931845200035,-94.4697309905534,
4.2357905006904));
#13688=CARTESIAN_POINT('Ctrl Pts',(-202.315173521402,-92.9117048313377,
4.31612699380478));
#13689=CARTESIAN_POINT('Ctrl Pts',(-204.794830735755,-91.3718494664313,
4.44943292652058));
#13690=CARTESIAN_POINT('Ctrl Pts',(-207.938821267524,-92.8625013967925,
4.60834124532489));
#13691=CARTESIAN_POINT('Ctrl Pts',(-208.38853330781,-96.3127881561792,4.7672495641292));
#13692=CARTESIAN_POINT('Ctrl Pts',(-205.731675884439,-98.55952540675,4.92615788293351));
#13693=CARTESIAN_POINT('Ctrl Pts',(-202.652180845941,-97.6187407126683,
5.07321584394959));
#13694=CARTESIAN_POINT('Ctrl Pts',(-201.933431315907,-95.790865204812,5.16730436536424));
#13695=CARTESIAN_POINT('Ctrl Pts',(-201.926089504652,-94.997192970312,5.20842344717746));
#13696=CARTESIAN_POINT('Origin',(-205.,-95.,-2.20842344717744));
#13697=CARTESIAN_POINT('',(-201.92505449297,-95.0026812154856,3.20842344717746));
#13698=CARTESIAN_POINT('',(-201.927395781804,-94.9972100788545,3.29157655282255));
#13699=CARTESIAN_POINT('',(-201.9265,-94.9999999999997,-2.20842344717744));
#13700=CARTESIAN_POINT('Ctrl Pts',(-201.927395781804,-94.9972100788545,
3.29157655282255));
#13701=CARTESIAN_POINT('Ctrl Pts',(-201.924984715586,-94.7247076994421,
3.30567922949157));
#13702=CARTESIAN_POINT('Ctrl Pts',(-202.083098692961,-93.431441735486,3.37275134576203));
#13703=CARTESIAN_POINT('Ctrl Pts',(-203.9034944657,-91.5354298104801,3.49279290163393));
#13704=CARTESIAN_POINT('Ctrl Pts',(-207.318557571481,-92.2018109830213,
3.65170122043824));
#13705=CARTESIAN_POINT('Ctrl Pts',(-208.607993009848,-95.4335405719414,
3.81060953924254));
#13706=CARTESIAN_POINT('Ctrl Pts',(-206.589660782539,-98.2678050099089,
3.96951785804685));
#13707=CARTESIAN_POINT('Ctrl Pts',(-203.113945317127,-98.1061823384649,
4.12842617685115));
#13708=CARTESIAN_POINT('Ctrl Pts',(-201.934002400455,-96.0731803187063,
4.23577907510972));
#13709=CARTESIAN_POINT('Ctrl Pts',(-201.921353503737,-95.0276917130945,
4.29016253376686));
#13710=CARTESIAN_POINT('Ctrl Pts',(-201.921415568031,-95.0005065249549,
4.29157655282255));
#13711=CARTESIAN_POINT('Ctrl Pts',(-201.92505449297,-95.0026812154857,3.20842344717746));
#13712=CARTESIAN_POINT('Ctrl Pts',(-201.932628937064,-94.1756633460531,
3.25130719641512));
#13713=CARTESIAN_POINT('Ctrl Pts',(-202.703262857742,-92.3146803557045,
3.34716038525422));
#13714=CARTESIAN_POINT('Ctrl Pts',(-205.849650506345,-91.4667770036684,
3.49598301369474));
#13715=CARTESIAN_POINT('Ctrl Pts',(-208.430318355407,-93.8006307060494,
3.65489133249905));
#13716=CARTESIAN_POINT('Ctrl Pts',(-207.866108674953,-97.2340527708336,
3.81379965130336));
#13717=CARTESIAN_POINT('Ctrl Pts',(-204.674282595805,-98.6193202254382,
3.97270797010767));
#13718=CARTESIAN_POINT('Ctrl Pts',(-202.279337066252,-97.0193151145692,
4.10424923539903));
#13719=CARTESIAN_POINT('Ctrl Pts',(-201.931007785871,-95.4966211118274,
4.18282106108896));
#13720=CARTESIAN_POINT('Ctrl Pts',(-201.931412543801,-95.0002813817275,
4.20842344717746));
#13721=CARTESIAN_POINT('Origin',(-205.,-95.,-2.20842344717744));
#13722=CARTESIAN_POINT('',(-201.922621816358,-94.9982129686146,2.20842344717746));
#13723=CARTESIAN_POINT('',(-201.931144087497,-95.0009810700816,2.29157655282255));
#13724=CARTESIAN_POINT('',(-201.9265,-94.9999999999997,-2.20842344717744));
#13725=CARTESIAN_POINT('Ctrl Pts',(-201.931144087497,-95.0009810700815,
2.29157655282255));
#13726=CARTESIAN_POINT('Ctrl Pts',(-201.93278473837,-94.4268914775859,2.32119592521629));
#13727=CARTESIAN_POINT('Ctrl Pts',(-202.363262699554,-92.8238514576806,
2.40378473721147));
#13728=CARTESIAN_POINT('Ctrl Pts',(-204.94900324081,-91.3664108391532,2.53934298880809));
#13729=CARTESIAN_POINT('Ctrl Pts',(-208.026893856913,-92.9891582387231,
2.6982513076124));
#13730=CARTESIAN_POINT('Ctrl Pts',(-208.329762022302,-96.4554229209582,
2.8571596264167));
#13731=CARTESIAN_POINT('Ctrl Pts',(-205.579941578641,-98.5873721213763,
3.01606794522101));
#13732=CARTESIAN_POINT('Ctrl Pts',(-202.589661678081,-97.5331315540107,
3.16087358735629));
#13733=CARTESIAN_POINT('Ctrl Pts',(-201.934040643722,-95.748222502078,3.25270978989014));
#13734=CARTESIAN_POINT('Ctrl Pts',(-201.927395781804,-94.9972100788545,
3.29157655282255));
#13735=CARTESIAN_POINT('Ctrl Pts',(-201.922621816358,-94.9982129686145,
2.20842344717746));
#13736=CARTESIAN_POINT('Ctrl Pts',(-201.921899400381,-94.8936907064347,
2.2138544525384));
#13737=CARTESIAN_POINT('Ctrl Pts',(-201.974189338711,-93.7704778816497,
2.27225489750078));
#13738=CARTESIAN_POINT('Ctrl Pts',(-203.3543200081,-91.7600452157265,2.3836247820646));
#13739=CARTESIAN_POINT('Ctrl Pts',(-206.83230253,-91.8618097110707,2.5425331008689));
#13740=CARTESIAN_POINT('Ctrl Pts',(-208.630450771479,-94.8406321802388,
2.70144141967321));
#13741=CARTESIAN_POINT('Ctrl Pts',(-207.100242225817,-97.9655611925551,
2.86034973847752));
#13742=CARTESIAN_POINT('Ctrl Pts',(-203.644555128245,-98.3716968938806,
3.01925805728183));
#13743=CARTESIAN_POINT('Ctrl Pts',(-202.028743553123,-96.4112848780084,
3.13528262684847));
#13744=CARTESIAN_POINT('Ctrl Pts',(-201.923273083948,-95.1971848749064,
3.19833775681368));
#13745=CARTESIAN_POINT('Ctrl Pts',(-201.92505449297,-95.0026812154857,3.20842344717746));
#13746=CARTESIAN_POINT('Origin',(-205.,-95.,-2.20842344717744));
#13747=CARTESIAN_POINT('',(-201.930545885435,-94.9983467356882,1.20842344717746));
#13748=CARTESIAN_POINT('',(-201.923792845874,-95.0023469955484,1.29157655282255));
#13749=CARTESIAN_POINT('',(-201.9265,-94.9999999999997,-2.20842344717744));
#13750=CARTESIAN_POINT('Ctrl Pts',(-201.923792845874,-95.0023469955484,
1.29157655282255));
#13751=CARTESIAN_POINT('Ctrl Pts',(-201.931146827165,-94.1328175962329,
1.33671262094101));
#13752=CARTESIAN_POINT('Ctrl Pts',(-202.771183473608,-92.2304180348085,
1.43481812866091));
#13753=CARTESIAN_POINT('Ctrl Pts',(-205.99884385808,-91.5060233304403,1.58589307598225));
#13754=CARTESIAN_POINT('Ctrl Pts',(-208.478131419088,-93.947301914462,1.74480139478656));
#13755=CARTESIAN_POINT('Ctrl Pts',(-207.768707464389,-97.3536847345279,
1.90370971359086));
#13756=CARTESIAN_POINT('Ctrl Pts',(-204.520963212211,-98.6022345372543,
2.06261803239517));
#13757=CARTESIAN_POINT('Ctrl Pts',(-202.235891711733,-96.9311358694141,
2.19190697880573));
#13758=CARTESIAN_POINT('Ctrl Pts',(-201.929850700601,-95.4535575254436,
2.26822648561486));
#13759=CARTESIAN_POINT('Ctrl Pts',(-201.931144087497,-95.0009810700815,
2.29157655282255));
#13760=CARTESIAN_POINT('Ctrl Pts',(-201.930545885435,-94.9983467356882,
1.20842344717746));
#13761=CARTESIAN_POINT('Ctrl Pts',(-201.928558487872,-94.5925295358999,
1.22937114826312));
#13762=CARTESIAN_POINT('Ctrl Pts',(-202.192304255167,-93.1630157504797,
1.30328828895022));
#13763=CARTESIAN_POINT('Ctrl Pts',(-204.358397024947,-91.4231516694834,
1.43017486923876));
#13764=CARTESIAN_POINT('Ctrl Pts',(-207.659318082557,-92.523390293429,1.58908318804306));
#13765=CARTESIAN_POINT('Ctrl Pts',(-208.522221650421,-95.8941719984357,
1.74799150684737));
#13766=CARTESIAN_POINT('Ctrl Pts',(-206.155984228169,-98.445179562461,1.90689982565168));
#13767=CARTESIAN_POINT('Ctrl Pts',(-202.847048276294,-97.8584507200909,
2.06037713909504));
#13768=CARTESIAN_POINT('Ctrl Pts',(-201.92894523571,-95.9131125787372,2.16088501293697));
#13769=CARTESIAN_POINT('Ctrl Pts',(-201.922621816358,-94.9982129686145,
2.20842344717746));
#13770=CARTESIAN_POINT('Origin',(-205.,-95.,-2.20842344717744));
#13771=CARTESIAN_POINT('',(-201.929615858992,-95.0031001153078,0.208423447177458));
#13772=CARTESIAN_POINT('',(-201.92372071423,-94.9977231567353,0.291576552822548));
#13773=CARTESIAN_POINT('',(-201.9265,-94.9999999999997,-2.20842344717744));
#13774=CARTESIAN_POINT('',(-204.206200717467,-97.9692229537457,0.));
#13775=CARTESIAN_POINT('Ctrl Pts',(-204.206200717467,-97.9692229537457,
-1.94289029309402E-15));
#13776=CARTESIAN_POINT('Ctrl Pts',(-203.217993421758,-97.7050332130129,
0.0529694396014337));
#13777=CARTESIAN_POINT('Ctrl Pts',(-202.119889495333,-96.6624088612686,
0.12244392199392));
#13778=CARTESIAN_POINT('Ctrl Pts',(-201.927197987239,-95.3223298493217,
0.191918404386407));
#13779=CARTESIAN_POINT('Ctrl Pts',(-201.929615858992,-95.0031001153078,
0.208423447177458));
#13780=CARTESIAN_POINT('',(-205.795569492778,-97.9745894933442,-2.18341408843227E-15));
#13781=CARTESIAN_POINT('Origin',(-205.,-95.,0.));
#13782=CARTESIAN_POINT('Ctrl Pts',(-205.795570948431,-97.9745939062759,
-4.32461141550156E-16));
#13783=CARTESIAN_POINT('Ctrl Pts',(-204.831203870468,-98.23107300128,0.0519060689144959));
#13784=CARTESIAN_POINT('Ctrl Pts',(-202.766510494357,-97.7537503538027,
0.149098253188679));
#13785=CARTESIAN_POINT('Ctrl Pts',(-201.931000984951,-95.8699154848355,
0.246290437462861));
#13786=CARTESIAN_POINT('Ctrl Pts',(-201.92372071423,-94.9977231567353,0.291576552822548));
#13787=CARTESIAN_POINT('Origin',(-205.,65.,9.));
#13788=CARTESIAN_POINT('',(-202.486496179335,65.0006394388502,16.6125833024919));
#13789=CARTESIAN_POINT('',(-202.48457052599,64.9962980322032,16.8874166975081));
#13790=CARTESIAN_POINT('',(-202.4825,65.,9.));
#13791=CARTESIAN_POINT('',(-203.086534003335,66.6359872033749,17.));
#13792=CARTESIAN_POINT('Ctrl Pts',(-202.48457052599,64.9962980322032,16.8874166975081));
#13793=CARTESIAN_POINT('Ctrl Pts',(-202.489762931999,65.5889737230783,16.9249444650054));
#13794=CARTESIAN_POINT('Ctrl Pts',(-202.700778171916,66.1848035603044,16.9624722325027));
#13795=CARTESIAN_POINT('Ctrl Pts',(-203.086534003335,66.6359872033749,17.));
#13796=CARTESIAN_POINT('',(-202.4825,65.,17.));
#13797=CARTESIAN_POINT('Origin',(-205.,65.,17.));
#13798=CARTESIAN_POINT('',(-202.4825,65.,18.));
#13799=CARTESIAN_POINT('',(-202.4825,65.,9.));
#13800=CARTESIAN_POINT('Origin',(-205.,65.,18.));
#13801=CARTESIAN_POINT('',(-206.917145133663,66.6387833132748,17.));
#13802=CARTESIAN_POINT('Origin',(-205.,65.,17.));
#13803=CARTESIAN_POINT('Ctrl Pts',(-206.917148172614,66.6387856228499,17.));
#13804=CARTESIAN_POINT('Ctrl Pts',(-206.385177397257,67.2593634683583,16.9480939310855));
#13805=CARTESIAN_POINT('Ctrl Pts',(-205.522587697278,67.5988758107765,16.896187862171));
#13806=CARTESIAN_POINT('Ctrl Pts',(-204.71052147175,67.5049508117595,16.8442817932565));
#13807=CARTESIAN_POINT('Ctrl Pts',(-203.881818898331,67.4091016236675,16.791312353655));
#13808=CARTESIAN_POINT('Ctrl Pts',(-203.105731096268,66.8618740047602,16.7383429140536));
#13809=CARTESIAN_POINT('Ctrl Pts',(-202.737501947155,66.1136053435159,16.6853734744522));
#13810=CARTESIAN_POINT('Ctrl Pts',(-202.568829449161,65.7708504460112,16.6611100837988));
#13811=CARTESIAN_POINT('Ctrl Pts',(-202.485734906376,65.3859125981344,16.6368466931454));
#13812=CARTESIAN_POINT('Ctrl Pts',(-202.486496179335,65.0006394388502,16.6125833024919));
#13813=CARTESIAN_POINT('Origin',(-205.,65.,9.));
#13814=CARTESIAN_POINT('',(-202.482814461221,64.9976897634636,15.6125833024919));
#13815=CARTESIAN_POINT('',(-202.478263011551,65.0000328308196,15.8874166975081));
#13816=CARTESIAN_POINT('',(-202.4825,65.,9.));
#13817=CARTESIAN_POINT('Ctrl Pts',(-202.478263011551,65.0000328308196,15.8874166975081));
#13818=CARTESIAN_POINT('Ctrl Pts',(-202.478152266341,65.8352649464484,15.9404611607301));
#13819=CARTESIAN_POINT('Ctrl Pts',(-202.934430616534,66.6703612939895,15.9935056239522));
#13820=CARTESIAN_POINT('Ctrl Pts',(-203.637206972926,67.1217640108908,16.0465500871742));
#13821=CARTESIAN_POINT('Ctrl Pts',(-204.33898935514,67.5725282847932,16.0995195267756));
#13822=CARTESIAN_POINT('Ctrl Pts',(-205.286572131988,67.6406835188332,16.1524889663771));
#13823=CARTESIAN_POINT('Ctrl Pts',(-206.045557105916,67.2948210424227,16.2054584059785));
#13824=CARTESIAN_POINT('Ctrl Pts',(-206.804542079844,66.9489585660121,16.2584278455799));
#13825=CARTESIAN_POINT('Ctrl Pts',(-207.374929250853,66.1890783791509,16.3113972851814));
#13826=CARTESIAN_POINT('Ctrl Pts',(-207.495321313456,65.3638484600988,16.3643667247828));
#13827=CARTESIAN_POINT('Ctrl Pts',(-207.61571337606,64.5386185410466,16.4173361643842));
#13828=CARTESIAN_POINT('Ctrl Pts',(-207.286110330258,63.6480388898036,16.4703056039857));
#13829=CARTESIAN_POINT('Ctrl Pts',(-206.657467900973,63.0996378515271,16.5232750435871));
#13830=CARTESIAN_POINT('Ctrl Pts',(-206.028825471689,62.5512368132507,16.5762444831886));
#13831=CARTESIAN_POINT('Ctrl Pts',(-205.101143658922,62.3450143879409,16.62921392279));
#13832=CARTESIAN_POINT('Ctrl Pts',(-204.29994880059,62.5769614457771,16.6821833623914));
#13833=CARTESIAN_POINT('Ctrl Pts',(-203.498753942257,62.8089085036132,16.7351528019929));
#13834=CARTESIAN_POINT('Ctrl Pts',(-202.824046038359,63.4790250445952,16.7881222415943));
#13835=CARTESIAN_POINT('Ctrl Pts',(-202.584870045267,64.2765863098395,16.8410916811957));
#13836=CARTESIAN_POINT('Ctrl Pts',(-202.515145364615,64.5090916871573,16.8565333532998));
#13837=CARTESIAN_POINT('Ctrl Pts',(-202.482433989863,64.7524278450617,16.871975025404));
#13838=CARTESIAN_POINT('Ctrl Pts',(-202.48457052599,64.9962980322032,16.8874166975081));
#13839=CARTESIAN_POINT('Ctrl Pts',(-202.486496179335,65.0006394388502,16.6125833024919));
#13840=CARTESIAN_POINT('Ctrl Pts',(-202.48739684236,64.5448222644593,16.5838772535439));
#13841=CARTESIAN_POINT('Ctrl Pts',(-202.60567289555,64.0885357450751,16.5551712045959));
#13842=CARTESIAN_POINT('Ctrl Pts',(-202.838472440105,63.7010804418779,16.5264651556478));
#13843=CARTESIAN_POINT('Ctrl Pts',(-203.268042578331,62.9861339050655,16.4734957160464));
#13844=CARTESIAN_POINT('Ctrl Pts',(-204.087553350947,62.5055505350222,16.420526276445));
#13845=CARTESIAN_POINT('Ctrl Pts',(-204.92122518277,62.4795075785488,16.3675568368436));
#13846=CARTESIAN_POINT('Ctrl Pts',(-205.754897014594,62.4534646220754,16.3145873972421));
#13847=CARTESIAN_POINT('Ctrl Pts',(-206.602729905625,62.8819620791719,16.2616179576407));
#13848=CARTESIAN_POINT('Ctrl Pts',(-207.07614049038,63.5686371465989,16.2086485180392));
#13849=CARTESIAN_POINT('Ctrl Pts',(-207.549551075135,64.255312214026,16.1556790784378));
#13850=CARTESIAN_POINT('Ctrl Pts',(-207.648539353615,65.2001648917836,16.1027096388364));
#13851=CARTESIAN_POINT('Ctrl Pts',(-207.32770123824,65.9700518006814,16.0497401992349));
#13852=CARTESIAN_POINT('Ctrl Pts',(-207.006863122865,66.7399387095791,15.9967707596335));
#13853=CARTESIAN_POINT('Ctrl Pts',(-206.266198613636,67.334859849617,15.9438013200321));
#13854=CARTESIAN_POINT('Ctrl Pts',(-205.445237984819,67.4821203893694,15.8908318804306));
#13855=CARTESIAN_POINT('Ctrl Pts',(-204.624277356003,67.6293809291217,15.8378624408292));
#13856=CARTESIAN_POINT('Ctrl Pts',(-203.7230206076,67.3289808685885,15.7848930012278));
#13857=CARTESIAN_POINT('Ctrl Pts',(-203.15459209185,66.7186152645058,15.7319235616263));
#13858=CARTESIAN_POINT('Ctrl Pts',(-202.727701876918,66.2602302667535,15.6921434752482));
#13859=CARTESIAN_POINT('Ctrl Pts',(-202.488527469465,65.6270240651797,15.6523633888701));
#13860=CARTESIAN_POINT('Ctrl Pts',(-202.482814461221,64.9976897634636,15.6125833024919));
#13861=CARTESIAN_POINT('Origin',(-205.,65.,9.));
#13862=CARTESIAN_POINT('',(-202.478480714095,65.0006753766358,14.6125833024919));
#13863=CARTESIAN_POINT('',(-202.48391344512,65.0021895194833,14.8874166975081));
#13864=CARTESIAN_POINT('',(-202.4825,65.,9.));
#13865=CARTESIAN_POINT('Ctrl Pts',(-202.48391344512,65.0021895194833,14.8874166975081));
#13866=CARTESIAN_POINT('Ctrl Pts',(-202.481864131876,65.2491292700526,14.9030084168534));
#13867=CARTESIAN_POINT('Ctrl Pts',(-202.515267256566,65.4955265999556,14.9186001361987));
#13868=CARTESIAN_POINT('Ctrl Pts',(-202.58638727583,65.7305084281609,14.9341918555441));
#13869=CARTESIAN_POINT('Ctrl Pts',(-202.828001909944,66.5288075432794,14.9871612951455));
#13870=CARTESIAN_POINT('Ctrl Pts',(-203.504926567004,67.1953544989996,15.0401307347469));
#13871=CARTESIAN_POINT('Ctrl Pts',(-204.306862968527,67.4246089596421,15.0931001743484));
#13872=CARTESIAN_POINT('Ctrl Pts',(-205.10879937005,67.6538634202845,15.1460696139498));
#13873=CARTESIAN_POINT('Ctrl Pts',(-206.035747516037,67.4458253858491,15.1990390535512));
#13874=CARTESIAN_POINT('Ctrl Pts',(-206.662799141937,66.8958561385943,15.2520084931527));
#13875=CARTESIAN_POINT('Ctrl Pts',(-207.289850767837,66.3458868913395,15.3049779327541));
#13876=CARTESIAN_POINT('Ctrl Pts',(-207.617005873651,65.4539864312653,15.3579473723555));
#13877=CARTESIAN_POINT('Ctrl Pts',(-207.494299240605,64.6290014535642,15.410916811957));
#13878=CARTESIAN_POINT('Ctrl Pts',(-207.37159260756,63.8040164758631,15.4638862515584));
#13879=CARTESIAN_POINT('Ctrl Pts',(-206.799024235656,63.0459469805351,15.5168556911598));
#13880=CARTESIAN_POINT('Ctrl Pts',(-206.039054509905,62.7022785064846,15.5698251307613));
#13881=CARTESIAN_POINT('Ctrl Pts',(-205.279084784155,62.358610032434,15.6227945703627));
#13882=CARTESIAN_POINT('Ctrl Pts',(-204.331713704558,62.4293425796608,15.6757640099641));
#13883=CARTESIAN_POINT('Ctrl Pts',(-203.631214496525,62.8820718503695,15.7287334495656));
#13884=CARTESIAN_POINT('Ctrl Pts',(-202.931707445237,63.3341598949429,15.7816278655464));
#13885=CARTESIAN_POINT('Ctrl Pts',(-202.478373443496,64.1671633420724,15.8345222815272));
#13886=CARTESIAN_POINT('Ctrl Pts',(-202.478263011551,65.0000328308196,15.8874166975081));
#13887=CARTESIAN_POINT('Ctrl Pts',(-202.482814461221,64.9976897634636,15.6125833024919));
#13888=CARTESIAN_POINT('Ctrl Pts',(-202.480920275196,64.7890297740916,15.5993939492686));
#13889=CARTESIAN_POINT('Ctrl Pts',(-202.504690461007,64.5807954220112,15.5862045960453));
#13890=CARTESIAN_POINT('Ctrl Pts',(-202.555792352561,64.3794997079143,15.573015242822));
#13891=CARTESIAN_POINT('Ctrl Pts',(-202.761021412117,63.5710809030377,15.5200458032206));
#13892=CARTESIAN_POINT('Ctrl Pts',(-203.407079814325,62.8745744409167,15.4670763636191));
#13893=CARTESIAN_POINT('Ctrl Pts',(-204.197816415991,62.6092534217428,15.4141069240177));
#13894=CARTESIAN_POINT('Ctrl Pts',(-204.988553017657,62.343932402569,15.3611374844163));
#13895=CARTESIAN_POINT('Ctrl Pts',(-205.92396781878,62.5097968263422,15.3081680448148));
#13896=CARTESIAN_POINT('Ctrl Pts',(-206.575272670495,63.0308161306152,15.2551986052134));
#13897=CARTESIAN_POINT('Ctrl Pts',(-207.226577522209,63.5518354348882,15.202229165612));
#13898=CARTESIAN_POINT('Ctrl Pts',(-207.593772424515,64.4280096196609,15.1492597260105));
#13899=CARTESIAN_POINT('Ctrl Pts',(-207.508536912918,65.2577049646526,15.0962902864091));
#13900=CARTESIAN_POINT('Ctrl Pts',(-207.423301401321,66.0874003096444,15.0433208468077));
#13901=CARTESIAN_POINT('Ctrl Pts',(-206.885635475823,66.8706168148552,14.9903514072062));
#13902=CARTESIAN_POINT('Ctrl Pts',(-206.142002373318,67.2483325911416,14.9373819676048));
#13903=CARTESIAN_POINT('Ctrl Pts',(-205.398369270814,67.6260483674281,14.8844125280034));
#13904=CARTESIAN_POINT('Ctrl Pts',(-204.448768991303,67.5982634147903,14.8314430884019));
#13905=CARTESIAN_POINT('Ctrl Pts',(-203.728492908084,67.1777141128455,14.7784736488005));
#13906=CARTESIAN_POINT('Ctrl Pts',(-203.008216824865,66.7571648109008,14.725504209199));
#13907=CARTESIAN_POINT('Ctrl Pts',(-202.517264937938,65.9438511596491,14.6725347695976));
#13908=CARTESIAN_POINT('Ctrl Pts',(-202.480686891426,65.1105916341598,14.6195653299962));
#13909=CARTESIAN_POINT('Ctrl Pts',(-202.479079745062,65.0739803291702,14.6172379874948));
#13910=CARTESIAN_POINT('Ctrl Pts',(-202.478349767474,65.0373305186669,14.6149106449934));
#13911=CARTESIAN_POINT('Ctrl Pts',(-202.478480714095,65.0006753766358,14.6125833024919));
#13912=CARTESIAN_POINT('Origin',(-205.,65.,9.));
#13913=CARTESIAN_POINT('',(-202.484829356871,65.0019240714538,13.6125833024919));
#13914=CARTESIAN_POINT('',(-202.48603693456,64.9988431445427,13.8874166975081));
#13915=CARTESIAN_POINT('',(-202.4825,65.,9.));
#13916=CARTESIAN_POINT('Ctrl Pts',(-202.48603693456,64.9988431445427,13.8874166975081));
#13917=CARTESIAN_POINT('Ctrl Pts',(-202.488081702897,65.4925818678139,13.9185251125781));
#13918=CARTESIAN_POINT('Ctrl Pts',(-202.628468449655,65.9873937525298,13.9496335276482));
#13919=CARTESIAN_POINT('Ctrl Pts',(-202.899518895525,66.3954024519509,13.9807419427182));
#13920=CARTESIAN_POINT('Ctrl Pts',(-203.361046433623,67.0901338329029,14.0337113823196));
#13921=CARTESIAN_POINT('Ctrl Pts',(-204.201408831768,67.5331956776596,14.0866808219211));
#13922=CARTESIAN_POINT('Ctrl Pts',(-205.035388665575,67.5214909265688,14.1396502615225));
#13923=CARTESIAN_POINT('Ctrl Pts',(-205.869368499381,67.509786175478,14.192619701124));
#13924=CARTESIAN_POINT('Ctrl Pts',(-206.69696576885,67.0433148285397,14.2455891407254));
#13925=CARTESIAN_POINT('Ctrl Pts',(-207.13881450515,66.3359047155866,14.2985585803268));
#13926=CARTESIAN_POINT('Ctrl Pts',(-207.580663241451,65.6284946026335,14.3515280199283));
#13927=CARTESIAN_POINT('Ctrl Pts',(-207.636763444583,64.6801457236657,14.4044974595297));
#13928=CARTESIAN_POINT('Ctrl Pts',(-207.281399106155,63.9255759642922,14.4574668991311));
#13929=CARTESIAN_POINT('Ctrl Pts',(-206.926034767727,63.1710062049186,14.5104363387326));
#13930=CARTESIAN_POINT('Ctrl Pts',(-206.159205887739,62.6102155651394,14.563405778334));
#13931=CARTESIAN_POINT('Ctrl Pts',(-205.332422516349,62.5002672183578,14.6163752179354));
#13932=CARTESIAN_POINT('Ctrl Pts',(-204.505639144959,62.3903188715762,14.6693446575369));
#13933=CARTESIAN_POINT('Ctrl Pts',(-203.618901282167,62.7312128177923,14.7223140971383));
#13934=CARTESIAN_POINT('Ctrl Pts',(-203.078684656356,63.3666854281588,14.7752835367397));
#13935=CARTESIAN_POINT('Ctrl Pts',(-202.697482475075,63.8151046985801,14.8126612569959));
#13936=CARTESIAN_POINT('Ctrl Pts',(-202.488826223208,64.4102057419109,14.850038977252));
#13937=CARTESIAN_POINT('Ctrl Pts',(-202.48391344512,65.0021895194833,14.8874166975081));
#13938=CARTESIAN_POINT('Ctrl Pts',(-202.478480714095,65.0006753766358,14.6125833024919));
#13939=CARTESIAN_POINT('Ctrl Pts',(-202.481330063292,64.2030732786072,14.5619412053919));
#13940=CARTESIAN_POINT('Ctrl Pts',(-202.891810860674,63.4029468022227,14.5112991082919));
#13941=CARTESIAN_POINT('Ctrl Pts',(-203.54255899523,62.9420800015405,14.4606570111919));
#13942=CARTESIAN_POINT('Ctrl Pts',(-204.223213351645,62.4600332941377,14.4076875715904));
#13943=CARTESIAN_POINT('Ctrl Pts',(-205.166726270573,62.349145279059,14.354718131989));
#13944=CARTESIAN_POINT('Ctrl Pts',(-205.940596712799,62.6602464127481,14.3017486923876));
#13945=CARTESIAN_POINT('Ctrl Pts',(-206.714467155025,62.9713475464372,14.2487792527861));
#13946=CARTESIAN_POINT('Ctrl Pts',(-207.318695120548,63.7044378288941,14.1958098131847));
#13947=CARTESIAN_POINT('Ctrl Pts',(-207.476305881734,64.5234727665736,14.1428403735833));
#13948=CARTESIAN_POINT('Ctrl Pts',(-207.63391664292,65.3425077042531,14.0898709339818));
#13949=CARTESIAN_POINT('Ctrl Pts',(-207.344910199768,66.2474872971551,14.0369014943804));
#13950=CARTESIAN_POINT('Ctrl Pts',(-206.74176549312,66.8235739596422,13.9839320547789));
#13951=CARTESIAN_POINT('Ctrl Pts',(-206.138620786471,67.3996606221293,13.9309626151775));
#13952=CARTESIAN_POINT('Ctrl Pts',(-205.221337816326,67.6468543542013,13.8779931755761));
#13953=CARTESIAN_POINT('Ctrl Pts',(-204.4103939689,67.4518429293449,13.8250237359746));
#13954=CARTESIAN_POINT('Ctrl Pts',(-203.599450121474,67.2568315044885,13.7720542963732));
#13955=CARTESIAN_POINT('Ctrl Pts',(-202.894845396768,66.6196149227036,13.7190848567718));
#13956=CARTESIAN_POINT('Ctrl Pts',(-202.619566663537,65.8322897046192,13.6661154171703));
#13957=CARTESIAN_POINT('Ctrl Pts',(-202.526832357198,65.5670601421846,13.6482713789442));
#13958=CARTESIAN_POINT('Ctrl Pts',(-202.482819782445,65.2847956160355,13.6304273407181));
#13959=CARTESIAN_POINT('Ctrl Pts',(-202.484829356871,65.0019240714538,13.6125833024919));
#13960=CARTESIAN_POINT('Origin',(-205.,65.,9.));
#13961=CARTESIAN_POINT('',(-202.485436378814,64.9983728001324,12.6125833024919));
#13962=CARTESIAN_POINT('',(-202.479673360095,64.9983441228843,12.8874166975081));
#13963=CARTESIAN_POINT('',(-202.4825,65.,9.));
#13964=CARTESIAN_POINT('Ctrl Pts',(-202.479673360095,64.9983441228843,12.8874166975081));
#13965=CARTESIAN_POINT('Ctrl Pts',(-202.48526219209,65.7335978500889,12.9340418083028));
#13966=CARTESIAN_POINT('Ctrl Pts',(-202.82574540688,66.473357371898,12.9806669190976));
#13967=CARTESIAN_POINT('Ctrl Pts',(-203.391061399314,66.9417737892996,13.0272920298924));
#13968=CARTESIAN_POINT('Ctrl Pts',(-204.033300544841,67.4739281307464,13.0802614694938));
#13969=CARTESIAN_POINT('Ctrl Pts',(-204.965721796711,67.655871464688,13.1332309090952));
#13970=CARTESIAN_POINT('Ctrl Pts',(-205.760908463841,67.4042019838009,13.1862003486967));
#13971=CARTESIAN_POINT('Ctrl Pts',(-206.556095130971,67.1525325029139,13.2391697882981));
#13972=CARTESIAN_POINT('Ctrl Pts',(-207.214047213361,66.467250207198,13.2921392278995));
#13973=CARTESIAN_POINT('Ctrl Pts',(-207.433163153269,65.6624846710021,13.345108667501));
#13974=CARTESIAN_POINT('Ctrl Pts',(-207.652279093177,64.8577191348062,13.3980781071024));
#13975=CARTESIAN_POINT('Ctrl Pts',(-207.432558890604,63.9334703581302,13.4510475467039));
#13976=CARTESIAN_POINT('Ctrl Pts',(-206.874721058672,63.3134088159122,13.5040169863053));
#13977=CARTESIAN_POINT('Ctrl Pts',(-206.31688322674,62.6933472736942,13.5569864259067));
#13978=CARTESIAN_POINT('Ctrl Pts',(-205.420927765449,62.377472965934,13.6099558655082));
#13979=CARTESIAN_POINT('Ctrl Pts',(-204.597555650998,62.5105809084757,13.6629253051096));
#13980=CARTESIAN_POINT('Ctrl Pts',(-203.774183536547,62.6436888510174,13.715894744711));
#13981=CARTESIAN_POINT('Ctrl Pts',(-203.023394768935,63.2257790438609,13.7688641843125));
#13982=CARTESIAN_POINT('Ctrl Pts',(-202.689346724155,63.9900245988563,13.8218336239139));
#13983=CARTESIAN_POINT('Ctrl Pts',(-202.551481710733,64.305436484492,13.8436946484453));
#13984=CARTESIAN_POINT('Ctrl Pts',(-202.484600000834,64.6518748301101,13.8655556729767));
#13985=CARTESIAN_POINT('Ctrl Pts',(-202.48603693456,64.9988431445427,13.8874166975081));
#13986=CARTESIAN_POINT('Ctrl Pts',(-202.484829356871,65.0019240714538,13.6125833024919));
#13987=CARTESIAN_POINT('Ctrl Pts',(-202.488785137923,64.4451007551634,13.5774579011166));
#13988=CARTESIAN_POINT('Ctrl Pts',(-202.671070421135,63.8859253258832,13.5423324997413));
#13989=CARTESIAN_POINT('Ctrl Pts',(-203.0110940357,63.4497025812941,13.507207098366));
#13990=CARTESIAN_POINT('Ctrl Pts',(-203.523852882846,62.7918745304371,13.4542376587646));
#13991=CARTESIAN_POINT('Ctrl Pts',(-204.395323318893,62.4136522831071,13.4012682191632));
#13992=CARTESIAN_POINT('Ctrl Pts',(-205.226028166212,62.4884108039558,13.3482987795617));
#13993=CARTESIAN_POINT('Ctrl Pts',(-206.05673301353,62.5631693248045,13.2953293399603));
#13994=CARTESIAN_POINT('Ctrl Pts',(-206.84667227212,63.0909086138319,13.2423599003589));
#13995=CARTESIAN_POINT('Ctrl Pts',(-207.233742200274,63.8297159301003,13.1893904607574));
#13996=CARTESIAN_POINT('Ctrl Pts',(-207.620812128428,64.5685232463688,13.136421021156));
#13997=CARTESIAN_POINT('Ctrl Pts',(-207.605012726144,65.5183985898783,13.0834515815545));
#13998=CARTESIAN_POINT('Ctrl Pts',(-207.193586351169,66.2439244114753,13.0304821419531));
#13999=CARTESIAN_POINT('Ctrl Pts',(-206.782159976194,66.9694502330724,12.9775127023517));
#14000=CARTESIAN_POINT('Ctrl Pts',(-205.975106628526,67.4706265327569,12.9245432627502));
#14001=CARTESIAN_POINT('Ctrl Pts',(-205.142375052588,67.5177168955105,12.8715738231488));
#14002=CARTESIAN_POINT('Ctrl Pts',(-204.30964347665,67.5648072582641,12.8186043835474));
#14003=CARTESIAN_POINT('Ctrl Pts',(-203.451233672441,67.1578116840866,12.7656349439459));
#14004=CARTESIAN_POINT('Ctrl Pts',(-202.960635897084,66.4832946697357,12.7126655043445));
#14005=CARTESIAN_POINT('Ctrl Pts',(-202.651652038019,66.0584764570002,12.6793047703936));
#14006=CARTESIAN_POINT('Ctrl Pts',(-202.48856518007,65.5275426939449,12.6459440364428));
#14007=CARTESIAN_POINT('Ctrl Pts',(-202.485436378814,64.9983728001324,12.6125833024919));
#14008=CARTESIAN_POINT('Origin',(-205.,65.,9.));
#14009=CARTESIAN_POINT('',(-202.478899910386,64.9988537237822,11.6125833024919));
#14010=CARTESIAN_POINT('',(-202.480895712983,65.0021035865431,11.8874166975081));
#14011=CARTESIAN_POINT('',(-202.4825,65.,9.));
#14012=CARTESIAN_POINT('Ctrl Pts',(-202.480895712983,65.0021035865431,11.8874166975081));
#14013=CARTESIAN_POINT('Ctrl Pts',(-202.479598519915,65.1469297626336,11.8965890644261));
#14014=CARTESIAN_POINT('Ctrl Pts',(-202.491010908424,65.2915516069264,11.9057614313442));
#14015=CARTESIAN_POINT('Ctrl Pts',(-202.515857741095,65.4338272778794,11.9149337982622));
#14016=CARTESIAN_POINT('Ctrl Pts',(-202.659345546828,66.2554540865998,11.9679032378637));
#14017=CARTESIAN_POINT('Ctrl Pts',(-203.250863894479,66.998837441384,12.0208726774651));
#14018=CARTESIAN_POINT('Ctrl Pts',(-204.019264079124,67.3232145667187,12.0738421170665));
#14019=CARTESIAN_POINT('Ctrl Pts',(-204.787664263768,67.6475916920535,12.126811556668));
#14020=CARTESIAN_POINT('Ctrl Pts',(-205.732946285406,67.5529625879387,12.1797809962694));
#14021=CARTESIAN_POINT('Ctrl Pts',(-206.421798147929,67.0827047068781,12.2327504358708));
#14022=CARTESIAN_POINT('Ctrl Pts',(-207.110650010453,66.6124468258175,12.2857198754723));
#14023=CARTESIAN_POINT('Ctrl Pts',(-207.543071713862,65.7665601678111,12.3386893150737));
#14024=CARTESIAN_POINT('Ctrl Pts',(-207.520843565857,64.9327944497339,12.3916587546751));
#14025=CARTESIAN_POINT('Ctrl Pts',(-207.498615417853,64.0990287316567,12.4446281942766));
#14026=CARTESIAN_POINT('Ctrl Pts',(-207.021737418434,63.2773839535086,12.497597633878));
#14027=CARTESIAN_POINT('Ctrl Pts',(-206.308807777554,62.8444974899262,12.5505670734795));
#14028=CARTESIAN_POINT('Ctrl Pts',(-205.595878136674,62.4116110263438,12.6035365130809));
#14029=CARTESIAN_POINT('Ctrl Pts',(-204.646896854331,62.367482877327,12.6565059526823));
#14030=CARTESIAN_POINT('Ctrl Pts',(-203.896871647065,62.7323411397584,12.7094753922838));
#14031=CARTESIAN_POINT('Ctrl Pts',(-203.146846439799,63.0971994021897,12.7624448318852));
#14032=CARTESIAN_POINT('Ctrl Pts',(-202.595777307608,63.8710440760693,12.8154142714866));
#14033=CARTESIAN_POINT('Ctrl Pts',(-202.496271261105,64.6991490874851,12.8683837110881));
#14034=CARTESIAN_POINT('Ctrl Pts',(-202.484353085606,64.7983340235237,12.8747280398947));
#14035=CARTESIAN_POINT('Ctrl Pts',(-202.478912881734,64.8982973600521,12.8810723687014));
#14036=CARTESIAN_POINT('Ctrl Pts',(-202.479673360095,64.9983441228843,12.8874166975081));
#14037=CARTESIAN_POINT('Ctrl Pts',(-202.485436378814,64.9983728001324,12.6125833024919));
#14038=CARTESIAN_POINT('Ctrl Pts',(-202.483597338253,64.6873383755837,12.5929745968414));
#14039=CARTESIAN_POINT('Ctrl Pts',(-202.537021084319,64.3769133378432,12.5733658911908));
#14040=CARTESIAN_POINT('Ctrl Pts',(-202.648562957585,64.0890044692285,12.5537571855402));
#14041=CARTESIAN_POINT('Ctrl Pts',(-202.94987353995,63.3112697375966,12.5007877459388));
#14042=CARTESIAN_POINT('Ctrl Pts',(-203.675280451186,62.6978387288571,12.4478183063373));
#14043=CARTESIAN_POINT('Ctrl Pts',(-204.492261217045,62.5299047893222,12.3948488667359));
#14044=CARTESIAN_POINT('Ctrl Pts',(-205.309241982905,62.3619708497873,12.3418794271344));
#14045=CARTESIAN_POINT('Ctrl Pts',(-206.217796603388,62.639533979457,12.288909987533));
#14046=CARTESIAN_POINT('Ctrl Pts',(-206.801448717827,63.2353607908227,12.2359405479316));
#14047=CARTESIAN_POINT('Ctrl Pts',(-207.385100832267,63.8311876021884,12.1829711083301));
#14048=CARTESIAN_POINT('Ctrl Pts',(-207.643850440664,64.7452780952501,12.1300016687287));
#14049=CARTESIAN_POINT('Ctrl Pts',(-207.459088168525,65.5586182962889,12.0770322291273));
#14050=CARTESIAN_POINT('Ctrl Pts',(-207.274325896385,66.3719584973278,12.0240627895258));
#14051=CARTESIAN_POINT('Ctrl Pts',(-206.64605174371,67.0845484063438,11.9710933499244));
#14052=CARTESIAN_POINT('Ctrl Pts',(-205.862263071039,67.3697407912789,11.918123910323));
#14053=CARTESIAN_POINT('Ctrl Pts',(-205.078474398368,67.6549331762139,11.8651544707215));
#14054=CARTESIAN_POINT('Ctrl Pts',(-204.139171205702,67.512728037068,11.8121850311201));
#14055=CARTESIAN_POINT('Ctrl Pts',(-203.47492482736,67.0083114149271,11.7592155915187));
#14056=CARTESIAN_POINT('Ctrl Pts',(-202.861992995554,66.5428621264053,11.7103381618431));
#14057=CARTESIAN_POINT('Ctrl Pts',(-202.483261962138,65.7690030327609,11.6614607321675));
#14058=CARTESIAN_POINT('Ctrl Pts',(-202.478899910386,64.9988537237822,11.6125833024919));
#14059=CARTESIAN_POINT('Origin',(-205.,65.,9.));
#14060=CARTESIAN_POINT('',(-202.481967556149,65.0022835844395,10.6125833024919));
#14061=CARTESIAN_POINT('',(-202.486473208904,65.0004666846809,10.8874166975081));
#14062=CARTESIAN_POINT('',(-202.4825,65.,9.));
#14063=CARTESIAN_POINT('Ctrl Pts',(-202.486473208904,65.0004666846809,10.8874166975081));
#14064=CARTESIAN_POINT('Ctrl Pts',(-202.485824990019,65.3924902192974,10.9121057601508));
#14065=CARTESIAN_POINT('Ctrl Pts',(-202.571984008169,65.784244058827,10.9367948227936));
#14066=CARTESIAN_POINT('Ctrl Pts',(-202.746442526037,66.1316570068074,10.9614838854364));
#14067=CARTESIAN_POINT('Ctrl Pts',(-203.120736603494,66.8770181989703,11.0144533250378));
#14068=CARTESIAN_POINT('Ctrl Pts',(-203.901473819497,67.4182779954878,11.0674227646393));
#14069=CARTESIAN_POINT('Ctrl Pts',(-204.730768597298,67.5073259304104,11.1203922042407));
#14070=CARTESIAN_POINT('Ctrl Pts',(-205.560063375099,67.5963738653331,11.1733616438421));
#14071=CARTESIAN_POINT('Ctrl Pts',(-206.437915714699,67.2332099386611,11.2263310834436));
#14072=CARTESIAN_POINT('Ctrl Pts',(-206.961923009412,66.5843064648767,11.279300523045));
#14073=CARTESIAN_POINT('Ctrl Pts',(-207.485930304125,65.9354029910924,11.3322699626464));
#14074=CARTESIAN_POINT('Ctrl Pts',(-207.656092553952,65.0007599701958,11.3852394022479));
#14075=CARTESIAN_POINT('Ctrl Pts',(-207.394408334505,64.2088125398099,11.4382088418493));
#14076=CARTESIAN_POINT('Ctrl Pts',(-207.132724115059,63.416865109424,11.4911782814507));
#14077=CARTESIAN_POINT('Ctrl Pts',(-206.439193426339,62.7676132695489,11.5441477210522));
#14078=CARTESIAN_POINT('Ctrl Pts',(-205.631726860331,62.5586704353066,11.5971171606536));
#14079=CARTESIAN_POINT('Ctrl Pts',(-204.824260294323,62.3497276010643,11.650086600255));
#14080=CARTESIAN_POINT('Ctrl Pts',(-203.902857851026,62.5810937724549,11.7030560398565));
#14081=CARTESIAN_POINT('Ctrl Pts',(-203.289885261286,63.1467119894785,11.7560254794579));
#14082=CARTESIAN_POINT('Ctrl Pts',(-202.783057073792,63.614385847243,11.7998225521413));
#14083=CARTESIAN_POINT('Ctrl Pts',(-202.48708967138,64.3105740590657,11.8436196248247));
#14084=CARTESIAN_POINT('Ctrl Pts',(-202.480895712983,65.0021035865431,11.8874166975081));
#14085=CARTESIAN_POINT('Ctrl Pts',(-202.478899910386,64.9988537237822,11.6125833024919));
#14086=CARTESIAN_POINT('Ctrl Pts',(-202.478534720171,64.9343769573553,11.6084912925661));
#14087=CARTESIAN_POINT('Ctrl Pts',(-202.48079348564,64.8699261928438,11.6043992826402));
#14088=CARTESIAN_POINT('Ctrl Pts',(-202.485758456508,64.8056845798517,11.6003072727143));
#14089=CARTESIAN_POINT('Ctrl Pts',(-202.550028028015,63.9741024720533,11.5473378331129));
#14090=CARTESIAN_POINT('Ctrl Pts',(-203.067756735046,63.1775663615925,11.4943683935115));
#14091=CARTESIAN_POINT('Ctrl Pts',(-203.801620631571,62.781203950145,11.44139895391));
#14092=CARTESIAN_POINT('Ctrl Pts',(-204.535484528097,62.3848415386974,11.3884295143086));
#14093=CARTESIAN_POINT('Ctrl Pts',(-205.485483614117,62.388652826263,11.3354600747072));
#14094=CARTESIAN_POINT('Ctrl Pts',(-206.216143617571,62.7908907399206,11.2824906351057));
#14095=CARTESIAN_POINT('Ctrl Pts',(-206.946803621026,63.1931286535783,11.2295211955043));
#14096=CARTESIAN_POINT('Ctrl Pts',(-207.458124541916,63.9937931933281,11.1765517559029));
#14097=CARTESIAN_POINT('Ctrl Pts',(-207.515719727568,64.8258642085796,11.1235823163014));
#14098=CARTESIAN_POINT('Ctrl Pts',(-207.57331491322,65.6579352238312,11.0706128767));
#14099=CARTESIAN_POINT('Ctrl Pts',(-207.177184363636,66.5214127145845,11.0176434370986));
#14100=CARTESIAN_POINT('Ctrl Pts',(-206.508912109009,67.0204834245331,10.9646739974971));
#14101=CARTESIAN_POINT('Ctrl Pts',(-205.840639854383,67.5195541344816,10.9117045578957));
#14102=CARTESIAN_POINT('Ctrl Pts',(-204.900225894714,67.6542180636253,10.8587351182942));
#14103=CARTESIAN_POINT('Ctrl Pts',(-204.11875073371,67.3627460194001,10.8057656786928));
#14104=CARTESIAN_POINT('Ctrl Pts',(-203.337275572705,67.0712739751749,10.7527962390914));
#14105=CARTESIAN_POINT('Ctrl Pts',(-202.714739210364,66.3536659575809,10.6998267994899));
#14106=CARTESIAN_POINT('Ctrl Pts',(-202.536508836204,65.5388694716049,10.6468573598885));
#14107=CARTESIAN_POINT('Ctrl Pts',(-202.498067311432,65.3631305188742,10.6354326740897));
#14108=CARTESIAN_POINT('Ctrl Pts',(-202.48029480925,65.1828703787145,10.6240079882908));
#14109=CARTESIAN_POINT('Ctrl Pts',(-202.481967556149,65.0022835844395,10.6125833024919));
#14110=CARTESIAN_POINT('Origin',(-205.,65.,9.));
#14111=CARTESIAN_POINT('',(-202.486546886373,64.9998805727156,9.61258330249194));
#14112=CARTESIAN_POINT('',(-202.482611670102,64.997686958861,9.88741669750806));
#14113=CARTESIAN_POINT('',(-202.4825,65.,9.));
#14114=CARTESIAN_POINT('Ctrl Pts',(-202.482611670102,64.997686958861,9.88741669750806));
#14115=CARTESIAN_POINT('Ctrl Pts',(-202.488432746159,65.6336242075107,9.92762245587555));
#14116=CARTESIAN_POINT('Ctrl Pts',(-202.733277868516,66.2735520171247,9.96782821424304));
#14117=CARTESIAN_POINT('Ctrl Pts',(-203.168440184143,66.7333659482197,10.0080339726105));
#14118=CARTESIAN_POINT('Ctrl Pts',(-203.741748708353,67.3391519659441,10.061003412212));
#14119=CARTESIAN_POINT('Ctrl Pts',(-204.64539046284,67.6323146295356,10.1139728518134));
#14120=CARTESIAN_POINT('Ctrl Pts',(-205.465141117256,67.4784698123131,10.1669422914149));
#14121=CARTESIAN_POINT('Ctrl Pts',(-206.284891771673,67.3246249950906,10.2199117310163));
#14122=CARTESIAN_POINT('Ctrl Pts',(-207.020751326018,66.7237726970541,10.2728811706177));
#14123=CARTESIAN_POINT('Ctrl Pts',(-207.335405872855,65.9513402538225,10.3258506102192));
#14124=CARTESIAN_POINT('Ctrl Pts',(-207.650060419693,65.178907810591,10.3788200498206));
#14125=CARTESIAN_POINT('Ctrl Pts',(-207.543509959022,64.2348952221644,10.431789489422));
#14126=CARTESIAN_POINT('Ctrl Pts',(-207.064596626569,63.5520325835608,10.4847589290235));
#14127=CARTESIAN_POINT('Ctrl Pts',(-206.585683294116,62.8691699449572,10.5377283686249));
#14128=CARTESIAN_POINT('Ctrl Pts',(-205.73440708988,62.4474572561765,10.5906978082263));
#14129=CARTESIAN_POINT('Ctrl Pts',(-204.900988268614,62.4802052570581,10.6436672478278));
#14130=CARTESIAN_POINT('Ctrl Pts',(-204.067569447348,62.5129532579397,10.6966366874292));
#14131=CARTESIAN_POINT('Ctrl Pts',(-203.252008009052,63.0001619484835,10.7496061270306));
#14132=CARTESIAN_POINT('Ctrl Pts',(-202.82815275936,63.7184975876597,10.8025755666321));
#14133=CARTESIAN_POINT('Ctrl Pts',(-202.601856496319,64.1020168925947,10.8308559435907));
#14134=CARTESIAN_POINT('Ctrl Pts',(-202.487215718844,64.5514187197568,10.8591363205494));
#14135=CARTESIAN_POINT('Ctrl Pts',(-202.486473208904,65.0004666846809,10.8874166975081));
#14136=CARTESIAN_POINT('Ctrl Pts',(-202.481967556149,65.0022835844395,10.6125833024919));
#14137=CARTESIAN_POINT('Ctrl Pts',(-202.488050336832,64.3455973490155,10.5710385486894));
#14138=CARTESIAN_POINT('Ctrl Pts',(-202.751265847009,63.6845916284616,10.5294937948868));
#14139=CARTESIAN_POINT('Ctrl Pts',(-203.212768103735,63.220963415075,10.4879490410842));
#14140=CARTESIAN_POINT('Ctrl Pts',(-203.801182131406,62.6298387988791,10.4349796014828));
#14141=CARTESIAN_POINT('Ctrl Pts',(-204.711934572726,62.3595745208452,10.3820101618813));
#14142=CARTESIAN_POINT('Ctrl Pts',(-205.52754159824,62.5340582156802,10.3290407222799));
#14143=CARTESIAN_POINT('Ctrl Pts',(-206.343148623755,62.7085419105152,10.2760712826785));
#14144=CARTESIAN_POINT('Ctrl Pts',(-207.063610233464,63.327773578219,10.223101843077));
#14145=CARTESIAN_POINT('Ctrl Pts',(-207.358670851702,64.1079008828283,10.1701324034756));
#14146=CARTESIAN_POINT('Ctrl Pts',(-207.65373146994,64.8880281874377,10.1171629638742));
#14147=CARTESIAN_POINT('Ctrl Pts',(-207.523391096707,65.8290511289526,10.0641935242727));
#14148=CARTESIAN_POINT('Ctrl Pts',(-207.0273970307,66.4996100497921,10.0112240846713));
#14149=CARTESIAN_POINT('Ctrl Pts',(-206.531402964692,67.1701689706315,9.95825464506984));
#14150=CARTESIAN_POINT('Ctrl Pts',(-205.66975520591,67.5702638707955,9.90528520546841));
#14151=CARTESIAN_POINT('Ctrl Pts',(-204.837428271749,67.5164934839379,9.85231576586697));
#14152=CARTESIAN_POINT('Ctrl Pts',(-204.005101337589,67.4627230970802,9.79934632626553));
#14153=CARTESIAN_POINT('Ctrl Pts',(-203.20209522805,66.955087423201,9.7463768866641));
#14154=CARTESIAN_POINT('Ctrl Pts',(-202.796503456228,66.2262838183368,9.69340744706266));
#14155=CARTESIAN_POINT('Ctrl Pts',(-202.590210870358,65.8555988323875,9.66646606553909));
#14156=CARTESIAN_POINT('Ctrl Pts',(-202.486727607399,65.4276986856451,9.63952468401551));
#14157=CARTESIAN_POINT('Ctrl Pts',(-202.486546886373,64.9998805727156,9.61258330249194));
#14158=CARTESIAN_POINT('Origin',(-205.,65.,9.));
#14159=CARTESIAN_POINT('',(-202.48152822651,64.9977697676256,8.61258330249193));
#14160=CARTESIAN_POINT('',(-202.478564103745,65.0007934494835,8.88741669750805));
#14161=CARTESIAN_POINT('',(-202.4825,65.,9.));
#14162=CARTESIAN_POINT('Ctrl Pts',(-202.478564103745,65.0007934494835,8.88741669750805));
#14163=CARTESIAN_POINT('Ctrl Pts',(-202.478385247511,65.044156657915,8.89016971199883));
#14164=CARTESIAN_POINT('Ctrl Pts',(-202.479406854651,65.0875112638012,8.89292272648962));
#14165=CARTESIAN_POINT('Ctrl Pts',(-202.48165537137,65.130802144333,8.8956757409804));
#14166=CARTESIAN_POINT('Ctrl Pts',(-202.524918009827,65.9637413421835,8.94864518058183));
#14167=CARTESIAN_POINT('Ctrl Pts',(-203.02237980079,66.7730895579156,9.00161462018326));
#14168=CARTESIAN_POINT('Ctrl Pts',(-203.746007039296,67.1878460923965,9.0545840597847));
#14169=CARTESIAN_POINT('Ctrl Pts',(-204.469634277802,67.6026026268774,9.10755349938614));
#14170=CARTESIAN_POINT('Ctrl Pts',(-205.41942696385,67.6227674801071,9.16052293898758));
#14171=CARTESIAN_POINT('Ctrl Pts',(-206.160005437975,67.2390971960543,9.21349237858901));
#14172=CARTESIAN_POINT('Ctrl Pts',(-206.9005839121,66.8554269120015,9.26646181819045));
#14173=CARTESIAN_POINT('Ctrl Pts',(-207.431948174301,66.0679214906662,9.31943125779188));
#14174=CARTESIAN_POINT('Ctrl Pts',(-207.510523816259,65.2375690162959,9.37240069739331));
#14175=CARTESIAN_POINT('Ctrl Pts',(-207.589099458218,64.4072165419256,9.42537013699475));
#14176=CARTESIAN_POINT('Ctrl Pts',(-207.214886479934,63.5340170145203,9.47833957659619));
#14177=CARTESIAN_POINT('Ctrl Pts',(-206.559422019403,63.0182402176573,9.53130901619763));
#14178=CARTESIAN_POINT('Ctrl Pts',(-205.903957558871,62.5024634207942,9.58427845579906));
#14179=CARTESIAN_POINT('Ctrl Pts',(-204.967241616092,62.3441093544734,9.6372478954005));
#14180=CARTESIAN_POINT('Ctrl Pts',(-204.178659544495,62.615766637751,9.69021733500193));
#14181=CARTESIAN_POINT('Ctrl Pts',(-203.390077472898,62.8874239210286,9.74318677460337));
#14182=CARTESIAN_POINT('Ctrl Pts',(-202.749629272483,63.5890925539047,9.7961562142048));
#14183=CARTESIAN_POINT('Ctrl Pts',(-202.550892819242,64.3991315562713,9.84912565380624));
#14184=CARTESIAN_POINT('Ctrl Pts',(-202.503004664151,64.5943210785895,9.86188933504018));
#14185=CARTESIAN_POINT('Ctrl Pts',(-202.480763716917,64.7958029338822,9.87465301627412));
#14186=CARTESIAN_POINT('Ctrl Pts',(-202.482611670102,64.997686958861,9.88741669750806));
#14187=CARTESIAN_POINT('Ctrl Pts',(-202.486546886373,64.9998805727156,9.61258330249194));
#14188=CARTESIAN_POINT('Ctrl Pts',(-202.486372291861,64.5865656623298,9.58655524441408));
#14189=CARTESIAN_POINT('Ctrl Pts',(-202.582614964632,64.1733273180761,9.56052718633622));
#14190=CARTESIAN_POINT('Ctrl Pts',(-202.775719644012,63.8118308540053,9.53449912825836));
#14191=CARTESIAN_POINT('Ctrl Pts',(-203.16870503772,63.0761530303869,9.48152968865693));
#14192=CARTESIAN_POINT('Ctrl Pts',(-203.962853259241,62.554768918999,9.42856024905549));
#14193=CARTESIAN_POINT('Ctrl Pts',(-204.794131201844,62.4866780828008,9.37559080945405));
#14194=CARTESIAN_POINT('Ctrl Pts',(-205.625409144447,62.4185872466025,9.32262136985262));
#14195=CARTESIAN_POINT('Ctrl Pts',(-206.493816808132,62.8037896855938,9.26965193025118));
#14196=CARTESIAN_POINT('Ctrl Pts',(-207.001280972872,63.4657107544051,9.21668249064975));
#14197=CARTESIAN_POINT('Ctrl Pts',(-207.508745137613,64.1276318232163,9.16371305104831));
#14198=CARTESIAN_POINT('Ctrl Pts',(-207.655265803409,65.0662715218476,9.11074361144688));
#14199=CARTESIAN_POINT('Ctrl Pts',(-207.373678715875,65.8513626579371,9.05777417184544));
#14200=CARTESIAN_POINT('Ctrl Pts',(-207.092091628341,66.6364537940267,9.004804732244));
#14201=CARTESIAN_POINT('Ctrl Pts',(-206.382396787478,67.2679963675745,8.95183529264257));
#14202=CARTESIAN_POINT('Ctrl Pts',(-205.56991434228,67.4564947921768,8.89886585304113));
#14203=CARTESIAN_POINT('Ctrl Pts',(-204.757431897082,67.644993216779,8.8458964134397));
#14204=CARTESIAN_POINT('Ctrl Pts',(-203.84216184755,67.3904474924357,8.79292697383826));
#14205=CARTESIAN_POINT('Ctrl Pts',(-203.243658869497,66.8095399566832,8.73995753423683));
#14206=CARTESIAN_POINT('Ctrl Pts',(-202.763924028678,66.3439088831306,8.69749945698853));
#14207=CARTESIAN_POINT('Ctrl Pts',(-202.48771051161,65.6685919114507,8.65504137974023));
#14208=CARTESIAN_POINT('Ctrl Pts',(-202.48152822651,64.9977697676256,8.61258330249193));
#14209=CARTESIAN_POINT('Origin',(-205.,65.,9.));
#14210=CARTESIAN_POINT('',(-202.479185657883,65.0013671530438,7.61258330249194));
#14211=CARTESIAN_POINT('',(-202.484985693937,65.0018590734507,7.88741669750805));
#14212=CARTESIAN_POINT('',(-202.4825,65.,9.));
#14213=CARTESIAN_POINT('Ctrl Pts',(-202.484985693937,65.0018590734507,7.88741669750805));
#14214=CARTESIAN_POINT('Ctrl Pts',(-202.483005747609,65.2915238451685,7.90568640772355));
#14215=CARTESIAN_POINT('Ctrl Pts',(-202.529199000709,65.5805765589219,7.92395611793905));
#14216=CARTESIAN_POINT('Ctrl Pts',(-202.626321312497,65.851362647761,7.94222582815455));
#14217=CARTESIAN_POINT('Ctrl Pts',(-202.907908396665,66.6364537744666,7.99519526775599));
#14218=CARTESIAN_POINT('Ctrl Pts',(-203.617603229046,67.2679963404659,8.04816470735743));
#14219=CARTESIAN_POINT('Ctrl Pts',(-204.430085664532,67.4564947628151,8.10113414695886));
#14220=CARTESIAN_POINT('Ctrl Pts',(-205.242568100018,67.6449931851643,8.1541035865603));
#14221=CARTESIAN_POINT('Ctrl Pts',(-206.15783813861,67.3904474638634,8.20707302616174));
#14222=CARTESIAN_POINT('Ctrl Pts',(-206.756341109509,66.8095399350544,8.26004246576317));
#14223=CARTESIAN_POINT('Ctrl Pts',(-207.354844080409,66.2286324062453,8.3130119053646));
#14224=CARTESIAN_POINT('Ctrl Pts',(-207.636579983615,65.3213630699281,8.36598134496604));
#14225=CARTESIAN_POINT('Ctrl Pts',(-207.47240265555,64.5036191196896,8.41895078456747));
#14226=CARTESIAN_POINT('Ctrl Pts',(-207.308225327486,63.6858751694511,8.47192022416891));
#14227=CARTESIAN_POINT('Ctrl Pts',(-206.69813476815,62.9576566052913,8.52488966377034));
#14228=CARTESIAN_POINT('Ctrl Pts',(-205.921793080516,62.6527747474469,8.57785910337178));
#14229=CARTESIAN_POINT('Ctrl Pts',(-205.145451392881,62.3478928896025,8.63082854297322));
#14230=CARTESIAN_POINT('Ctrl Pts',(-204.202858576947,62.4663477380736,8.68379798257465));
#14231=CARTESIAN_POINT('Ctrl Pts',(-203.526093911955,62.9538402522936,8.73676742217609));
#14232=CARTESIAN_POINT('Ctrl Pts',(-202.884503168825,63.4159960069425,8.78698384728674));
#14233=CARTESIAN_POINT('Ctrl Pts',(-202.481826535046,64.2098258334208,8.8372002723974));
#14234=CARTESIAN_POINT('Ctrl Pts',(-202.478564103745,65.0007934494835,8.88741669750805));
#14235=CARTESIAN_POINT('Ctrl Pts',(-202.48152822651,64.9977697676256,8.61258330249193));
#14236=CARTESIAN_POINT('Ctrl Pts',(-202.479997675833,64.831694074018,8.60207194013879));
#14237=CARTESIAN_POINT('Ctrl Pts',(-202.495017634632,64.6658938733246,8.59156057778566));
#14238=CARTESIAN_POINT('Ctrl Pts',(-202.527597314898,64.5036191137564,8.58104921543252));
#14239=CARTESIAN_POINT('Ctrl Pts',(-202.691774644925,63.6858751537437,8.52807977583108));
#14240=CARTESIAN_POINT('Ctrl Pts',(-203.301865211552,62.9576565808797,8.47511033622965));
#14241=CARTESIAN_POINT('Ctrl Pts',(-204.078206908466,62.6527747193912,8.42214089662821));
#14242=CARTESIAN_POINT('Ctrl Pts',(-204.85454860538,62.3478928579027,8.36917145702678));
#14243=CARTESIAN_POINT('Ctrl Pts',(-205.797141432581,62.4663477077896,8.31620201742534));
#14244=CARTESIAN_POINT('Ctrl Pts',(-206.473906105662,62.9538402278365,8.2632325778239));
#14245=CARTESIAN_POINT('Ctrl Pts',(-207.150670778743,63.4413327478833,8.21026313822247));
#14246=CARTESIAN_POINT('Ctrl Pts',(-207.561607297705,64.2978629380902,8.15729369862104));
#14247=CARTESIAN_POINT('Ctrl Pts',(-207.518344658731,65.1308021458965,8.1043242590196));
#14248=CARTESIAN_POINT('Ctrl Pts',(-207.475082019757,65.9637413537029,8.05135481941817));
#14249=CARTESIAN_POINT('Ctrl Pts',(-206.977620222847,66.7730895791089,7.99838537981673));
#14250=CARTESIAN_POINT('Ctrl Pts',(-206.253992975692,67.1878461185472,7.94541594021529));
#14251=CARTESIAN_POINT('Ctrl Pts',(-205.530365728537,67.6026026579855,7.89244650061386));
#14252=CARTESIAN_POINT('Ctrl Pts',(-204.580573031136,67.6227675114562,7.83947706101243));
#14253=CARTESIAN_POINT('Ctrl Pts',(-203.83999454816,67.2390972228175,7.78650762141099));
#14254=CARTESIAN_POINT('Ctrl Pts',(-203.099416065183,66.8554269341788,7.73353818180956));
#14255=CARTESIAN_POINT('Ctrl Pts',(-202.568051796631,66.0679215034307,7.68056874220812));
#14256=CARTESIAN_POINT('Ctrl Pts',(-202.489476153733,65.2375690191355,7.62759930260668));
#14257=CARTESIAN_POINT('Ctrl Pts',(-202.482051168863,65.159105077831,7.6225939692351));
#14258=CARTESIAN_POINT('Ctrl Pts',(-202.478669249412,65.0802585442292,7.61758863586352));
#14259=CARTESIAN_POINT('Ctrl Pts',(-202.479185657883,65.0013671530438,7.61258330249194));
#14260=CARTESIAN_POINT('Origin',(-205.,65.,9.));
#14261=CARTESIAN_POINT('',(-202.485705065293,65.0014474068846,6.61258330249194));
#14262=CARTESIAN_POINT('',(-202.485300168502,64.9982947807633,6.88741669750805));
#14263=CARTESIAN_POINT('',(-202.4825,65.,9.));
#14264=CARTESIAN_POINT('Ctrl Pts',(-202.485300168502,64.9982947807633,6.88741669750805));
#14265=CARTESIAN_POINT('Ctrl Pts',(-202.488632032345,65.5341438421791,6.92120310344827));
#14266=CARTESIAN_POINT('Ctrl Pts',(-202.656234597268,66.071895942272,6.9549895093885));
#14267=CARTESIAN_POINT('Ctrl Pts',(-202.972602993533,66.4996100318676,6.98877591532872));
#14268=CARTESIAN_POINT('Ctrl Pts',(-203.468597053612,67.1701689446921,7.04174535493015));
#14269=CARTESIAN_POINT('Ctrl Pts',(-204.330244802095,67.5702638400739,7.09471479453159));
#14270=CARTESIAN_POINT('Ctrl Pts',(-205.162571726307,67.516493453859,7.14768423413302));
#14271=CARTESIAN_POINT('Ctrl Pts',(-205.99489865052,67.4627230676441,7.20065367373446));
#14272=CARTESIAN_POINT('Ctrl Pts',(-206.79790475046,66.9550873998325,7.25362311333589));
#14273=CARTESIAN_POINT('Ctrl Pts',(-207.203496517434,66.2262838036795,7.30659255293733));
#14274=CARTESIAN_POINT('Ctrl Pts',(-207.609088284407,65.4974802075266,7.35956199253877));
#14275=CARTESIAN_POINT('Ctrl Pts',(-207.617265718413,64.5475086830323,7.4125314321402));
#14276=CARTESIAN_POINT('Ctrl Pts',(-207.224280329402,63.8118308682072,7.46550087174164));
#14277=CARTESIAN_POINT('Ctrl Pts',(-206.831294940391,63.0761530533821,7.51847031134307));
#14278=CARTESIAN_POINT('Ctrl Pts',(-206.037146728362,62.5547689482262,7.57143975094451));
#14279=CARTESIAN_POINT('Ctrl Pts',(-205.205868795696,62.4866781128418,7.62440919054594));
#14280=CARTESIAN_POINT('Ctrl Pts',(-204.374590863029,62.4185872774574,7.67737863014738));
#14281=CARTESIAN_POINT('Ctrl Pts',(-203.506183209724,62.8037897118444,7.73034806974881));
#14282=CARTESIAN_POINT('Ctrl Pts',(-202.998719051049,63.4657107727439,7.78331750935025));
#14283=CARTESIAN_POINT('Ctrl Pts',(-202.666284554637,63.8993283805738,7.81801723873618));
#14284=CARTESIAN_POINT('Ctrl Pts',(-202.48874621345,64.4516976821268,7.85271696812212));
#14285=CARTESIAN_POINT('Ctrl Pts',(-202.484985693937,65.0018590734507,7.88741669750805));
#14286=CARTESIAN_POINT('Ctrl Pts',(-202.479185657883,65.0013671530438,7.61258330249194));
#14287=CARTESIAN_POINT('Ctrl Pts',(-202.48413419356,64.2453825289387,7.56461919626208));
#14288=CARTESIAN_POINT('Ctrl Pts',(-202.847051437472,63.4852788025991,7.51665509003223));
#14289=CARTESIAN_POINT('Ctrl Pts',(-203.440577961958,63.0182401939698,7.46869098380237));
#14290=CARTESIAN_POINT('Ctrl Pts',(-204.096042430324,62.5024633909419,7.41572154420094));
#14291=CARTESIAN_POINT('Ctrl Pts',(-205.032758384299,62.3441093227284,7.3627521045995));
#14292=CARTESIAN_POINT('Ctrl Pts',(-205.821340465322,62.615766609253,7.30978266499807));
#14293=CARTESIAN_POINT('Ctrl Pts',(-206.609922546345,62.8874238957777,7.25681322539663));
#14294=CARTESIAN_POINT('Ctrl Pts',(-207.250370754415,63.5890925370406,7.2038437857952));
#14295=CARTESIAN_POINT('Ctrl Pts',(-207.449107210032,64.3991315490894,7.15087434619376));
#14296=CARTESIAN_POINT('Ctrl Pts',(-207.647843665648,65.2091705611382,7.09790490659232));
#14297=CARTESIAN_POINT('Ctrl Pts',(-207.404868368812,66.127579943973,7.04493546699089));
#14298=CARTESIAN_POINT('Ctrl Pts',(-206.831559837749,66.7333659689382,6.99196602738945));
#14299=CARTESIAN_POINT('Ctrl Pts',(-206.258251306687,67.3391519939033,6.93899658778802));
#14300=CARTESIAN_POINT('Ctrl Pts',(-205.354609541398,67.6323146609989,6.88602714818658));
#14301=CARTESIAN_POINT('Ctrl Pts',(-204.534858877184,67.4784698419375,6.83305770858515));
#14302=CARTESIAN_POINT('Ctrl Pts',(-203.715108212969,67.3246250228761,6.78008826898371));
#14303=CARTESIAN_POINT('Ctrl Pts',(-202.979248649829,66.7237727176577,6.72711882938228));
#14304=CARTESIAN_POINT('Ctrl Pts',(-202.66459409923,65.9513402651935,6.67414938978084));
#14305=CARTESIAN_POINT('Ctrl Pts',(-202.542687016746,65.6520756064832,6.65362736068454));
#14306=CARTESIAN_POINT('Ctrl Pts',(-202.48400413857,65.3270562251041,6.63310533158824));
#14307=CARTESIAN_POINT('Ctrl Pts',(-202.485705065293,65.0014474068846,6.61258330249194));
#14308=CARTESIAN_POINT('Origin',(-205.,65.,9.));
#14309=CARTESIAN_POINT('',(-202.484474821952,64.9979518749283,5.61258330249194));
#14310=CARTESIAN_POINT('',(-202.478781766938,64.9989624751798,5.88741669750806));
#14311=CARTESIAN_POINT('',(-202.4825,65.,9.));
#14312=CARTESIAN_POINT('Ctrl Pts',(-202.478781766938,64.9989624751798,5.88741669750806));
#14313=CARTESIAN_POINT('Ctrl Pts',(-202.482826134015,65.7757224753788,5.936719799173));
#14314=CARTESIAN_POINT('Ctrl Pts',(-202.869070859878,66.5559564232876,5.98602290083794));
#14315=CARTESIAN_POINT('Ctrl Pts',(-203.491087909026,67.0204834003828,6.03532600250288));
#14316=CARTESIAN_POINT('Ctrl Pts',(-204.159360155665,67.5195541043661,6.08829544210431));
#14317=CARTESIAN_POINT('Ctrl Pts',(-205.099774104093,67.6542180319002,6.14126488170575));
#14318=CARTESIAN_POINT('Ctrl Pts',(-205.881249255757,67.3627459911589,6.19423432130718));
#14319=CARTESIAN_POINT('Ctrl Pts',(-206.662724407421,67.0712739504177,6.24720376090862));
#14320=CARTESIAN_POINT('Ctrl Pts',(-207.285260762321,66.353665941401,6.30017320051005));
#14321=CARTESIAN_POINT('Ctrl Pts',(-207.463491134351,65.538869465164,6.35314264011149));
#14322=CARTESIAN_POINT('Ctrl Pts',(-207.64172150638,64.724072988927,6.40611207971293));
#14323=CARTESIAN_POINT('Ctrl Pts',(-207.37564589554,63.8120880454697,6.45908151931436));
#14324=CARTESIAN_POINT('Ctrl Pts',(-206.787231874903,63.2209634363394,6.5120509589158));
#14325=CARTESIAN_POINT('Ctrl Pts',(-206.198817854265,62.6298388272089,6.56502039851723));
#14326=CARTESIAN_POINT('Ctrl Pts',(-205.288065423831,62.3595745524054,6.61798983811866));
#14327=CARTESIAN_POINT('Ctrl Pts',(-204.472458408065,62.5340582451549,6.6709592777201));
#14328=CARTESIAN_POINT('Ctrl Pts',(-203.656851392299,62.7085419379043,6.72392871732154));
#14329=CARTESIAN_POINT('Ctrl Pts',(-202.936389791202,63.3277735982066,6.77689815692298));
#14330=CARTESIAN_POINT('Ctrl Pts',(-202.64132917649,64.1079008934913,6.82986759652441));
#14331=CARTESIAN_POINT('Ctrl Pts',(-202.534472133133,64.3904262190013,6.84905063018563));
#14332=CARTESIAN_POINT('Ctrl Pts',(-202.483408423747,64.6940537614417,6.86823366384684));
#14333=CARTESIAN_POINT('Ctrl Pts',(-202.485300168502,64.9982947807633,6.88741669750805));
#14334=CARTESIAN_POINT('Ctrl Pts',(-202.485705065293,65.0014474068846,6.61258330249194));
#14335=CARTESIAN_POINT('Ctrl Pts',(-202.488394403048,64.4866268236333,6.5801358919868));
#14336=CARTESIAN_POINT('Ctrl Pts',(-202.642036120458,63.9703327179061,6.54768848148167));
#14337=CARTESIAN_POINT('Ctrl Pts',(-202.935403348754,63.5520325662536,6.51524107097653));
#14338=CARTESIAN_POINT('Ctrl Pts',(-203.414316686931,62.869169919488,6.4622716313751));
#14339=CARTESIAN_POINT('Ctrl Pts',(-204.265592901342,62.4474572256667,6.40930219177367));
#14340=CARTESIAN_POINT('Ctrl Pts',(-205.099011732569,62.4802052269398,6.35633275217223));
#14341=CARTESIAN_POINT('Ctrl Pts',(-205.932430563797,62.5129532282128,6.30336331257079));
#14342=CARTESIAN_POINT('Ctrl Pts',(-206.747992011841,63.0001619245801,6.25039387296935));
#14343=CARTESIAN_POINT('Ctrl Pts',(-207.1718472666,63.7184975723424,6.19742443336792));
#14344=CARTESIAN_POINT('Ctrl Pts',(-207.595702521358,64.4368332201046,6.14445499376648));
#14345=CARTESIAN_POINT('Ctrl Pts',(-207.62785158283,65.3862958192617,6.09148555416505));
#14346=CARTESIAN_POINT('Ctrl Pts',(-207.253557500899,66.1316570203338,6.03851611456362));
#14347=CARTESIAN_POINT('Ctrl Pts',(-206.879263418968,66.8770182214058,5.98554667496218));
#14348=CARTESIAN_POINT('Ctrl Pts',(-206.098526193634,67.4182780243928,5.93257723536074));
#14349=CARTESIAN_POINT('Ctrl Pts',(-205.26923140592,67.5073259603798,5.87960779575931));
#14350=CARTESIAN_POINT('Ctrl Pts',(-204.439936618207,67.5963738963668,5.82663835615787));
#14351=CARTESIAN_POINT('Ctrl Pts',(-203.562084268114,67.2332099653539,5.77366891655643));
#14352=CARTESIAN_POINT('Ctrl Pts',(-203.038076967138,66.5843064838134,5.720699476955));
#14353=CARTESIAN_POINT('Ctrl Pts',(-202.681559037815,66.1428131589339,5.68466075213398));
#14354=CARTESIAN_POINT('Ctrl Pts',(-202.488836318919,65.5690507238242,5.64862202731296));
#14355=CARTESIAN_POINT('Ctrl Pts',(-202.484474821952,64.9979518749283,5.61258330249194));
#14356=CARTESIAN_POINT('Origin',(-205.,65.,9.));
#14357=CARTESIAN_POINT('',(-202.478344473785,64.9995851075454,4.61258330249193));
#14358=CARTESIAN_POINT('',(-202.48217288036,65.0022992261759,4.88741669750805));
#14359=CARTESIAN_POINT('',(-202.4825,65.,9.));
#14360=CARTESIAN_POINT('Ctrl Pts',(-202.48217288036,65.0022992261759,4.88741669750805));
#14361=CARTESIAN_POINT('Ctrl Pts',(-202.480439771035,65.1896536409608,4.89926705529628));
#14362=CARTESIAN_POINT('Ctrl Pts',(-202.499576724591,65.3766572882651,4.9111174130845));
#14363=CARTESIAN_POINT('Ctrl Pts',(-202.540911860868,65.5586182896119,4.92296777087273));
#14364=CARTESIAN_POINT('Ctrl Pts',(-202.725674130799,66.3719584809291,4.97593721047417));
#14365=CARTESIAN_POINT('Ctrl Pts',(-203.353948275965,67.0845483814278,5.0289066500756));
#14366=CARTESIAN_POINT('Ctrl Pts',(-204.137736939267,67.3697407629541,5.08187608967704));
#14367=CARTESIAN_POINT('Ctrl Pts',(-204.92152560257,67.6549331444803,5.13484552927847));
#14368=CARTESIAN_POINT('Ctrl Pts',(-205.860828784009,67.5127280070342,5.18781496887991));
#14369=CARTESIAN_POINT('Ctrl Pts',(-206.525075154411,67.0083113909224,5.24078440848134));
#14370=CARTESIAN_POINT('Ctrl Pts',(-207.189321524813,66.5038947748106,5.29375384808278));
#14371=CARTESIAN_POINT('Ctrl Pts',(-207.578511084179,65.6372666800331,5.34672328768421));
#14372=CARTESIAN_POINT('Ctrl Pts',(-207.51424151344,64.8056845821744,5.39969272728565));
#14373=CARTESIAN_POINT('Ctrl Pts',(-207.449971942702,63.9741024843156,5.45266216688709));
#14374=CARTESIAN_POINT('Ctrl Pts',(-206.932243241859,63.1775663833756,5.50563160648852));
#14375=CARTESIAN_POINT('Ctrl Pts',(-206.198379354105,62.7812039766656,5.55860104608996));
#14376=CARTESIAN_POINT('Ctrl Pts',(-205.464515466351,62.3848415699556,5.61157048569139));
#14377=CARTESIAN_POINT('Ctrl Pts',(-204.514516391686,62.3886528574756,5.66453992529283));
#14378=CARTESIAN_POINT('Ctrl Pts',(-203.783856396965,62.7908907663254,5.71750936489426));
#14379=CARTESIAN_POINT('Ctrl Pts',(-203.053196402243,63.1931286751752,5.7704788044957));
#14380=CARTESIAN_POINT('Ctrl Pts',(-202.541875487466,63.9937932053548,5.82344824409714));
#14381=CARTESIAN_POINT('Ctrl Pts',(-202.484280302502,64.8258642106609,5.87641768369857));
#14382=CARTESIAN_POINT('Ctrl Pts',(-202.48029378852,64.8834569191276,5.88008402163507));
#14383=CARTESIAN_POINT('Ctrl Pts',(-202.478481014735,64.9412000918792,5.88375035957156));
#14384=CARTESIAN_POINT('Ctrl Pts',(-202.478781766938,64.9989624751798,5.88741669750806));
#14385=CARTESIAN_POINT('Ctrl Pts',(-202.484474821952,64.9979518749283,5.61258330249194));
#14386=CARTESIAN_POINT('Ctrl Pts',(-202.482425824339,64.7296540433568,5.59565258771152));
#14387=CARTESIAN_POINT('Ctrl Pts',(-202.521949050352,64.4619440780171,5.57872187293111));
#14388=CARTESIAN_POINT('Ctrl Pts',(-202.605591636875,64.208812530353,5.5617911581507));
#14389=CARTESIAN_POINT('Ctrl Pts',(-202.86727585945,63.4168650905012,5.50882171854926));
#14390=CARTESIAN_POINT('Ctrl Pts',(-203.560806556459,62.7676132428658,5.45585227894782));
#14391=CARTESIAN_POINT('Ctrl Pts',(-204.368273132118,62.5586704061261,5.40288283934639));
#14392=CARTESIAN_POINT('Ctrl Pts',(-205.175739707778,62.3497275693864,5.34991339974495));
#14393=CARTESIAN_POINT('Ctrl Pts',(-206.097142162087,62.5810937435424,5.29694396014351));
#14394=CARTESIAN_POINT('Ctrl Pts',(-206.710114759154,63.1467119673268,5.24397452054208));
#14395=CARTESIAN_POINT('Ctrl Pts',(-207.323087356221,63.7123301911111,5.19100508094064));
#14396=CARTESIAN_POINT('Ctrl Pts',(-207.627630096046,64.6122004645237,5.13803564133921));
#14397=CARTESIAN_POINT('Ctrl Pts',(-207.484142288597,65.4338272830649,5.08506620173777));
#14398=CARTESIAN_POINT('Ctrl Pts',(-207.340654481149,66.255454101606,5.03209676213634));
#14399=CARTESIAN_POINT('Ctrl Pts',(-206.749136126427,66.9988374652756,4.9791273225349));
#14400=CARTESIAN_POINT('Ctrl Pts',(-205.980735932599,67.3232145944874,4.92615788293347));
#14401=CARTESIAN_POINT('Ctrl Pts',(-205.21233573877,67.6475917236993,4.87318844333203));
#14402=CARTESIAN_POINT('Ctrl Pts',(-204.267053705834,67.5529626184535,4.82021900373059));
#14403=CARTESIAN_POINT('Ctrl Pts',(-203.578201835077,67.082704731772,4.76724956412916));
#14404=CARTESIAN_POINT('Ctrl Pts',(-202.907738863261,66.6250003781818,4.71569414358342));
#14405=CARTESIAN_POINT('Ctrl Pts',(-202.48019798657,65.811454380222,4.66413872303768));
#14406=CARTESIAN_POINT('Ctrl Pts',(-202.478344473785,64.9995851075454,4.61258330249193));
#14407=CARTESIAN_POINT('Origin',(-205.,65.,9.));
#14408=CARTESIAN_POINT('',(-202.483242841669,65.0022852126429,3.61258330249194));
#14409=CARTESIAN_POINT('',(-202.486532959272,64.9997695214146,3.88741669750805));
#14410=CARTESIAN_POINT('',(-202.4825,65.,9.));
#14411=CARTESIAN_POINT('Ctrl Pts',(-202.486532959272,64.9997695214146,3.88741669750805));
#14412=CARTESIAN_POINT('Ctrl Pts',(-202.486887346168,65.4343411087312,3.914783751021));
#14413=CARTESIAN_POINT('Ctrl Pts',(-202.593847191985,65.8690761086745,3.94215080453394));
#14414=CARTESIAN_POINT('Ctrl Pts',(-202.80641367505,66.2439243966071,3.96951785804689));
#14415=CARTESIAN_POINT('Ctrl Pts',(-203.217840045108,66.9694502095321,4.02248729764833));
#14416=CARTESIAN_POINT('Ctrl Pts',(-204.024893383128,67.4706265032263,4.07545673724976));
#14417=CARTESIAN_POINT('Ctrl Pts',(-204.857624949113,67.517716865417,4.12842617685119));
#14418=CARTESIAN_POINT('Ctrl Pts',(-205.690356515098,67.5648072276077,4.18139561645263));
#14419=CARTESIAN_POINT('Ctrl Pts',(-206.548766309047,67.1578116582949,4.23436505605407));
#14420=CARTESIAN_POINT('Ctrl Pts',(-207.03936407854,66.4832946520063,4.2873344956555));
#14421=CARTESIAN_POINT('Ctrl Pts',(-207.529961848034,65.8087776457177,4.34030393525694));
#14422=CARTESIAN_POINT('Ctrl Pts',(-207.652747593072,64.8667392024533,4.39327337485837));
#14423=CARTESIAN_POINT('Ctrl Pts',(-207.351437014309,64.0890044801174,4.44624281445981));
#14424=CARTESIAN_POINT('Ctrl Pts',(-207.050126435545,63.3112697577815,4.49921225406124));
#14425=CARTESIAN_POINT('Ctrl Pts',(-206.32471953298,62.6978387563742,4.55218169366268));
#14426=CARTESIAN_POINT('Ctrl Pts',(-205.507738776886,62.5299048188465,4.60515113326412));
#14427=CARTESIAN_POINT('Ctrl Pts',(-204.690758020792,62.3619708813189,4.65812057286555));
#14428=CARTESIAN_POINT('Ctrl Pts',(-203.782203411168,62.639534007671,4.71109001246699));
#14429=CARTESIAN_POINT('Ctrl Pts',(-203.198551303705,63.2353608119149,4.76405945206842));
#14430=CARTESIAN_POINT('Ctrl Pts',(-202.745474228738,63.6978888525088,4.80517853388163));
#14431=CARTESIAN_POINT('Ctrl Pts',(-202.488186526988,64.3522056469539,4.84629761569484));
#14432=CARTESIAN_POINT('Ctrl Pts',(-202.48217288036,65.0022992261759,4.88741669750805));
#14433=CARTESIAN_POINT('Ctrl Pts',(-202.478344473785,64.9995851075454,4.61258330249193));
#14434=CARTESIAN_POINT('Ctrl Pts',(-202.478293637183,64.9773178345769,4.61116928343624));
#14435=CARTESIAN_POINT('Ctrl Pts',(-202.47856302365,64.955051822924,4.60975526438055));
#14436=CARTESIAN_POINT('Ctrl Pts',(-202.479156404012,64.9327944489305,4.60834124532485));
#14437=CARTESIAN_POINT('Ctrl Pts',(-202.501384552282,64.0990287208875,4.55537180572342));
#14438=CARTESIAN_POINT('Ctrl Pts',(-202.9782625574,63.2773839329187,4.50240236612198));
#14439=CARTESIAN_POINT('Ctrl Pts',(-203.691192206802,62.8444974641621,4.44943292652054));
#14440=CARTESIAN_POINT('Ctrl Pts',(-204.404121856204,62.4116109954056,4.39646348691911));
#14441=CARTESIAN_POINT('Ctrl Pts',(-205.353103149889,62.3674828458613,4.34349404731767));
#14442=CARTESIAN_POINT('Ctrl Pts',(-206.10312836612,62.7323411126537,4.29052460771624));
#14443=CARTESIAN_POINT('Ctrl Pts',(-206.853153582352,63.0971993794462,4.23755516811481));
#14444=CARTESIAN_POINT('Ctrl Pts',(-207.404222721129,63.8710440625754,4.18458572851337));
#14445=CARTESIAN_POINT('Ctrl Pts',(-207.503728768821,64.6991490838892,4.13161628891193));
#14446=CARTESIAN_POINT('Ctrl Pts',(-207.603234816513,65.5272541052031,4.0786468493105));
#14447=CARTESIAN_POINT('Ctrl Pts',(-207.251177773121,66.4096194647016,4.02567740970906));
#14448=CARTESIAN_POINT('Ctrl Pts',(-206.608938619917,66.941773812509,3.97270797010763));
#14449=CARTESIAN_POINT('Ctrl Pts',(-205.966699466714,67.4739281603165,3.91973853050619));
#14450=CARTESIAN_POINT('Ctrl Pts',(-205.034278203699,67.6558714964329,3.86676909090476));
#14451=CARTESIAN_POINT('Ctrl Pts',(-204.239091527064,67.4042020125377,3.81379965130332));
#14452=CARTESIAN_POINT('Ctrl Pts',(-203.44390485043,67.1525325286424,3.76083021170188));
#14453=CARTESIAN_POINT('Ctrl Pts',(-202.785952760175,66.4672502247354,3.70786077210045));
#14454=CARTESIAN_POINT('Ctrl Pts',(-202.566836817648,65.6624846789204,3.65489133249901));
#14455=CARTESIAN_POINT('Ctrl Pts',(-202.508499004114,65.4482224859956,3.64078865582999));
#14456=CARTESIAN_POINT('Ctrl Pts',(-202.481267947496,65.2254907625162,3.62668597916096));
#14457=CARTESIAN_POINT('Ctrl Pts',(-202.483242841669,65.0022852126429,3.61258330249194));
#14458=CARTESIAN_POINT('Origin',(-205.,65.,9.));
#14459=CARTESIAN_POINT('',(-202.486313063014,64.9991964084992,2.61258330249194));
#14460=CARTESIAN_POINT('',(-202.481325106597,64.9978038277911,2.88741669750805));
#14461=CARTESIAN_POINT('',(-202.4825,65.,9.));
#14462=CARTESIAN_POINT('Ctrl Pts',(-202.481325106597,64.9978038277911,2.88741669750805));
#14463=CARTESIAN_POINT('Ctrl Pts',(-202.487529301803,65.6752106759204,2.93030044674572));
#14464=CARTESIAN_POINT('Ctrl Pts',(-202.769932098234,66.3571775427947,2.97318419598338));
#14465=CARTESIAN_POINT('Ctrl Pts',(-203.258234527699,66.8235739378454,3.01606794522105));
#14466=CARTESIAN_POINT('Ctrl Pts',(-203.861379227138,67.3996605934466,3.06903738482248));
#14467=CARTESIAN_POINT('Ctrl Pts',(-204.778662186319,67.6468543225643,3.12200682442392));
#14468=CARTESIAN_POINT('Ctrl Pts',(-205.589606024052,67.4518429000389,3.17497626402536));
#14469=CARTESIAN_POINT('Ctrl Pts',(-206.400549861785,67.2568314775134,3.22794570362679));
#14470=CARTESIAN_POINT('Ctrl Pts',(-207.10515457807,66.6196149033449,3.28091514322823));
#14471=CARTESIAN_POINT('Ctrl Pts',(-207.38043330801,65.8322896946712,3.33388458282966));
#14472=CARTESIAN_POINT('Ctrl Pts',(-207.65571203795,65.0449644859974,3.3868540224311));
#14473=CARTESIAN_POINT('Ctrl Pts',(-207.501664781545,64.1075306428185,3.43982346203253));
#14474=CARTESIAN_POINT('Ctrl Pts',(-206.988905940528,63.4497025998243,3.49279290163397));
#14475=CARTESIAN_POINT('Ctrl Pts',(-206.47614709951,62.7918745568302,3.5457623412354));
#14476=CARTESIAN_POINT('Ctrl Pts',(-205.604676673879,62.413652314021,3.59873178083684));
#14477=CARTESIAN_POINT('Ctrl Pts',(-204.77397183649,62.4884108339761,3.65170122043828));
#14478=CARTESIAN_POINT('Ctrl Pts',(-203.9432669991,62.5631693539311,3.70467066003971));
#14479=CARTESIAN_POINT('Ctrl Pts',(-203.153327749952,63.0909086366506,3.75764009964115));
#14480=CARTESIAN_POINT('Ctrl Pts',(-202.766257826425,63.8297159440883,3.81060953924258));
#14481=CARTESIAN_POINT('Ctrl Pts',(-202.579170447364,64.1868129810278,3.83621192533107));
#14482=CARTESIAN_POINT('Ctrl Pts',(-202.486201423758,64.5932197422685,3.86181431141956));
#14483=CARTESIAN_POINT('Ctrl Pts',(-202.486532959272,64.9997695214146,3.88741669750805));
#14484=CARTESIAN_POINT('Ctrl Pts',(-202.483242841669,65.0022852126429,3.61258330249194));
#14485=CARTESIAN_POINT('Ctrl Pts',(-202.488685620045,64.3871341036922,3.57371653955953));
#14486=CARTESIAN_POINT('Ctrl Pts',(-202.715960806614,63.7683840689348,3.53484977662712));
#14487=CARTESIAN_POINT('Ctrl Pts',(-203.12527891892,63.313408795753,3.49598301369471));
#14488=CARTESIAN_POINT('Ctrl Pts',(-203.68311675752,62.6933472461235,3.44301357409327));
#14489=CARTESIAN_POINT('Ctrl Pts',(-204.57907222952,62.3774729345875,3.39004413449183));
#14490=CARTESIAN_POINT('Ctrl Pts',(-205.402444353812,62.5105808787203,3.3370746948904));
#14491=CARTESIAN_POINT('Ctrl Pts',(-206.225816478105,62.6436888228531,3.28410525528896));
#14492=CARTESIAN_POINT('Ctrl Pts',(-206.976605254691,63.2257790226548,3.23113581568753));
#14493=CARTESIAN_POINT('Ctrl Pts',(-207.310653303464,63.9900245867847,3.17816637608609));
#14494=CARTESIAN_POINT('Ctrl Pts',(-207.644701352236,64.7542701509147,3.12519693648466));
#14495=CARTESIAN_POINT('Ctrl Pts',(-207.562008673197,65.7006710793728,3.07222749688322));
#14496=CARTESIAN_POINT('Ctrl Pts',(-207.100481129582,66.3954024686292,3.01925805728179));
#14497=CARTESIAN_POINT('Ctrl Pts',(-206.638953585967,67.0901338578856,2.96628861768035));
#14498=CARTESIAN_POINT('Ctrl Pts',(-205.798591177777,67.5331957079404,2.91331917807891));
#14499=CARTESIAN_POINT('Ctrl Pts',(-204.964611334002,67.5214909567086,2.86034973847748));
#14500=CARTESIAN_POINT('Ctrl Pts',(-204.130631490227,67.5097862054768,2.80738029887604));
#14501=CARTESIAN_POINT('Ctrl Pts',(-203.303034210866,67.0433148529584,2.75441085927461));
#14502=CARTESIAN_POINT('Ctrl Pts',(-202.861185469285,66.3359047315519,2.70144141967317));
#14503=CARTESIAN_POINT('Ctrl Pts',(-202.614113147639,65.9403361928114,2.67182204727943));
#14504=CARTESIAN_POINT('Ctrl Pts',(-202.487656913234,65.4694307733786,2.64220267488568));
#14505=CARTESIAN_POINT('Ctrl Pts',(-202.486313063014,64.9991964084992,2.61258330249194));
#14506=CARTESIAN_POINT('Origin',(-205.,65.,9.));
#14507=CARTESIAN_POINT('',(-202.480291681284,64.9980775076607,1.61258330249194));
#14508=CARTESIAN_POINT('',(-202.479332509853,65.0014637523716,1.88741669750805));
#14509=CARTESIAN_POINT('',(-202.4825,65.,9.));
#14510=CARTESIAN_POINT('Ctrl Pts',(-202.479332509853,65.0014637523716,1.88741669750805));
#14511=CARTESIAN_POINT('Ctrl Pts',(-202.478740781633,65.0870774969918,1.892847702869));
#14512=CARTESIAN_POINT('Ctrl Pts',(-202.482723841763,65.1726355357681,1.89827870822995));
#14513=CARTESIAN_POINT('Ctrl Pts',(-202.491463117057,65.2577049615865,1.9037097135909));
#14514=CARTESIAN_POINT('Ctrl Pts',(-202.576698627627,66.0874002966744,1.95667915319234));
#14515=CARTESIAN_POINT('Ctrl Pts',(-203.114364546716,66.8706167924958,2.00964859279377));
#14516=CARTESIAN_POINT('Ctrl Pts',(-203.857997640336,67.2483325642607,2.06261803239521));
#14517=CARTESIAN_POINT('Ctrl Pts',(-204.601630733957,67.6260483360257,2.11558747199664));
#14518=CARTESIAN_POINT('Ctrl Pts',(-205.551231002108,67.5982633837343,2.16855691159808));
#14519=CARTESIAN_POINT('Ctrl Pts',(-206.271507076716,67.1777140868197,2.22152635119952));
#14520=CARTESIAN_POINT('Ctrl Pts',(-206.991783151323,66.7571647899052,2.27449579080095));
#14521=CARTESIAN_POINT('Ctrl Pts',(-207.482735032387,65.9438511483675,2.32746523040239));
#14522=CARTESIAN_POINT('Ctrl Pts',(-207.519313078463,65.1105916328361,2.38043467000382));
#14523=CARTESIAN_POINT('Ctrl Pts',(-207.555891124539,64.2773321173047,2.43340410960526));
#14524=CARTESIAN_POINT('Ctrl Pts',(-207.138095335629,63.4241267277794,2.48637354920669));
#14525=CARTESIAN_POINT('Ctrl Pts',(-206.457440987349,62.9420800261392,2.53934298880813));
#14526=CARTESIAN_POINT('Ctrl Pts',(-205.776786639069,62.460033324499,2.59231242840957));
#14527=CARTESIAN_POINT('Ctrl Pts',(-204.83327373142,62.3491453107438,2.645281868011));
#14528=CARTESIAN_POINT('Ctrl Pts',(-204.059403298444,62.660246440714,2.69825130761244));
#14529=CARTESIAN_POINT('Ctrl Pts',(-203.285532865468,62.9713475706841,2.75122074721387));
#14530=CARTESIAN_POINT('Ctrl Pts',(-202.681304907167,63.7044378443795,2.80419018681531));
#14531=CARTESIAN_POINT('Ctrl Pts',(-202.523694147865,64.5234727722695,2.85715962641674));
#14532=CARTESIAN_POINT('Ctrl Pts',(-202.493684139673,64.6794218014072,2.86724531678051));
#14533=CARTESIAN_POINT('Ctrl Pts',(-202.479865961982,64.8384867008611,2.87733100714428));
#14534=CARTESIAN_POINT('Ctrl Pts',(-202.481325106597,64.9978038277911,2.88741669750805));
#14535=CARTESIAN_POINT('Ctrl Pts',(-202.486313063014,64.9991964084992,2.61258330249194));
#14536=CARTESIAN_POINT('Ctrl Pts',(-202.485253655255,64.6284929419525,2.58923323528425));
#14537=CARTESIAN_POINT('Ctrl Pts',(-202.561948628095,64.2582065199014,2.56588316807656));
#14538=CARTESIAN_POINT('Ctrl Pts',(-202.718600866576,63.9255759514543,2.54253310086887));
#14539=CARTESIAN_POINT('Ctrl Pts',(-203.073965209252,63.1710061830575,2.48956366126743));
#14540=CARTESIAN_POINT('Ctrl Pts',(-203.840794098404,62.6102155365585,2.43659422166599));
#14541=CARTESIAN_POINT('Ctrl Pts',(-204.667577479677,62.5002671884707,2.38362478206456));
#14542=CARTESIAN_POINT('Ctrl Pts',(-205.49436086095,62.3903188403828,2.33065534246312));
#14543=CARTESIAN_POINT('Ctrl Pts',(-206.381098734343,62.7312127907059,2.27768590286169));
#14544=CARTESIAN_POINT('Ctrl Pts',(-206.92131536661,63.366685408653,2.22471646326025));
#14545=CARTESIAN_POINT('Ctrl Pts',(-207.461531998877,64.0021580266001,2.17174702365882));
#14546=CARTESIAN_POINT('Ctrl Pts',(-207.655227390017,64.932209312171,2.11877758405738));
#14547=CARTESIAN_POINT('Ctrl Pts',(-207.413612753018,65.7305084368602,2.06580814445595));
#14548=CARTESIAN_POINT('Ctrl Pts',(-207.171998116018,66.5288075615494,2.01283870485451));
#14549=CARTESIAN_POINT('Ctrl Pts',(-206.495073450879,67.1953545253569,1.95986926525307));
#14550=CARTESIAN_POINT('Ctrl Pts',(-205.693137039763,67.4246089886848,1.90689982565164));
#14551=CARTESIAN_POINT('Ctrl Pts',(-204.891200628647,67.6538634520127,1.8539303860502));
#14552=CARTESIAN_POINT('Ctrl Pts',(-203.964252471554,67.4458254148609,1.80096094644877));
#14553=CARTESIAN_POINT('Ctrl Pts',(-203.337200838176,66.8958561611357,1.74799150684733));
#14554=CARTESIAN_POINT('Ctrl Pts',(-202.802880568774,66.4272189641786,1.70285543872887));
#14555=CARTESIAN_POINT('Ctrl Pts',(-202.486315293188,65.710305364988,1.6577193706104));
#14556=CARTESIAN_POINT('Ctrl Pts',(-202.480291681284,64.9980775076607,1.61258330249194));
#14557=CARTESIAN_POINT('Origin',(-205.,65.,9.));
#14558=CARTESIAN_POINT('',(-202.480232429385,65.0018635099461,0.612583302491936));
#14559=CARTESIAN_POINT('',(-202.485823128102,65.0013539996937,0.887416697508052));
#14560=CARTESIAN_POINT('',(-202.4825,65.,9.));
#14561=CARTESIAN_POINT('',(-206.913465996665,66.6359872033749,0.));
#14562=CARTESIAN_POINT('Ctrl Pts',(-202.480232429385,65.0018635099461,0.612583302491936));
#14563=CARTESIAN_POINT('Ctrl Pts',(-202.486197578718,64.2874572406361,0.567297187132251));
#14564=CARTESIAN_POINT('Ctrl Pts',(-202.805075480509,63.5684921698319,0.522011071772566));
#14565=CARTESIAN_POINT('Ctrl Pts',(-203.34253206956,63.09963781157,0.476724956412881));
#14566=CARTESIAN_POINT('Ctrl Pts',(-203.971174515616,62.55123677486,0.423755516811446));
#14567=CARTESIAN_POINT('Ctrl Pts',(-204.898856375572,62.3450143916412,0.370786077210011));
#14568=CARTESIAN_POINT('Ctrl Pts',(-205.700051205779,62.576961421545,0.317816637608576));
#14569=CARTESIAN_POINT('Ctrl Pts',(-206.501246035986,62.8089084514488,0.264847198007142));
#14570=CARTESIAN_POINT('Ctrl Pts',(-207.175953836445,63.4790248944752,0.211877758405707));
#14571=CARTESIAN_POINT('Ctrl Pts',(-207.415129834976,64.2765861727607,0.158908318804272));
#14572=CARTESIAN_POINT('Ctrl Pts',(-207.654305833508,65.0741474510461,0.105938879202837));
#14573=CARTESIAN_POINT('Ctrl Pts',(-207.457950030113,65.9991535645905,0.0529694396014022));
#14574=CARTESIAN_POINT('Ctrl Pts',(-206.913465996665,66.635987203375,-3.2665312349373E-14));
#14575=CARTESIAN_POINT('',(-203.082854885701,66.6387832991579,-5.61437644333811E-15));
#14576=CARTESIAN_POINT('Origin',(-205.,65.,0.));
#14577=CARTESIAN_POINT('Ctrl Pts',(-203.082851846776,66.6387856087132,-3.81639164714898E-15));
#14578=CARTESIAN_POINT('Ctrl Pts',(-203.61482262847,67.259363488501,0.0519060689145044));
#14579=CARTESIAN_POINT('Ctrl Pts',(-204.477412313746,67.5988757717313,0.103812137829013));
#14580=CARTESIAN_POINT('Ctrl Pts',(-205.2894785266,67.5049507621395,0.155718206743521));
#14581=CARTESIAN_POINT('Ctrl Pts',(-206.118181087084,67.4091015632562,0.208687646344957));
#14582=CARTESIAN_POINT('Ctrl Pts',(-206.894268878324,66.8618739841832,0.261657085946393));
#14583=CARTESIAN_POINT('Ctrl Pts',(-207.26249802366,66.113605339536,0.314626525547829));
#14584=CARTESIAN_POINT('Ctrl Pts',(-207.630727168995,65.3653366948888,0.367595965149265));
#14585=CARTESIAN_POINT('Ctrl Pts',(-207.591097668426,64.4160269846675,0.420565404750701));
#14586=CARTESIAN_POINT('Ctrl Pts',(-207.161527535563,63.7010804522683,0.473534844352138));
#14587=CARTESIAN_POINT('Ctrl Pts',(-206.7319574027,62.9861339198691,0.526504283953574));
#14588=CARTESIAN_POINT('Ctrl Pts',(-205.912446637543,62.5055505652921,0.57947372355501));
#14589=CARTESIAN_POINT('Ctrl Pts',(-205.078774815322,62.4795076113936,0.632443163156446));
#14590=CARTESIAN_POINT('Ctrl Pts',(-204.245102993101,62.4534646574951,0.685412602757882));
#14591=CARTESIAN_POINT('Ctrl Pts',(-203.397270113817,62.881962104275,0.738382042359318));
#14592=CARTESIAN_POINT('Ctrl Pts',(-202.923859535018,63.5686371622738,0.791351481960754));
#14593=CARTESIAN_POINT('Ctrl Pts',(-202.637667536784,63.9837544321181,0.82337322047652));
#14594=CARTESIAN_POINT('Ctrl Pts',(-202.488311662699,64.4932251195213,0.855394958992286));
#14595=CARTESIAN_POINT('Ctrl Pts',(-202.485823128102,65.0013539996937,0.887416697508052));
#14596=CARTESIAN_POINT('Origin',(-205.,65.,-2.20842344717744));
#14597=CARTESIAN_POINT('',(-201.921327255612,65.0000400816385,16.2084234471775));
#14598=CARTESIAN_POINT('',(-201.931378751613,65.000780661492,16.2915765528226));
#14599=CARTESIAN_POINT('',(-201.9265,65.0000000000003,-2.20842344717744));
#14600=CARTESIAN_POINT('',(-205.793799282533,62.0307770462544,17.));
#14601=CARTESIAN_POINT('Ctrl Pts',(-201.931378751613,65.000780661492,16.2915765528226));
#14602=CARTESIAN_POINT('Ctrl Pts',(-201.930449348459,65.4711429475139,16.315839943476));
#14603=CARTESIAN_POINT('Ctrl Pts',(-202.253363219044,66.967050695802,16.3930727737308));
#14604=CARTESIAN_POINT('Ctrl Pts',(-204.58235401933,68.6092464457014,16.5232750435871));
#14605=CARTESIAN_POINT('Ctrl Pts',(-207.810233494003,67.3070985281123,16.6821833623914));
#14606=CARTESIAN_POINT('Ctrl Pts',(-208.456478816595,63.8847024923042,16.8410916811957));
#14607=CARTESIAN_POINT('Ctrl Pts',(-206.782006578242,62.2949667869872,16.9470305603986));
#14608=CARTESIAN_POINT('Ctrl Pts',(-205.793799282533,62.0307770462544,17.));
#14609=CARTESIAN_POINT('',(-204.206200717467,62.0307770462543,17.));
#14610=CARTESIAN_POINT('Origin',(-205.,65.,17.));
#14611=CARTESIAN_POINT('Ctrl Pts',(-201.921327255612,65.0000400816385,16.2084234471775));
#14612=CARTESIAN_POINT('Ctrl Pts',(-201.921327064386,65.0014822929036,16.2084984707981));
#14613=CARTESIAN_POINT('Ctrl Pts',(-201.921978896747,66.0211785478221,16.2615429340201));
#14614=CARTESIAN_POINT('Ctrl Pts',(-203.036142251593,68.0574739112173,16.3675568368436));
#14615=CARTESIAN_POINT('Ctrl Pts',(-206.506722984033,68.3070966859805,16.5264651556479));
#14616=CARTESIAN_POINT('Ctrl Pts',(-208.595801399242,65.5239883392264,16.6853734744522));
#14617=CARTESIAN_POINT('Ctrl Pts',(-207.396687980664,62.2840121808758,16.8432184225696));
#14618=CARTESIAN_POINT('Ctrl Pts',(-205.168807349915,61.7689270476826,16.9480939310855));
#14619=CARTESIAN_POINT('Ctrl Pts',(-204.204431285565,62.0254151804089,17.));
#14620=CARTESIAN_POINT('Origin',(-205.,65.,-2.20842344717744));
#14621=CARTESIAN_POINT('',(-201.92822561016,65.0026730836673,15.2084234471775));
#14622=CARTESIAN_POINT('',(-201.926883911247,64.9971795384332,15.2915765528226));
#14623=CARTESIAN_POINT('',(-201.9265,65.0000000000003,-2.20842344717744));
#14624=CARTESIAN_POINT('Ctrl Pts',(-201.926883911247,64.9971795384332,15.2915765528226));
#14625=CARTESIAN_POINT('Ctrl Pts',(-201.933858660338,65.7655048517695,15.3313566392007));
#14626=CARTESIAN_POINT('Ctrl Pts',(-202.614666302031,67.5679201912294,15.4241061651802));
#14627=CARTESIAN_POINT('Ctrl Pts',(-205.641600424982,68.5768349043511,15.5698251307612));
#14628=CARTESIAN_POINT('Ctrl Pts',(-208.354330159779,66.3978993048601,15.7287334495655));
#14629=CARTESIAN_POINT('Ctrl Pts',(-207.991779446085,62.9373177297799,15.8876417683699));
#14630=CARTESIAN_POINT('Ctrl Pts',(-204.886538861478,61.3679191982373,16.0465500871742));
#14631=CARTESIAN_POINT('Ctrl Pts',(-202.343324158449,62.8593293585014,16.1811950153251));
#14632=CARTESIAN_POINT('Ctrl Pts',(-201.932478329689,64.4442944309099,16.2628705038745));
#14633=CARTESIAN_POINT('Ctrl Pts',(-201.931378751613,65.000780661492,16.2915765528226));
#14634=CARTESIAN_POINT('Ctrl Pts',(-201.92822561016,65.0026730836673,15.2084234471775));
#14635=CARTESIAN_POINT('Ctrl Pts',(-201.925723697844,65.3041504713038,15.2240151665228));
#14636=CARTESIAN_POINT('Ctrl Pts',(-202.105046276089,66.6269190709931,15.2925763254696));
#14637=CARTESIAN_POINT('Ctrl Pts',(-204.001159776429,68.4939639011247,15.4141069240177));
#14638=CARTESIAN_POINT('Ctrl Pts',(-207.396164892643,67.7320116880119,15.5730152428221));
#14639=CARTESIAN_POINT('Ctrl Pts',(-208.594390772745,64.4653708967053,15.7319235616264));
#14640=CARTESIAN_POINT('Ctrl Pts',(-206.497323573879,61.6888943200732,15.8908318804307));
#14641=CARTESIAN_POINT('Ctrl Pts',(-203.029156356454,61.9478343561165,16.0496651756144));
#14642=CARTESIAN_POINT('Ctrl Pts',(-201.921462076895,63.9832280166276,16.1555290311966));
#14643=CARTESIAN_POINT('Ctrl Pts',(-201.921327255612,65.0000400816385,16.2084234471775));
#14644=CARTESIAN_POINT('Origin',(-205.,65.,-2.20842344717744));
#14645=CARTESIAN_POINT('',(-201.930818080783,64.9985876483626,14.2084234471775));
#14646=CARTESIAN_POINT('',(-201.921593038638,65.0008245362821,14.2915765528226));
#14647=CARTESIAN_POINT('',(-201.9265,65.0000000000003,-2.20842344717744));
#14648=CARTESIAN_POINT('Ctrl Pts',(-201.921593038638,65.0008245362821,14.2915765528226));
#14649=CARTESIAN_POINT('Ctrl Pts',(-201.921433171929,65.0455751138522,14.293903895324));
#14650=CARTESIAN_POINT('Ctrl Pts',(-201.94260765529,66.108677346403,14.3492006774268));
#14651=CARTESIAN_POINT('Ctrl Pts',(-203.167704085678,68.1381789685902,14.4574668991311));
#14652=CARTESIAN_POINT('Ctrl Pts',(-206.645674046841,68.2399430821141,14.6163752179354));
#14653=CARTESIAN_POINT('Ctrl Pts',(-208.614908869506,65.3713640210235,14.7752835367397));
#14654=CARTESIAN_POINT('Ctrl Pts',(-207.270034749662,62.1623216890685,14.934191855544));
#14655=CARTESIAN_POINT('Ctrl Pts',(-203.844019983521,61.5548329425339,15.0931001743483));
#14656=CARTESIAN_POINT('Ctrl Pts',(-202.070137533967,63.4672306219619,15.2122284067745));
#14657=CARTESIAN_POINT('Ctrl Pts',(-201.92457138662,64.7424361512098,15.2783871995992));
#14658=CARTESIAN_POINT('Ctrl Pts',(-201.926883911247,64.9971795384332,15.2915765528226));
#14659=CARTESIAN_POINT('Ctrl Pts',(-201.930818080783,64.9985876483626,14.2084234471775));
#14660=CARTESIAN_POINT('Ctrl Pts',(-201.93331444443,65.6013705544098,14.2395318622475));
#14661=CARTESIAN_POINT('Ctrl Pts',(-202.396541145728,67.2340750825248,14.323609716919));
#14662=CARTESIAN_POINT('Ctrl Pts',(-205.050996574037,68.6335759662945,14.4606570111919));
#14663=CARTESIAN_POINT('Ctrl Pts',(-208.082122938738,66.9250957063364,14.6195653299962));
#14664=CARTESIAN_POINT('Ctrl Pts',(-208.287593414598,63.4517090773303,14.7784736488005));
#14665=CARTESIAN_POINT('Ctrl Pts',(-205.479035047994,61.3977785533642,14.9373819676048));
#14666=CARTESIAN_POINT('Ctrl Pts',(-202.549962640807,62.5238193976047,15.0806985670638));
#14667=CARTESIAN_POINT('Ctrl Pts',(-201.934223395047,64.2799473079498,15.1710457269214));
#14668=CARTESIAN_POINT('Ctrl Pts',(-201.92822561016,65.0026730836673,15.2084234471775));
#14669=CARTESIAN_POINT('Origin',(-205.,65.,-2.20842344717744));
#14670=CARTESIAN_POINT('',(-201.923049085304,64.9979784157639,13.2084234471775));
#14671=CARTESIAN_POINT('',(-201.929343804705,65.0023490103727,13.2915765528226));
#14672=CARTESIAN_POINT('',(-201.9265,65.0000000000003,-2.20842344717744));
#14673=CARTESIAN_POINT('Ctrl Pts',(-201.929343804705,65.0023490103727,13.2915765528226));
#14674=CARTESIAN_POINT('Ctrl Pts',(-201.926890407685,65.3476938732414,13.3094205910487));
#14675=CARTESIAN_POINT('Ctrl Pts',(-202.140127765787,66.715242629014,13.3802340688762));
#14676=CARTESIAN_POINT('Ctrl Pts',(-204.150352559975,68.5332102455456,13.5040169863053));
#14677=CARTESIAN_POINT('Ctrl Pts',(-207.509958369796,67.627847859619,13.6629253051095));
#14678=CARTESIAN_POINT('Ctrl Pts',(-208.568462405179,64.313303932567,13.8218336239139));
#14679=CARTESIAN_POINT('Ctrl Pts',(-206.355439979715,61.6283152734234,13.9807419427182));
#14680=CARTESIAN_POINT('Ctrl Pts',(-202.950376540163,62.028501342373,14.1373229190211));
#14681=CARTESIAN_POINT('Ctrl Pts',(-201.925071678064,64.0270688070702,14.2409344557225));
#14682=CARTESIAN_POINT('Ctrl Pts',(-201.921593038638,65.0008245362821,14.2915765528226));
#14683=CARTESIAN_POINT('Ctrl Pts',(-201.923049085304,64.9979784157639,13.2084234471775));
#14684=CARTESIAN_POINT('Ctrl Pts',(-201.929872233322,65.8956158856996,13.2550485579722));
#14685=CARTESIAN_POINT('Ctrl Pts',(-202.81779490193,67.8247836690126,13.3546431083684));
#14686=CARTESIAN_POINT('Ctrl Pts',(-206.096501553054,68.4645576101642,13.5072070983661));
#14687=CARTESIAN_POINT('Ctrl Pts',(-208.506291890959,65.9546686696882,13.6661154171704));
#14688=CARTESIAN_POINT('Ctrl Pts',(-207.70155301198,62.5695501611123,13.8250237359747));
#14689=CARTESIAN_POINT('Ctrl Pts',(-204.420060527044,61.4126409040308,13.983932054779));
#14690=CARTESIAN_POINT('Ctrl Pts',(-202.208562006044,63.127226492007,14.1117319585132));
#14691=CARTESIAN_POINT('Ctrl Pts',(-201.929063794464,64.574989986234,14.1865624226461));
#14692=CARTESIAN_POINT('Ctrl Pts',(-201.930818080783,64.9985876483626,14.2084234471775));
#14693=CARTESIAN_POINT('Origin',(-205.,65.,-2.20842344717744));
#14694=CARTESIAN_POINT('',(-201.924541399743,65.0025681720917,12.2084234471775));
#14695=CARTESIAN_POINT('',(-201.930084889885,64.9980134264973,12.2915765528226));
#14696=CARTESIAN_POINT('',(-201.9265,65.0000000000003,-2.20842344717744));
#14697=CARTESIAN_POINT('Ctrl Pts',(-201.930084889885,64.9980134264973,12.2915765528226));
#14698=CARTESIAN_POINT('Ctrl Pts',(-201.933904699482,65.6440526195987,12.3249372867734));
#14699=CARTESIAN_POINT('Ctrl Pts',(-202.449144876912,67.3214312246058,12.4112674603257));
#14700=CARTESIAN_POINT('Ctrl Pts',(-205.205168523821,68.6281374401227,12.5505670734794));
#14701=CARTESIAN_POINT('Ctrl Pts',(-208.161051499856,66.7925481367497,12.7094753922837));
#14702=CARTESIAN_POINT('Ctrl Pts',(-208.218917791317,63.3135707366188,12.868383711088));
#14703=CARTESIAN_POINT('Ctrl Pts',(-205.325716228722,61.3806928361316,13.0272920298923));
#14704=CARTESIAN_POINT('Ctrl Pts',(-202.492315006707,62.6104022255164,13.1683563104705));
#14705=CARTESIAN_POINT('Ctrl Pts',(-201.934173235912,64.3225490252213,13.2564511514473));
#14706=CARTESIAN_POINT('Ctrl Pts',(-201.929343804705,65.0023490103727,13.2915765528226));
#14707=CARTESIAN_POINT('Ctrl Pts',(-201.924541399743,65.0025681720917,12.2084234471775));
#14708=CARTESIAN_POINT('Ctrl Pts',(-201.922957716369,65.1793797916405,12.2175958140955));
#14709=CARTESIAN_POINT('Ctrl Pts',(-202.017351358014,66.3755695754831,12.279737620615));
#14710=CARTESIAN_POINT('Ctrl Pts',(-203.586717704544,68.3478512877946,12.3948488667359));
#14711=CARTESIAN_POINT('Ctrl Pts',(-207.048871778231,68.0012663207677,12.5537571855402));
#14712=CARTESIAN_POINT('Ctrl Pts',(-208.632643105455,64.9031539354061,12.7126655043445));
#14713=CARTESIAN_POINT('Ctrl Pts',(-206.886047834894,61.8938289396112,12.8715738231488));
#14714=CARTESIAN_POINT('Ctrl Pts',(-203.410344989279,61.7322068549995,13.0304821419532));
#14715=CARTESIAN_POINT('Ctrl Pts',(-201.984214525019,63.7348656859119,13.1427653499627));
#14716=CARTESIAN_POINT('Ctrl Pts',(-201.922120652239,64.8758359229873,13.2020791183708));
#14717=CARTESIAN_POINT('Ctrl Pts',(-201.923049085304,64.9979784157639,13.2084234471775));
#14718=CARTESIAN_POINT('Origin',(-205.,65.,-2.20842344717744));
#14719=CARTESIAN_POINT('',(-201.93135070807,65.0005697538699,11.2084234471775));
#14720=CARTESIAN_POINT('',(-201.922104816116,64.9986005640695,11.2915765528226));
#14721=CARTESIAN_POINT('',(-201.9265,65.0000000000003,-2.20842344717744));
#14722=CARTESIAN_POINT('Ctrl Pts',(-201.922104816116,64.9986005640695,11.2915765528226));
#14723=CARTESIAN_POINT('Ctrl Pts',(-201.927430244541,65.9388404453587,11.3404539824981));
#14724=CARTESIAN_POINT('Ctrl Pts',(-202.890890835511,67.9074743145328,11.4423008517751));
#14725=CARTESIAN_POINT('Ctrl Pts',(-206.24255786536,68.4148975619695,11.5971171606536));
#14726=CARTESIAN_POINT('Ctrl Pts',(-208.54365094371,65.80499279292,11.7560254794579));
#14727=CARTESIAN_POINT('Ctrl Pts',(-207.595964443522,62.4570796285605,11.9149337982622));
#14728=CARTESIAN_POINT('Ctrl Pts',(-204.268326756069,61.4404874390394,12.0738421170665));
#14729=CARTESIAN_POINT('Ctrl Pts',(-202.169249555209,63.215545030581,12.1993897019199));
#14730=CARTESIAN_POINT('Ctrl Pts',(-201.92783968982,64.6182857983542,12.271967847172));
#14731=CARTESIAN_POINT('Ctrl Pts',(-201.930084889885,64.9980134264973,12.2915765528226));
#14732=CARTESIAN_POINT('Ctrl Pts',(-201.93135070807,65.0005697538699,11.2084234471775));
#14733=CARTESIAN_POINT('Ctrl Pts',(-201.930559327437,65.4791732627651,11.2331125098202));
#14734=CARTESIAN_POINT('Ctrl Pts',(-202.261422849189,66.9835666250466,11.3107710120644));
#14735=CARTESIAN_POINT('Ctrl Pts',(-204.61202606459,68.6131636161778,11.4413989539101));
#14736=CARTESIAN_POINT('Ctrl Pts',(-207.827214742755,67.2830531947759,11.6003072727144));
#14737=CARTESIAN_POINT('Ctrl Pts',(-208.450444543957,63.859865121617,11.7592155915187));
#14738=CARTESIAN_POINT('Ctrl Pts',(-205.910345352164,61.4819399619076,11.918123910323));
#14739=CARTESIAN_POINT('Ctrl Pts',(-202.730442829122,62.2804204494558,12.0678598622093));
#14740=CARTESIAN_POINT('Ctrl Pts',(-201.932103318763,64.1583115672449,12.1646263744941));
#14741=CARTESIAN_POINT('Ctrl Pts',(-201.924541399743,65.0025681720917,12.2084234471775));
#14742=CARTESIAN_POINT('Origin',(-205.,65.,-2.20842344717744));
#14743=CARTESIAN_POINT('',(-201.926636332893,64.997176114423,10.2084234471775));
#14744=CARTESIAN_POINT('',(-201.925849963783,65.0027879232472,10.2915765528225));
#14745=CARTESIAN_POINT('',(-201.9265,65.0000000000003,-2.20842344717744));
#14746=CARTESIAN_POINT('Ctrl Pts',(-201.925849963783,65.0027879232472,10.2915765528226));
#14747=CARTESIAN_POINT('Ctrl Pts',(-201.923807784004,65.2232580373303,10.3030012386214));
#14748=CARTESIAN_POINT('Ctrl Pts',(-202.046104360132,66.4636685168287,10.3673953640217));
#14749=CARTESIAN_POINT('Ctrl Pts',(-203.730082217424,68.4048177973288,10.4847589290234));
#14750=CARTESIAN_POINT('Ctrl Pts',(-207.174406712011,67.9116027988503,10.6436672478277));
#14751=CARTESIAN_POINT('Ctrl Pts',(-208.625259435921,64.7490628967685,10.802575566632));
#14752=CARTESIAN_POINT('Ctrl Pts',(-206.752514827754,61.816579326257,10.9614838854363));
#14753=CARTESIAN_POINT('Ctrl Pts',(-203.273084212998,61.8026202489985,11.1203922042406));
#14754=CARTESIAN_POINT('Ctrl Pts',(-201.9601129259,63.8226531889706,11.2304230933694));
#14755=CARTESIAN_POINT('Ctrl Pts',(-201.921658972173,64.9198838444615,11.2874845428967));
#14756=CARTESIAN_POINT('Ctrl Pts',(-201.922104816116,64.9986005640695,11.2915765528226));
#14757=CARTESIAN_POINT('Ctrl Pts',(-201.926636332893,64.997176114423,10.2084234471775));
#14758=CARTESIAN_POINT('Ctrl Pts',(-201.933743017009,65.7735626620793,10.248629205545));
#14759=CARTESIAN_POINT('Ctrl Pts',(-202.626478224698,67.5840970922976,10.3418044035139));
#14760=CARTESIAN_POINT('Ctrl Pts',(-205.670288190648,68.5715807191365,10.4879490410843));
#14761=CARTESIAN_POINT('Ctrl Pts',(-208.365419479959,66.3709218853546,10.6468573598885));
#14762=CARTESIAN_POINT('Ctrl Pts',(-207.975171804641,62.9134171895902,10.8057656786929));
#14763=CARTESIAN_POINT('Ctrl Pts',(-204.857319871709,61.3688682931048,10.9646739974972));
#14764=CARTESIAN_POINT('Ctrl Pts',(-202.334362743788,62.8760590219367,11.0988932536587));
#14765=CARTESIAN_POINT('Ctrl Pts',(-201.932257204317,64.45234773989,11.1801430702188));
#14766=CARTESIAN_POINT('Ctrl Pts',(-201.93135070807,65.0005697538699,11.2084234471775));
#14767=CARTESIAN_POINT('Origin',(-205.,65.,-2.20842344717744));
#14768=CARTESIAN_POINT('',(-201.921694845227,65.0009686859934,9.20842344717746));
#14769=CARTESIAN_POINT('',(-201.931440657504,64.9998541967196,9.29157655282255));
#14770=CARTESIAN_POINT('',(-201.9265,65.0000000000003,-2.20842344717744));
#14771=CARTESIAN_POINT('Ctrl Pts',(-201.931440657504,64.9998541967196,9.29157655282255));
#14772=CARTESIAN_POINT('Ctrl Pts',(-201.931661291496,65.5221576605085,9.31851793434613));
#14773=CARTESIAN_POINT('Ctrl Pts',(-202.306392258298,67.071658817483,9.39842875547113));
#14774=CARTESIAN_POINT('Ctrl Pts',(-204.765727205063,68.6263744518545,9.53130901619758));
#14775=CARTESIAN_POINT('Ctrl Pts',(-207.921565600238,67.1610020478975,9.69021733500189));
#14776=CARTESIAN_POINT('Ctrl Pts',(-208.398945306849,63.714447119501,9.84912565380619));
#14777=CARTESIAN_POINT('Ctrl Pts',(-205.76020994545,61.4464727035873,10.0080339726105));
#14778=CARTESIAN_POINT('Ctrl Pts',(-202.664341261103,62.3651666064549,10.1555176056159));
#14779=CARTESIAN_POINT('Ctrl Pts',(-201.933276151044,64.2010698916383,10.25003179902));
#14780=CARTESIAN_POINT('Ctrl Pts',(-201.925849963783,65.0027879232472,10.2915765528226));
#14781=CARTESIAN_POINT('Ctrl Pts',(-201.921694845227,65.0009686859933,9.20842344717746));
#14782=CARTESIAN_POINT('Ctrl Pts',(-201.921476487875,65.0539088334071,9.21117646166824));
#14783=CARTESIAN_POINT('Ctrl Pts',(-201.94672114028,66.12523254833,9.26689891576045));
#14784=CARTESIAN_POINT('Ctrl Pts',(-203.192942654321,68.1527795421275,9.37559080945409));
#14785=CARTESIAN_POINT('Ctrl Pts',(-206.671617316371,68.2266345686238,9.5344991282584));
#14786=CARTESIAN_POINT('Ctrl Pts',(-208.617771906093,65.3423470860332,9.69340744706271));
#14787=CARTESIAN_POINT('Ctrl Pts',(-207.247193647397,62.1441996213101,9.85231576586701));
#14788=CARTESIAN_POINT('Ctrl Pts',(-203.816413369187,61.5642180250794,10.0112240846713));
#14789=CARTESIAN_POINT('Ctrl Pts',(-202.064218289351,63.4839054024564,10.1299266451081));
#14790=CARTESIAN_POINT('Ctrl Pts',(-201.924380251815,64.7507051905809,10.1956597659435));
#14791=CARTESIAN_POINT('Ctrl Pts',(-201.926636332893,64.997176114423,10.2084234471775));
#14792=CARTESIAN_POINT('Origin',(-205.,65.,-2.20842344717744));
#14793=CARTESIAN_POINT('',(-201.92953466944,65.0022696572995,8.20842344717746));
#14794=CARTESIAN_POINT('',(-201.925313606426,64.9972772118362,8.29157655282255));
#14795=CARTESIAN_POINT('',(-201.9265,65.0000000000003,-2.20842344717744));
#14796=CARTESIAN_POINT('Ctrl Pts',(-201.925313606426,64.9972772118362,8.29157655282255));
#14797=CARTESIAN_POINT('Ctrl Pts',(-201.932861274056,65.8162531240691,8.33403463007084));
#14798=CARTESIAN_POINT('Ctrl Pts',(-202.690778828862,67.6692927338958,8.42946214692057));
#14799=CARTESIAN_POINT('Ctrl Pts',(-205.821270877028,68.5399137777715,8.57785910337175));
#14800=CARTESIAN_POINT('Ctrl Pts',(-208.420572279286,66.2268499051207,8.73676742217605));
#14801=CARTESIAN_POINT('Ctrl Pts',(-207.883931246923,62.7890237517031,8.89567574098036));
#14802=CARTESIAN_POINT('Ctrl Pts',(-204.703334280485,61.3781959110996,9.05458405978466));
#14803=CARTESIAN_POINT('Ctrl Pts',(-202.287845274185,62.9640429293115,9.1865509970654));
#14804=CARTESIAN_POINT('Ctrl Pts',(-201.931227503092,64.4952570260857,9.26554849474469));
#14805=CARTESIAN_POINT('Ctrl Pts',(-201.931440657504,64.9998541967196,9.29157655282255));
#14806=CARTESIAN_POINT('Ctrl Pts',(-201.92953466944,65.0022696572995,8.20842344717746));
#14807=CARTESIAN_POINT('Ctrl Pts',(-201.927117444002,65.3559080588384,8.22669315739295));
#14808=CARTESIAN_POINT('Ctrl Pts',(-202.147019533078,66.7319379190628,8.29793230720988));
#14809=CARTESIAN_POINT('Ctrl Pts',(-204.178729132788,68.5399137354599,8.42214089662826));
#14810=CARTESIAN_POINT('Ctrl Pts',(-207.530962455862,67.6076242326776,8.58104921543256));
#14811=CARTESIAN_POINT('Ctrl Pts',(-208.562837687446,64.2846939782535,8.73995753423686));
#14812=CARTESIAN_POINT('Ctrl Pts',(-206.328343148279,61.6175482897389,8.89886585304117));
#14813=CARTESIAN_POINT('Ctrl Pts',(-202.935848069069,62.0438803005006,9.0550211573547));
#14814=CARTESIAN_POINT('Ctrl Pts',(-201.925677797602,64.0353126907724,9.1582070220668));
#14815=CARTESIAN_POINT('Ctrl Pts',(-201.921694845227,65.0009686859933,9.20842344717746));
#14816=CARTESIAN_POINT('Origin',(-205.,65.,-2.20842344717744));
#14817=CARTESIAN_POINT('',(-201.929918596978,64.9979181762371,7.20842344717746));
#14818=CARTESIAN_POINT('',(-201.922453672097,65.0016690942922,7.29157655282255));
#14819=CARTESIAN_POINT('',(-201.9265,65.0000000000003,-2.20842344717744));
#14820=CARTESIAN_POINT('Ctrl Pts',(-201.922453672097,65.0016690942922,7.29157655282255));
#14821=CARTESIAN_POINT('Ctrl Pts',(-201.921823212738,65.0979839665099,7.29658188619413));
#14822=CARTESIAN_POINT('Ctrl Pts',(-201.969645797573,66.2129262637451,7.35455665916715));
#14823=CARTESIAN_POINT('Ctrl Pts',(-203.328382663649,68.2266346071907,7.4655008717416));
#14824=CARTESIAN_POINT('Ctrl Pts',(-206.807057367278,68.1527795798118,7.62440919054589));
#14825=CARTESIAN_POINT('Ctrl Pts',(-208.629042073693,65.1884914716269,7.78331750935022));
#14826=CARTESIAN_POINT('Ctrl Pts',(-207.123961567999,62.0513964889848,7.94222582815451));
#14827=CARTESIAN_POINT('Ctrl Pts',(-203.671656835844,61.6175482493094,8.10113414695882));
#14828=CARTESIAN_POINT('Ctrl Pts',(-202.03418792352,63.5720699870132,8.21758438851483));
#14829=CARTESIAN_POINT('Ctrl Pts',(-201.923445027477,64.7945230333643,8.28106519046941));
#14830=CARTESIAN_POINT('Ctrl Pts',(-201.925313606426,64.9972772118362,8.29157655282255));
#14831=CARTESIAN_POINT('Ctrl Pts',(-201.929918596978,64.9979181762371,7.20842344717746));
#14832=CARTESIAN_POINT('Ctrl Pts',(-201.93398631635,65.6521116579694,7.24220985311768));
#14833=CARTESIAN_POINT('Ctrl Pts',(-202.459399722692,67.3378982854403,7.32896569865932));
#14834=CARTESIAN_POINT('Ctrl Pts',(-205.234272792136,68.6263744085096,7.46869098380242));
#14835=CARTESIAN_POINT('Ctrl Pts',(-208.175332472178,66.7671272684671,7.62759930260672));
#14836=CARTESIAN_POINT('Ctrl Pts',(-208.205282831762,63.2877975995101,7.78650762141103));
#14837=CARTESIAN_POINT('Ctrl Pts',(-205.29666571597,61.3781959543899,7.94541594021533));
#14838=CARTESIAN_POINT('Ctrl Pts',(-202.481742432778,62.6268207185444,8.08605454880415));
#14839=CARTESIAN_POINT('Ctrl Pts',(-201.934125714812,64.3306029100366,8.17372371779152));
#14840=CARTESIAN_POINT('Ctrl Pts',(-201.92953466944,65.0022696572995,8.20842344717746));
#14841=CARTESIAN_POINT('Origin',(-205.,65.,-2.20842344717744));
#14842=CARTESIAN_POINT('',(-201.921960580212,64.9987333336508,6.20842344717746));
#14843=CARTESIAN_POINT('',(-201.930412916854,65.0017670725165,6.29157655282255));
#14844=CARTESIAN_POINT('',(-201.9265,65.0000000000003,-2.20842344717744));
#14845=CARTESIAN_POINT('Ctrl Pts',(-201.930412916854,65.0017670725165,6.29157655282255));
#14846=CARTESIAN_POINT('Ctrl Pts',(-201.928336333622,65.3992879077885,6.31209858191885));
#14847=CARTESIAN_POINT('Ctrl Pts',(-202.184898002603,66.8202733387973,6.38559005061658));
#14848=CARTESIAN_POINT('Ctrl Pts',(-204.32971180134,68.5715807618264,6.51205095891576));
#14849=CARTESIAN_POINT('Ctrl Pts',(-207.639355851724,67.4978542982895,6.67095927772006));
#14850=CARTESIAN_POINT('Ctrl Pts',(-208.529267956781,64.1341229320817,6.82986759652437));
#14851=CARTESIAN_POINT('Ctrl Pts',(-206.18358664496,61.5642179840126,6.98877591532868));
#14852=CARTESIAN_POINT('Ctrl Pts',(-202.860869889385,62.1259311837648,7.1426789007614));
#14853=CARTESIAN_POINT('Ctrl Pts',(-201.92849511178,64.0787222254988,7.2436124465927));
#14854=CARTESIAN_POINT('Ctrl Pts',(-201.922453672097,65.0016690942922,7.29157655282255));
#14855=CARTESIAN_POINT('Ctrl Pts',(-201.921960580212,64.9987333336508,6.20842344717746));
#14856=CARTESIAN_POINT('Ctrl Pts',(-201.926898162024,65.9470439039035,6.2577265488424));
#14857=CARTESIAN_POINT('Ctrl Pts',(-202.905060880587,67.9229822365129,6.35999909010877));
#14858=CARTESIAN_POINT('Ctrl Pts',(-206.269917767397,68.4048177566322,6.51524107097658));
#14859=CARTESIAN_POINT('Ctrl Pts',(-208.549995805274,65.7765338848791,6.67414938978088));
#14860=CARTESIAN_POINT('Ctrl Pts',(-207.575477366445,62.4363324266277,6.83305770858519));
#14861=CARTESIAN_POINT('Ctrl Pts',(-204.239790063637,61.4464727460615,6.99196602738949));
#14862=CARTESIAN_POINT('Ctrl Pts',(-202.162091334594,63.2322401369024,7.11708794025358));
#14863=CARTESIAN_POINT('Ctrl Pts',(-201.927609052785,64.6264843041873,7.18924041351624));
#14864=CARTESIAN_POINT('Ctrl Pts',(-201.929918596978,64.9979181762371,7.20842344717746));
#14865=CARTESIAN_POINT('Origin',(-205.,65.,-2.20842344717744));
#14866=CARTESIAN_POINT('',(-201.926100634672,65.0028070195242,5.20842344717746));
#14867=CARTESIAN_POINT('',(-201.928910969323,64.9974995382691,5.29157655282255));
#14868=CARTESIAN_POINT('',(-201.9265,65.0000000000003,-2.20842344717744));
#14869=CARTESIAN_POINT('Ctrl Pts',(-201.928910969323,64.9974995382691,5.29157655282255));
#14870=CARTESIAN_POINT('Ctrl Pts',(-201.934235720436,65.6947278648159,5.32761527764357));
#14871=CARTESIAN_POINT('Ctrl Pts',(-202.515344024246,67.4247683985249,5.41662344206603));
#14872=CARTESIAN_POINT('Ctrl Pts',(-205.387973940047,68.613163659365,5.55860104608992));
#14873=CARTESIAN_POINT('Ctrl Pts',(-208.247472484712,66.6307660373427,5.71750936489423));
#14874=CARTESIAN_POINT('Ctrl Pts',(-208.129724551721,63.1533003390197,5.87641768369853));
#14875=CARTESIAN_POINT('Ctrl Pts',(-205.142680129997,61.368868249703,6.03532600250284));
#14876=CARTESIAN_POINT('Ctrl Pts',(-202.427479508272,62.7139482003332,6.17371229221085));
#14877=CARTESIAN_POINT('Ctrl Pts',(-201.933696205667,64.3732462929244,6.25912914231742));
#14878=CARTESIAN_POINT('Ctrl Pts',(-201.930412916854,65.0017670725165,6.29157655282255));
#14879=CARTESIAN_POINT('Ctrl Pts',(-201.926100634672,65.0028070195242,5.20842344717746));
#14880=CARTESIAN_POINT('Ctrl Pts',(-201.923984761182,65.2315394103251,5.22027380496568));
#14881=CARTESIAN_POINT('Ctrl Pts',(-202.051779433128,66.4803311623585,5.28509360235534));
#14882=CARTESIAN_POINT('Ctrl Pts',(-203.757442149492,68.4148975211522,5.40288283934643));
#14883=CARTESIAN_POINT('Ctrl Pts',(-207.197698349872,67.894062379217,5.56179115815073));
#14884=CARTESIAN_POINT('Ctrl Pts',(-208.623129266309,64.7199831943528,5.72069947695504));
#14885=CARTESIAN_POINT('Ctrl Pts',(-206.726915766361,61.8026202872159,5.87960779575935));
#14886=CARTESIAN_POINT('Ctrl Pts',(-203.247485193193,61.8165793643074,6.03851611456365));
#14887=CARTESIAN_POINT('Ctrl Pts',(-201.955780778247,63.8392267441314,6.14812133170303));
#14888=CARTESIAN_POINT('Ctrl Pts',(-201.921593405675,64.9282138956866,6.20475710924096));
#14889=CARTESIAN_POINT('Ctrl Pts',(-201.921960580212,64.9987333336508,6.20842344717746));
#14890=CARTESIAN_POINT('Origin',(-205.,65.,-2.20842344717744));
#14891=CARTESIAN_POINT('',(-201.931423654547,64.9997186192924,4.20842344717746));
#14892=CARTESIAN_POINT('',(-201.921426709108,64.9994934768783,4.29157655282255));
#14893=CARTESIAN_POINT('',(-201.9265,65.0000000000003,-2.20842344717744));
#14894=CARTESIAN_POINT('Ctrl Pts',(-201.921426709108,64.9994934768783,4.29157655282255));
#14895=CARTESIAN_POINT('Ctrl Pts',(-201.923689577646,65.9906673436395,4.34313197336829));
#14896=CARTESIAN_POINT('Ctrl Pts',(-202.981935595717,68.0043503849495,4.44765683351547));
#14897=CARTESIAN_POINT('Ctrl Pts',(-206.413282312349,68.3478513278105,4.60515113326408));
#14898=CARTESIAN_POINT('Ctrl Pts',(-208.579754999423,65.6251636198798,4.76405945206838));
#14899=CARTESIAN_POINT('Ctrl Pts',(-207.464348313206,62.3293328925706,4.92296777087269));
#14900=CARTESIAN_POINT('Ctrl Pts',(-204.089654636955,61.4819399198572,5.081876089677));
#14901=CARTESIAN_POINT('Ctrl Pts',(-202.125623034005,63.3205768432535,5.20474568366028));
#14902=CARTESIAN_POINT('Ctrl Pts',(-201.926409442345,64.6699470515422,5.27464583804213));
#14903=CARTESIAN_POINT('Ctrl Pts',(-201.928910969323,64.9974995382691,5.29157655282255));
#14904=CARTESIAN_POINT('Ctrl Pts',(-201.931423654547,64.9997186192924,4.20842344717746));
#14905=CARTESIAN_POINT('Ctrl Pts',(-201.931856309214,65.5302670894482,4.2357905006904));
#14906=CARTESIAN_POINT('Ctrl Pts',(-202.315183242628,67.0882876073577,4.31612699380478));
#14907=CARTESIAN_POINT('Ctrl Pts',(-204.794831478631,68.6281373967567,4.44943292652058));
#14908=CARTESIAN_POINT('Ctrl Pts',(-207.938810626636,67.1374908637484,4.60834124532489));
#14909=CARTESIAN_POINT('Ctrl Pts',(-208.388521038603,63.6872165971666,4.7672495641292));
#14910=CARTESIAN_POINT('Ctrl Pts',(-205.731673235186,61.4404874815853,4.92615788293351));
#14911=CARTESIAN_POINT('Ctrl Pts',(-202.652189346928,62.3812687692724,5.07321584394959));
#14912=CARTESIAN_POINT('Ctrl Pts',(-201.933442419344,64.209137658754,5.16730436536424));
#14913=CARTESIAN_POINT('Ctrl Pts',(-201.926100634672,65.0028070195242,5.20842344717746));
#14914=CARTESIAN_POINT('Origin',(-205.,65.,-2.20842344717744));
#14915=CARTESIAN_POINT('',(-201.925065626664,64.9973187943263,3.20842344717745));
#14916=CARTESIAN_POINT('',(-201.927406901239,65.0027899110459,3.29157655282255));
#14917=CARTESIAN_POINT('',(-201.9265,65.0000000000003,-2.20842344717744));
#14918=CARTESIAN_POINT('Ctrl Pts',(-201.927406901239,65.0027899110459,3.29157655282255));
#14919=CARTESIAN_POINT('Ctrl Pts',(-201.924995843745,65.2752913043072,3.30567922949157));
#14920=CARTESIAN_POINT('Ctrl Pts',(-202.083109248922,66.5685525880974,3.37275134576203));
#14921=CARTESIAN_POINT('Ctrl Pts',(-203.90349843384,68.4645576515751,3.49279290163393));
#14922=CARTESIAN_POINT('Ctrl Pts',(-207.318549180862,67.7981788906371,3.65170122043823));
#14923=CARTESIAN_POINT('Ctrl Pts',(-208.607979952898,64.5664609969902,3.81060953924254));
#14924=CARTESIAN_POINT('Ctrl Pts',(-206.589655029722,61.7322068159406,3.96951785804685));
#14925=CARTESIAN_POINT('Ctrl Pts',(-203.113952142563,61.893828902484,4.12842617685116));
#14926=CARTESIAN_POINT('Ctrl Pts',(-201.934013495981,63.9268235650214,4.23577907510972));
#14927=CARTESIAN_POINT('Ctrl Pts',(-201.921364645038,64.9723083871191,4.29016253376685));
#14928=CARTESIAN_POINT('Ctrl Pts',(-201.921426709108,64.9994934768783,4.29157655282255));
#14929=CARTESIAN_POINT('Ctrl Pts',(-201.925065626664,64.9973187943263,3.20842344717745));
#14930=CARTESIAN_POINT('Ctrl Pts',(-201.932640043333,65.8243336692917,3.25130719641511));
#14931=CARTESIAN_POINT('Ctrl Pts',(-202.703271173878,67.6853099211375,3.34716038525421));
#14932=CARTESIAN_POINT('Ctrl Pts',(-205.849647429869,68.5332102033146,3.49598301369475));
#14933=CARTESIAN_POINT('Ctrl Pts',(-208.430305934935,66.1993649512308,3.65489133249905));
#14934=CARTESIAN_POINT('Ctrl Pts',(-207.866098297326,62.7659553182491,3.81379965130336));
#14935=CARTESIAN_POINT('Ctrl Pts',(-204.674283775171,61.380692879392,3.97270797010767));
#14936=CARTESIAN_POINT('Ctrl Pts',(-202.279346917231,62.9806921969728,4.10424923539903));
#14937=CARTESIAN_POINT('Ctrl Pts',(-201.931018898082,64.5033806863407,4.18282106108896));
#14938=CARTESIAN_POINT('Ctrl Pts',(-201.931423654547,64.9997186192924,4.20842344717746));
#14939=CARTESIAN_POINT('Origin',(-205.,65.,-2.20842344717744));
#14940=CARTESIAN_POINT('',(-201.922632956914,65.0017870279701,2.20842344717745));
#14941=CARTESIAN_POINT('',(-201.931155193317,64.9990189320844,2.29157655282255));
#14942=CARTESIAN_POINT('',(-201.9265,65.0000000000003,-2.20842344717744));
#14943=CARTESIAN_POINT('Ctrl Pts',(-201.931155193316,64.9990189320844,2.29157655282255));
#14944=CARTESIAN_POINT('Ctrl Pts',(-201.932795838262,65.5731064476581,2.32119592521629));
#14945=CARTESIAN_POINT('Ctrl Pts',(-202.363272241673,67.1761406694018,2.40378473721147));
#14946=CARTESIAN_POINT('Ctrl Pts',(-204.949003425354,68.6335760097311,2.53934298880809));
#14947=CARTESIAN_POINT('Ctrl Pts',(-208.026882902896,67.010834485032,2.6982513076124));
#14948=CARTESIAN_POINT('Ctrl Pts',(-208.329749972245,63.5445823456684,2.8571596264167));
#14949=CARTESIAN_POINT('Ctrl Pts',(-205.579939479888,61.4126408611514,3.01606794522101));
#14950=CARTESIAN_POINT('Ctrl Pts',(-202.589670400847,62.4668776130536,3.16087358735629));
#14951=CARTESIAN_POINT('Ctrl Pts',(-201.93405173911,64.2517802056398,3.25270978989014));
#14952=CARTESIAN_POINT('Ctrl Pts',(-201.927406901239,65.0027899110459,3.29157655282255));
#14953=CARTESIAN_POINT('Ctrl Pts',(-201.922632956914,65.0017870279701,2.20842344717745));
#14954=CARTESIAN_POINT('Ctrl Pts',(-201.921910543138,65.106308912415,2.2138544525384));
#14955=CARTESIAN_POINT('Ctrl Pts',(-201.974200288337,66.229517676892,2.27225489750078));
#14956=CARTESIAN_POINT('Ctrl Pts',(-203.354325972851,68.2399430433535,2.3836247820646));
#14957=CARTESIAN_POINT('Ctrl Pts',(-206.83229589241,68.1381789310981,2.54253310086891));
#14958=CARTESIAN_POINT('Ctrl Pts',(-208.630437627999,65.1593672402151,2.70144141967321));
#14959=CARTESIAN_POINT('Ctrl Pts',(-207.100234620393,62.0344495464248,2.86034973847752));
#14960=CARTESIAN_POINT('Ctrl Pts',(-203.644560036488,61.6283153137219,3.01925805728183));
#14961=CARTESIAN_POINT('Ctrl Pts',(-202.028754311406,63.5887202320378,3.13528262684847));
#14962=CARTESIAN_POINT('Ctrl Pts',(-201.923284224092,64.8028158391646,3.19833775681368));
#14963=CARTESIAN_POINT('Ctrl Pts',(-201.925065626664,64.9973187943263,3.20842344717745));
#14964=CARTESIAN_POINT('Origin',(-205.,65.,-2.20842344717744));
#14965=CARTESIAN_POINT('',(-201.930557054308,65.0016530359719,1.20842344717746));
#14966=CARTESIAN_POINT('',(-201.923803965215,64.9976529174956,1.29157655282255));
#14967=CARTESIAN_POINT('',(-201.9265,65.0000000000003,-2.20842344717744));
#14968=CARTESIAN_POINT('Ctrl Pts',(-201.923803965215,64.9976529174956,1.29157655282255));
#14969=CARTESIAN_POINT('Ctrl Pts',(-201.931157916033,65.8671791615852,1.33671262094101));
#14970=CARTESIAN_POINT('Ctrl Pts',(-202.771191556777,67.7695720873782,1.43481812866091));
#14971=CARTESIAN_POINT('Ctrl Pts',(-205.998840235539,68.4939639431765,1.58589307598225));
#14972=CARTESIAN_POINT('Ctrl Pts',(-208.478118835308,66.0526943186335,1.74480139478656));
#14973=CARTESIAN_POINT('Ctrl Pts',(-207.768697443447,62.6463237610936,1.90370971359086));
#14974=CARTESIAN_POINT('Ctrl Pts',(-204.520964946279,61.3977785102674,2.06261803239517));
#14975=CARTESIAN_POINT('Ctrl Pts',(-202.235901714706,63.0688711165209,2.19190697880573));
#14976=CARTESIAN_POINT('Ctrl Pts',(-201.929861811092,64.5464441140382,2.26822648561486));
#14977=CARTESIAN_POINT('Ctrl Pts',(-201.931155193316,64.9990189320844,2.29157655282255));
#14978=CARTESIAN_POINT('Ctrl Pts',(-201.930557054308,65.0016530359719,1.20842344717746));
#14979=CARTESIAN_POINT('Ctrl Pts',(-201.928569592085,65.4074689546327,1.22937114826312));
#14980=CARTESIAN_POINT('Ctrl Pts',(-202.192314144726,66.836978287187,1.30328828895022));
#14981=CARTESIAN_POINT('Ctrl Pts',(-204.358399583502,68.5768348597731,1.43017486923876));
#14982=CARTESIAN_POINT('Ctrl Pts',(-207.659308320785,67.4766010095058,1.58908318804307));
#14983=CARTESIAN_POINT('Ctrl Pts',(-208.522208970686,64.1058310992964,1.74799150684737));
#14984=CARTESIAN_POINT('Ctrl Pts',(-206.155980002522,61.5548329839681,1.90689982565168));
#14985=CARTESIAN_POINT('Ctrl Pts',(-202.847056091155,62.1415595964765,2.06037713909504));
#14986=CARTESIAN_POINT('Ctrl Pts',(-201.928956357011,64.0868907242207,2.16088501293697));
#14987=CARTESIAN_POINT('Ctrl Pts',(-201.922632956914,65.0017870279701,2.20842344717745));
#14988=CARTESIAN_POINT('Origin',(-205.,65.,-2.20842344717744));
#14989=CARTESIAN_POINT('',(-201.929611540575,64.9968423971894,0.208423447177456));
#14990=CARTESIAN_POINT('',(-201.923731627295,65.0022750736125,0.291576552822547));
#14991=CARTESIAN_POINT('',(-201.9265,65.0000000000003,-2.20842344717744));
#14992=CARTESIAN_POINT('',(-204.206200717467,62.0307770462543,0.));
#14993=CARTESIAN_POINT('Ctrl Pts',(-204.206200717467,62.0307770462543,-5.55111512312578E-16));
#14994=CARTESIAN_POINT('Ctrl Pts',(-203.217993421758,62.2949667869871,0.052969439601435));
#14995=CARTESIAN_POINT('Ctrl Pts',(-202.119878197412,63.3375116748876,0.12244392199392));
#14996=CARTESIAN_POINT('Ctrl Pts',(-201.92719200432,64.6776063340067,0.191918404386406));
#14997=CARTESIAN_POINT('Ctrl Pts',(-201.929611540575,64.9968423971894,0.208423447177456));
#14998=CARTESIAN_POINT('',(-205.795567263823,62.0254195780229,4.05472878785602E-15));
#14999=CARTESIAN_POINT('Origin',(-205.,65.,0.));
#15000=CARTESIAN_POINT('Ctrl Pts',(-205.795568724168,62.0254151527766,-1.60732972070976E-16));
#15001=CARTESIAN_POINT('Ctrl Pts',(-204.831192689899,61.7689270501568,0.051906068914496));
#15002=CARTESIAN_POINT('Ctrl Pts',(-202.766529559188,62.2462762443893,0.149098253188679));
#15003=CARTESIAN_POINT('Ctrl Pts',(-201.931014203849,64.1300893064926,0.246290437462861));
#15004=CARTESIAN_POINT('Ctrl Pts',(-201.923731627295,65.0022750736125,0.291576552822547));
#15005=CARTESIAN_POINT('Origin',(-205.,-65.,9.));
#15006=CARTESIAN_POINT('',(-202.486496099891,-64.9993605807166,16.612583302492));
#15007=CARTESIAN_POINT('',(-202.484570781149,-65.0037022516384,16.887416697508));
#15008=CARTESIAN_POINT('',(-202.4825,-65.,9.));
#15009=CARTESIAN_POINT('',(-203.086534003335,-63.3640127966251,17.));
#15010=CARTESIAN_POINT('Ctrl Pts',(-202.484570781149,-65.0037022516384,
16.887416697508));
#15011=CARTESIAN_POINT('Ctrl Pts',(-202.489763089819,-64.4110264481633,
16.9249444650053));
#15012=CARTESIAN_POINT('Ctrl Pts',(-202.700778171916,-63.8151964396956,
16.9624722325027));
#15013=CARTESIAN_POINT('Ctrl Pts',(-203.086534003335,-63.3640127966251,
17.));
#15014=CARTESIAN_POINT('',(-202.4825,-65.,17.));
#15015=CARTESIAN_POINT('Origin',(-205.,-65.,17.));
#15016=CARTESIAN_POINT('',(-202.4825,-65.,18.));
#15017=CARTESIAN_POINT('',(-202.4825,-65.,9.));
#15018=CARTESIAN_POINT('Origin',(-205.,-65.,18.));
#15019=CARTESIAN_POINT('',(-206.917145184219,-63.36121664977,17.));
#15020=CARTESIAN_POINT('Origin',(-205.,-65.,17.));
#15021=CARTESIAN_POINT('Ctrl Pts',(-206.917148223239,-63.3612143401441,
17.));
#15022=CARTESIAN_POINT('Ctrl Pts',(-206.385177464426,-62.7406365841492,
16.9480939310855));
#15023=CARTESIAN_POINT('Ctrl Pts',(-205.522587726062,-62.4011240872398,
16.896187862171));
#15024=CARTESIAN_POINT('Ctrl Pts',(-204.710521467437,-62.4950490586621,
16.8442817932565));
#15025=CARTESIAN_POINT('Ctrl Pts',(-203.881818860243,-62.5908982185939,
16.7913123536551));
#15026=CARTESIAN_POINT('Ctrl Pts',(-203.105731029912,-63.1381259414902,
16.7383429140536));
#15027=CARTESIAN_POINT('Ctrl Pts',(-202.737501870931,-63.8863946460724,
16.6853734744522));
#15028=CARTESIAN_POINT('Ctrl Pts',(-202.568829368417,-64.2291495634286,
16.6611100837988));
#15029=CARTESIAN_POINT('Ctrl Pts',(-202.485734824973,-64.614087418431,16.6368466931454));
#15030=CARTESIAN_POINT('Ctrl Pts',(-202.486496099891,-64.9993605807166,
16.612583302492));
#15031=CARTESIAN_POINT('Origin',(-205.,-65.,9.));
#15032=CARTESIAN_POINT('',(-202.48281438265,-65.0023102366302,15.612583302492));
#15033=CARTESIAN_POINT('',(-202.478262929558,-64.9999671733494,15.887416697508));
#15034=CARTESIAN_POINT('',(-202.4825,-65.,9.));
#15035=CARTESIAN_POINT('Ctrl Pts',(-202.478262929558,-64.9999671733494,
15.887416697508));
#15036=CARTESIAN_POINT('Ctrl Pts',(-202.478152183127,-64.1647350270545,
15.9404611607301));
#15037=CARTESIAN_POINT('Ctrl Pts',(-202.934430543867,-63.3296386377248,
15.9935056239521));
#15038=CARTESIAN_POINT('Ctrl Pts',(-203.637206926075,-62.8782359116843,
16.0465500871742));
#15039=CARTESIAN_POINT('Ctrl Pts',(-204.338989334068,-62.4274716286557,
16.0995195267756));
#15040=CARTESIAN_POINT('Ctrl Pts',(-205.286572151919,-62.3593164180464,
16.152488966377));
#15041=CARTESIAN_POINT('Ctrl Pts',(-206.045557144883,-62.7051788961069,
16.2054584059785));
#15042=CARTESIAN_POINT('Ctrl Pts',(-206.804542137847,-63.0510413741674,
16.2584278455799));
#15043=CARTESIAN_POINT('Ctrl Pts',(-207.374929305926,-63.8109215408977,
16.3113972851813));
#15044=CARTESIAN_POINT('Ctrl Pts',(-207.495321385823,-64.636151503456,16.3643667247828));
#15045=CARTESIAN_POINT('Ctrl Pts',(-207.61571346572,-65.4613814660144,16.4173361643842));
#15046=CARTESIAN_POINT('Ctrl Pts',(-207.286110457436,-66.3519612244009,
16.4703056039856));
#15047=CARTESIAN_POINT('Ctrl Pts',(-206.657467982026,-66.9003622583766,
16.5232750435871));
#15048=CARTESIAN_POINT('Ctrl Pts',(-206.028825506615,-67.4487632923523,
16.5762444831885));
#15049=CARTESIAN_POINT('Ctrl Pts',(-205.101143564078,-67.6549856019172,
16.6292139227899));
#15050=CARTESIAN_POINT('Ctrl Pts',(-204.299948783103,-67.4230386209089,
16.6821833623914));
#15051=CARTESIAN_POINT('Ctrl Pts',(-203.498754002127,-67.1910916399006,
16.7351528019928));
#15052=CARTESIAN_POINT('Ctrl Pts',(-202.824046382713,-66.520975368319,16.7881222415943));
#15053=CARTESIAN_POINT('Ctrl Pts',(-202.584870374653,-65.7234140671963,
16.8410916811957));
#15054=CARTESIAN_POINT('Ctrl Pts',(-202.515145689638,-65.4909086794192,
16.8565333532998));
#15055=CARTESIAN_POINT('Ctrl Pts',(-202.482434285074,-65.2475724851116,
16.8719750254039));
#15056=CARTESIAN_POINT('Ctrl Pts',(-202.484570781149,-65.0037022516384,
16.887416697508));
#15057=CARTESIAN_POINT('Ctrl Pts',(-202.486496099891,-64.9993605807166,
16.612583302492));
#15058=CARTESIAN_POINT('Ctrl Pts',(-202.487396765235,-65.4551777586583,
16.583877253544));
#15059=CARTESIAN_POINT('Ctrl Pts',(-202.605672824408,-65.9114642758204,
16.5551712045959));
#15060=CARTESIAN_POINT('Ctrl Pts',(-202.838472376554,-66.2989195852673,
16.5264651556479));
#15061=CARTESIAN_POINT('Ctrl Pts',(-203.268042528788,-67.0138661336119,
16.4734957160465));
#15062=CARTESIAN_POINT('Ctrl Pts',(-204.087553320887,-67.4944495440329,
16.420526276445));
#15063=CARTESIAN_POINT('Ctrl Pts',(-204.92122517779,-67.5204925072279,16.3675568368436));
#15064=CARTESIAN_POINT('Ctrl Pts',(-205.754897034692,-67.5465354704228,
16.3145873972421));
#15065=CARTESIAN_POINT('Ctrl Pts',(-206.602729956398,-67.1180379863916,
16.2616179576407));
#15066=CARTESIAN_POINT('Ctrl Pts',(-207.076140556712,-66.4313628943424,
16.2086485180393));
#15067=CARTESIAN_POINT('Ctrl Pts',(-207.549551157025,-65.7446878022932,
16.1556790784378));
#15068=CARTESIAN_POINT('Ctrl Pts',(-207.648539435946,-64.799835102226,16.1027096388364));
#15069=CARTESIAN_POINT('Ctrl Pts',(-207.327701310022,-64.0299481709965,
16.049740199235));
#15070=CARTESIAN_POINT('Ctrl Pts',(-207.006863184097,-63.2600612397671,
15.9967707596335));
#15071=CARTESIAN_POINT('Ctrl Pts',(-206.266198653327,-62.6651400773755,
15.9438013200321));
#15072=CARTESIAN_POINT('Ctrl Pts',(-205.445237999217,-62.5178795321244,
15.8908318804307));
#15073=CARTESIAN_POINT('Ctrl Pts',(-204.624277345108,-62.3706189868733,
15.8378624408292));
#15074=CARTESIAN_POINT('Ctrl Pts',(-203.72302056766,-62.6710190587628,15.7848930012278));
#15075=CARTESIAN_POINT('Ctrl Pts',(-203.154592033966,-63.2813846823738,
15.7319235616264));
#15076=CARTESIAN_POINT('Ctrl Pts',(-202.727701805557,-63.7397696947918,
15.6921434752482));
#15077=CARTESIAN_POINT('Ctrl Pts',(-202.48852739089,-64.3729759156404,15.6523633888701));
#15078=CARTESIAN_POINT('Ctrl Pts',(-202.48281438265,-65.0023102366302,15.612583302492));
#15079=CARTESIAN_POINT('Origin',(-205.,-65.,9.));
#15080=CARTESIAN_POINT('',(-202.478480635384,-64.9993246233377,14.612583302492));
#15081=CARTESIAN_POINT('',(-202.483913362404,-64.9978104805478,14.887416697508));
#15082=CARTESIAN_POINT('',(-202.4825,-65.,9.));
#15083=CARTESIAN_POINT('Ctrl Pts',(-202.483913362404,-64.9978104805478,
14.887416697508));
#15084=CARTESIAN_POINT('Ctrl Pts',(-202.481864049093,-64.7508707218699,
14.9030084168533));
#15085=CARTESIAN_POINT('Ctrl Pts',(-202.51526717488,-64.5044733838642,14.9186001361987));
#15086=CARTESIAN_POINT('Ctrl Pts',(-202.586387196479,-64.2694915479097,
14.934191855544));
#15087=CARTESIAN_POINT('Ctrl Pts',(-202.828001838529,-63.4711924064649,
14.9871612951454));
#15088=CARTESIAN_POINT('Ctrl Pts',(-203.504926517813,-62.8046454284989,
15.0401307347469));
#15089=CARTESIAN_POINT('Ctrl Pts',(-204.306862945724,-62.5753909604694,
15.0931001743483));
#15090=CARTESIAN_POINT('Ctrl Pts',(-205.108799373635,-62.34613649244,15.1460696139497));
#15091=CARTESIAN_POINT('Ctrl Pts',(-206.035747550172,-62.5541745343471,
15.1990390535512));
#15092=CARTESIAN_POINT('Ctrl Pts',(-206.66279919664,-63.1041437994002,15.2520084931526));
#15093=CARTESIAN_POINT('Ctrl Pts',(-207.289850843108,-63.6541130644534,
15.3049779327541));
#15094=CARTESIAN_POINT('Ctrl Pts',(-207.617005959508,-64.5460135526525,
15.3579473723555));
#15095=CARTESIAN_POINT('Ctrl Pts',(-207.494299322538,-65.3709985580089,
15.4109168119569));
#15096=CARTESIAN_POINT('Ctrl Pts',(-207.371592685568,-66.1959835633652,
15.4638862515584));
#15097=CARTESIAN_POINT('Ctrl Pts',(-206.799024295229,-66.9540530858788,
15.5168556911598));
#15098=CARTESIAN_POINT('Ctrl Pts',(-206.039054544245,-67.2977215702459,
15.5698251307612));
#15099=CARTESIAN_POINT('Ctrl Pts',(-205.27908479326,-67.6413900546129,15.6227945703627));
#15100=CARTESIAN_POINT('Ctrl Pts',(-204.33171368163,-67.5706575008334,15.6757640099641));
#15101=CARTESIAN_POINT('Ctrl Pts',(-203.631214451117,-67.1179282170362,
15.7287334495655));
#15102=CARTESIAN_POINT('Ctrl Pts',(-202.931707377382,-66.6658401593929,
15.7816278655464));
#15103=CARTESIAN_POINT('Ctrl Pts',(-202.47837336272,-65.832836692676,15.8345222815272));
#15104=CARTESIAN_POINT('Ctrl Pts',(-202.478262929558,-64.9999671733494,
15.887416697508));
#15105=CARTESIAN_POINT('Ctrl Pts',(-202.48281438265,-65.0023102366302,15.612583302492));
#15106=CARTESIAN_POINT('Ctrl Pts',(-202.480920196627,-65.2109702323926,
15.5993939492687));
#15107=CARTESIAN_POINT('Ctrl Pts',(-202.504690383233,-65.4192045908632,
15.5862045960454));
#15108=CARTESIAN_POINT('Ctrl Pts',(-202.555792276411,-65.6205003111822,
15.5730152428221));
#15109=CARTESIAN_POINT('Ctrl Pts',(-202.761021342488,-66.4289191410472,
15.5200458032206));
#15110=CARTESIAN_POINT('Ctrl Pts',(-203.407079764582,-67.1254256254448,
15.4670763636192));
#15111=CARTESIAN_POINT('Ctrl Pts',(-204.197816390868,-67.3907466530304,
15.4141069240177));
#15112=CARTESIAN_POINT('Ctrl Pts',(-204.988553017154,-67.6560676806159,
15.3611374844163));
#15113=CARTESIAN_POINT('Ctrl Pts',(-205.923967847632,-67.4902032513894,
15.3081680448149));
#15114=CARTESIAN_POINT('Ctrl Pts',(-206.575272719714,-66.9691839307848,
15.2551986052134));
#15115=CARTESIAN_POINT('Ctrl Pts',(-207.226577591796,-66.4481646101802,
15.202229165612));
#15116=CARTESIAN_POINT('Ctrl Pts',(-207.593772505481,-65.5719903981975,
15.1492597260106));
#15117=CARTESIAN_POINT('Ctrl Pts',(-207.508536991204,-64.7422950273395,
15.0962902864091));
#15118=CARTESIAN_POINT('Ctrl Pts',(-207.423301476928,-63.9125996564815,
15.0433208468077));
#15119=CARTESIAN_POINT('Ctrl Pts',(-206.885635534689,-63.1293831267483,
14.9903514072063));
#15120=CARTESIAN_POINT('Ctrl Pts',(-206.14200240898,-62.7516673386529,14.9373819676048));
#15121=CARTESIAN_POINT('Ctrl Pts',(-205.398369283272,-62.3739515505575,
14.8844125280034));
#15122=CARTESIAN_POINT('Ctrl Pts',(-204.448768974094,-62.4017365040998,
14.831443088402));
#15123=CARTESIAN_POINT('Ctrl Pts',(-203.728492868385,-62.822285819182,14.7784736488005));
#15124=CARTESIAN_POINT('Ctrl Pts',(-203.008216762676,-63.2428351342642,
14.7255042091991));
#15125=CARTESIAN_POINT('Ctrl Pts',(-202.517264860435,-64.0561488108863,
14.6725347695977));
#15126=CARTESIAN_POINT('Ctrl Pts',(-202.480686812783,-64.889408362383,14.6195653299962));
#15127=CARTESIAN_POINT('Ctrl Pts',(-202.479079666369,-64.9260196685153,
14.6172379874948));
#15128=CARTESIAN_POINT('Ctrl Pts',(-202.478349688759,-64.9626694801625,
14.6149106449934));
#15129=CARTESIAN_POINT('Ctrl Pts',(-202.478480635384,-64.9993246233377,
14.612583302492));
#15130=CARTESIAN_POINT('Origin',(-205.,-65.,9.));
#15131=CARTESIAN_POINT('',(-202.484829278355,-64.9980759284861,13.612583302492));
#15132=CARTESIAN_POINT('',(-202.486036851904,-65.0011568554962,13.887416697508));
#15133=CARTESIAN_POINT('',(-202.4825,-65.,9.));
#15134=CARTESIAN_POINT('Ctrl Pts',(-202.486036851904,-65.0011568554962,
13.887416697508));
#15135=CARTESIAN_POINT('Ctrl Pts',(-202.488081620308,-64.5074181159925,
13.9185251125781));
#15136=CARTESIAN_POINT('Ctrl Pts',(-202.628468371682,-64.0126062150085,
13.9496335276481));
#15137=CARTESIAN_POINT('Ctrl Pts',(-202.899518826464,-63.6045975021718,
13.9807419427182));
#15138=CARTESIAN_POINT('Ctrl Pts',(-203.361046379736,-62.9098660983765,
14.0337113823196));
#15139=CARTESIAN_POINT('Ctrl Pts',(-204.201408805511,-62.4668042390463,
14.086680821921));
#15140=CARTESIAN_POINT('Ctrl Pts',(-205.035388666738,-62.4785089905249,
14.1396502615225));
#15141=CARTESIAN_POINT('Ctrl Pts',(-205.869368527965,-62.4902137420035,
14.1926197011239));
#15142=CARTESIAN_POINT('Ctrl Pts',(-206.696965824644,-62.956685104291,14.2455891407254));
#15143=CARTESIAN_POINT('Ctrl Pts',(-207.138814575472,-63.664095240497,14.2985585803268));
#15144=CARTESIAN_POINT('Ctrl Pts',(-207.580663326299,-64.3715053767029,
14.3515280199282));
#15145=CARTESIAN_POINT('Ctrl Pts',(-207.636763531275,-65.3198542868274,
14.4044974595297));
#15146=CARTESIAN_POINT('Ctrl Pts',(-207.281399181164,-66.0744240710213,
14.4574668991311));
#15147=CARTESIAN_POINT('Ctrl Pts',(-206.926034831053,-66.8289938552152,
14.5104363387325));
#15148=CARTESIAN_POINT('Ctrl Pts',(-206.159205925855,-67.3897845134786,
14.563405778334));
#15149=CARTESIAN_POINT('Ctrl Pts',(-205.33242252728,-67.4997328638535,14.6163752179354));
#15150=CARTESIAN_POINT('Ctrl Pts',(-204.505639128704,-67.6096812142285,
14.6693446575368));
#15151=CARTESIAN_POINT('Ctrl Pts',(-203.618901236752,-67.268787256715,14.7223140971383));
#15152=CARTESIAN_POINT('Ctrl Pts',(-203.078684593183,-66.6333146254965,
14.7752835367397));
#15153=CARTESIAN_POINT('Ctrl Pts',(-202.697482399372,-66.1848953403611,
14.8126612569958));
#15154=CARTESIAN_POINT('Ctrl Pts',(-202.488826140652,-65.5897942775585,
14.8500389772519));
#15155=CARTESIAN_POINT('Ctrl Pts',(-202.483913362404,-64.9978104805478,
14.887416697508));
#15156=CARTESIAN_POINT('Ctrl Pts',(-202.478480635384,-64.9993246233377,
14.612583302492));
#15157=CARTESIAN_POINT('Ctrl Pts',(-202.481329984672,-65.7969267462619,
14.561941205392));
#15158=CARTESIAN_POINT('Ctrl Pts',(-202.891810794862,-66.597053247633,14.5112991082919));
#15159=CARTESIAN_POINT('Ctrl Pts',(-203.542558949731,-67.0579200627044,
14.4606570111919));
#15160=CARTESIAN_POINT('Ctrl Pts',(-204.223213327393,-67.5399667851577,
14.4076875715905));
#15161=CARTESIAN_POINT('Ctrl Pts',(-205.166726275778,-67.6508548036931,
14.354718131989));
#15162=CARTESIAN_POINT('Ctrl Pts',(-205.940596742163,-67.3397536602911,
14.3017486923876));
#15163=CARTESIAN_POINT('Ctrl Pts',(-206.714467208547,-67.0286525168891,
14.2487792527862));
#15164=CARTESIAN_POINT('Ctrl Pts',(-207.318695192931,-66.2955622115496,
14.1958098131847));
#15165=CARTESIAN_POINT('Ctrl Pts',(-207.476305959037,-65.4765272483028,
14.1428403735833));
#15166=CARTESIAN_POINT('Ctrl Pts',(-207.633916725142,-64.657492285056,14.0898709339819));
#15167=CARTESIAN_POINT('Ctrl Pts',(-207.34491027297,-63.7525126639018,14.0369014943804));
#15168=CARTESIAN_POINT('Ctrl Pts',(-206.741765547493,-63.1764259834307,
13.983932054779));
#15169=CARTESIAN_POINT('Ctrl Pts',(-206.138620822016,-62.6003393029595,
13.9309626151776));
#15170=CARTESIAN_POINT('Ctrl Pts',(-205.221337823236,-62.3531455631714,
13.8779931755761));
#15171=CARTESIAN_POINT('Ctrl Pts',(-204.410393950494,-62.5481569941157,
13.8250237359747));
#15172=CARTESIAN_POINT('Ctrl Pts',(-203.599450077753,-62.74316842506,13.7720542963732));
#15173=CARTESIAN_POINT('Ctrl Pts',(-202.894845331051,-63.3803850267366,
13.7190848567718));
#15174=CARTESIAN_POINT('Ctrl Pts',(-202.619566589227,-64.167710269399,13.6661154171704));
#15175=CARTESIAN_POINT('Ctrl Pts',(-202.526832279993,-64.4329398401132,
13.6482713789442));
#15176=CARTESIAN_POINT('Ctrl Pts',(-202.482819703866,-64.7152043750739,
13.6304273407181));
#15177=CARTESIAN_POINT('Ctrl Pts',(-202.484829278355,-64.9980759284861,
13.612583302492));
#15178=CARTESIAN_POINT('Origin',(-205.,-65.,9.));
#15179=CARTESIAN_POINT('',(-202.485436300316,-65.0016271999185,12.612583302492));
#15180=CARTESIAN_POINT('',(-202.47967327723,-65.0016558771702,12.887416697508));
#15181=CARTESIAN_POINT('',(-202.4825,-65.,9.));
#15182=CARTESIAN_POINT('Ctrl Pts',(-202.47967327723,-65.0016558771702,12.887416697508));
#15183=CARTESIAN_POINT('Ctrl Pts',(-202.485262109409,-64.2664021257915,
12.9340418083028));
#15184=CARTESIAN_POINT('Ctrl Pts',(-202.825745335394,-63.5266425796602,
12.9806669190976));
#15185=CARTESIAN_POINT('Ctrl Pts',(-203.391061346414,-63.0582261468577,
13.0272920298923));
#15186=CARTESIAN_POINT('Ctrl Pts',(-204.033300513057,-62.5260717879144,
13.0802614694938));
#15187=CARTESIAN_POINT('Ctrl Pts',(-204.965721795584,-62.3441284479905,
13.1332309090952));
#15188=CARTESIAN_POINT('Ctrl Pts',(-205.760908488858,-62.5957979371522,
13.1862003486966));
#15189=CARTESIAN_POINT('Ctrl Pts',(-206.556095182133,-62.8474674263139,
13.2391697882981));
#15190=CARTESIAN_POINT('Ctrl Pts',(-207.214047286156,-63.5327497445611,
13.2921392278995));
#15191=CARTESIAN_POINT('Ctrl Pts',(-207.433163233268,-64.3375153072165,
13.3451086675009));
#15192=CARTESIAN_POINT('Ctrl Pts',(-207.652279180381,-65.1422808698718,
13.3980781071024));
#15193=CARTESIAN_POINT('Ctrl Pts',(-207.432558970583,-66.0665296769353,
13.4510475467038));
#15194=CARTESIAN_POINT('Ctrl Pts',(-206.87472112031,-66.6865912395403,13.5040169863053));
#15195=CARTESIAN_POINT('Ctrl Pts',(-206.316883270037,-67.3066528021453,
13.5569864259067));
#15196=CARTESIAN_POINT('Ctrl Pts',(-205.420927779289,-67.6225271202918,
13.6099558655081));
#15197=CARTESIAN_POINT('Ctrl Pts',(-204.597555637766,-67.4894191733733,
13.6629253051096));
#15198=CARTESIAN_POINT('Ctrl Pts',(-203.774183496244,-67.3563112264548,
13.715894744711));
#15199=CARTESIAN_POINT('Ctrl Pts',(-203.023394703947,-66.7742210144714,
13.7688641843124));
#15200=CARTESIAN_POINT('Ctrl Pts',(-202.689346648184,-66.0099754343495,
13.8218336239139));
#15201=CARTESIAN_POINT('Ctrl Pts',(-202.551481630229,-65.6945635383438,
13.8436946484453));
#15202=CARTESIAN_POINT('Ctrl Pts',(-202.484599918132,-65.348125181336,13.8655556729766));
#15203=CARTESIAN_POINT('Ctrl Pts',(-202.486036851904,-65.0011568554962,
13.887416697508));
#15204=CARTESIAN_POINT('Ctrl Pts',(-202.484829278355,-64.9980759284861,
13.612583302492));
#15205=CARTESIAN_POINT('Ctrl Pts',(-202.488785059531,-65.554899262159,13.5774579011167));
#15206=CARTESIAN_POINT('Ctrl Pts',(-202.671070348432,-66.1140747088951,
13.5423324997414));
#15207=CARTESIAN_POINT('Ctrl Pts',(-203.011093973612,-66.5502974671019,
13.5072070983661));
#15208=CARTESIAN_POINT('Ctrl Pts',(-203.523852836765,-67.2081255384944,
13.4542376587646));
#15209=CARTESIAN_POINT('Ctrl Pts',(-204.395323300017,-67.5863477976313,
13.4012682191632));
#15210=CARTESIAN_POINT('Ctrl Pts',(-205.226028173268,-67.5115892744489,
13.3482987795618));
#15211=CARTESIAN_POINT('Ctrl Pts',(-206.056733046519,-67.4368307512664,
13.2953293399603));
#15212=CARTESIAN_POINT('Ctrl Pts',(-206.846672329768,-66.9090914457645,
13.2423599003589));
#15213=CARTESIAN_POINT('Ctrl Pts',(-207.233742270005,-66.1702841064326,
13.1893904607575));
#15214=CARTESIAN_POINT('Ctrl Pts',(-207.620812210242,-65.4314767671007,
13.136421021156));
#15215=CARTESIAN_POINT('Ctrl Pts',(-207.605012807466,-64.4816013939387,
13.0834515815546));
#15216=CARTESIAN_POINT('Ctrl Pts',(-207.193586419647,-63.7560755496928,
13.0304821419532));
#15217=CARTESIAN_POINT('Ctrl Pts',(-206.782160031828,-63.030549705447,12.9775127023517));
#15218=CARTESIAN_POINT('Ctrl Pts',(-205.975106658967,-62.5293733901171,
12.9245432627503));
#15219=CARTESIAN_POINT('Ctrl Pts',(-205.142375057033,-62.4822830258936,
12.8715738231488));
#15220=CARTESIAN_POINT('Ctrl Pts',(-204.309643455099,-62.43519266167,12.8186043835474));
#15221=CARTESIAN_POINT('Ctrl Pts',(-203.451233624093,-62.8421882485527,
12.765634943946));
#15222=CARTESIAN_POINT('Ctrl Pts',(-202.960635833421,-63.5167052839601,
12.7126655043445));
#15223=CARTESIAN_POINT('Ctrl Pts',(-202.65165196471,-63.9415235099572,12.6793047703937));
#15224=CARTESIAN_POINT('Ctrl Pts',(-202.48856510167,-64.4724572895867,12.6459440364428));
#15225=CARTESIAN_POINT('Ctrl Pts',(-202.485436300316,-65.0016271999185,
12.612583302492));
#15226=CARTESIAN_POINT('Origin',(-205.,-65.,9.));
#15227=CARTESIAN_POINT('',(-202.478899831684,-65.0011462762536,11.612583302492));
#15228=CARTESIAN_POINT('',(-202.480895630158,-64.9978964133877,11.887416697508));
#15229=CARTESIAN_POINT('',(-202.4825,-65.,9.));
#15230=CARTESIAN_POINT('Ctrl Pts',(-202.480895630158,-64.9978964133877,
11.887416697508));
#15231=CARTESIAN_POINT('Ctrl Pts',(-202.479598437047,-64.8530702325355,
11.8965890644261));
#15232=CARTESIAN_POINT('Ctrl Pts',(-202.491010825932,-64.7084483834877,
11.9057614313441));
#15233=CARTESIAN_POINT('Ctrl Pts',(-202.51585765942,-64.566172707857,11.9149337982622));
#15234=CARTESIAN_POINT('Ctrl Pts',(-202.659345469871,-63.7445458721226,
11.9679032378636));
#15235=CARTESIAN_POINT('Ctrl Pts',(-203.25086383697,-63.001162492897,12.020872677465));
#15236=CARTESIAN_POINT('Ctrl Pts',(-204.019264046879,-62.6767853568972,
12.0738421170665));
#15237=CARTESIAN_POINT('Ctrl Pts',(-204.787664256787,-62.3524082208974,
12.1268115566679));
#15238=CARTESIAN_POINT('Ctrl Pts',(-205.732946309504,-62.4470373281234,
12.1797809962694));
#15239=CARTESIAN_POINT('Ctrl Pts',(-206.421798194676,-62.9172952246455,
12.2327504358708));
#15240=CARTESIAN_POINT('Ctrl Pts',(-207.110650079848,-63.3875531211675,
12.2857198754722));
#15241=CARTESIAN_POINT('Ctrl Pts',(-207.543071797474,-64.2334398069855,
12.3386893150737));
#15242=CARTESIAN_POINT('Ctrl Pts',(-207.520843648739,-65.0672055524758,
12.3916587546751));
#15243=CARTESIAN_POINT('Ctrl Pts',(-207.498615500004,-65.9009712979661,
12.4446281942765));
#15244=CARTESIAN_POINT('Ctrl Pts',(-207.021737484906,-66.7226161031286,
12.497597633878));
#15245=CARTESIAN_POINT('Ctrl Pts',(-206.308807820586,-67.1555025809437,
12.5505670734794));
#15246=CARTESIAN_POINT('Ctrl Pts',(-205.595878156265,-67.5883890587588,
12.6035365130808));
#15247=CARTESIAN_POINT('Ctrl Pts',(-204.646896842722,-67.6325172092266,
12.6565059526823));
#15248=CARTESIAN_POINT('Ctrl Pts',(-203.896871610796,-67.2676589347991,
12.7094753922837));
#15249=CARTESIAN_POINT('Ctrl Pts',(-203.14684637887,-66.9028006603717,12.7624448318852));
#15250=CARTESIAN_POINT('Ctrl Pts',(-202.595777228561,-66.1289559610491,
12.8154142714866));
#15251=CARTESIAN_POINT('Ctrl Pts',(-202.496271178786,-65.3008509224064,
12.868383711088));
#15252=CARTESIAN_POINT('Ctrl Pts',(-202.484353002895,-65.2016659831068,
12.8747280398947));
#15253=CARTESIAN_POINT('Ctrl Pts',(-202.478912798845,-65.1017026432918,
12.8810723687013));
#15254=CARTESIAN_POINT('Ctrl Pts',(-202.47967327723,-65.0016558771702,12.887416697508));
#15255=CARTESIAN_POINT('Ctrl Pts',(-202.485436300316,-65.0016271999185,
12.612583302492));
#15256=CARTESIAN_POINT('Ctrl Pts',(-202.483597259698,-65.3126616341767,
12.5929745968414));
#15257=CARTESIAN_POINT('Ctrl Pts',(-202.537021007432,-65.6230866816078,
12.5733658911908));
#15258=CARTESIAN_POINT('Ctrl Pts',(-202.64856288418,-65.9109955592103,12.5537571855402));
#15259=CARTESIAN_POINT('Ctrl Pts',(-202.949873475951,-66.6887303151208,
12.5007877459388));
#15260=CARTESIAN_POINT('Ctrl Pts',(-203.675280409832,-67.3021613430098,
12.4478183063374));
#15261=CARTESIAN_POINT('Ctrl Pts',(-204.492261201195,-67.4700952877871,
12.3948488667359));
#15262=CARTESIAN_POINT('Ctrl Pts',(-205.309241992558,-67.6380292325644,
12.3418794271345));
#15263=CARTESIAN_POINT('Ctrl Pts',(-206.217796641404,-67.36046609423,12.288909987533));
#15264=CARTESIAN_POINT('Ctrl Pts',(-206.801448774064,-66.7646392642643,
12.2359405479316));
#15265=CARTESIAN_POINT('Ctrl Pts',(-207.385100906723,-66.1688124342986,
12.1829711083302));
#15266=CARTESIAN_POINT('Ctrl Pts',(-207.643850523198,-65.2547219127016,
12.1300016687287));
#15267=CARTESIAN_POINT('Ctrl Pts',(-207.459088245291,-64.4413816862725,
12.0770322291273));
#15268=CARTESIAN_POINT('Ctrl Pts',(-207.274325967383,-63.6280414598435,
12.0240627895259));
#15269=CARTESIAN_POINT('Ctrl Pts',(-206.646051795095,-62.9154515285825,
11.9710933499244));
#15270=CARTESIAN_POINT('Ctrl Pts',(-205.862263097956,-62.6302591347446,
11.918123910323));
#15271=CARTESIAN_POINT('Ctrl Pts',(-205.078474400818,-62.3450667409066,
11.8651544707216));
#15272=CARTESIAN_POINT('Ctrl Pts',(-204.13917117883,-62.4872718844917,11.8121850311201));
#15273=CARTESIAN_POINT('Ctrl Pts',(-203.474924779752,-62.9916885223792,
11.7592155915187));
#15274=CARTESIAN_POINT('Ctrl Pts',(-202.861992928812,-63.4571378254309,
11.7103381618431));
#15275=CARTESIAN_POINT('Ctrl Pts',(-202.483261883573,-64.2309969432331,
11.6614607321676));
#15276=CARTESIAN_POINT('Ctrl Pts',(-202.478899831684,-65.0011462762536,
11.612583302492));
#15277=CARTESIAN_POINT('Origin',(-205.,-65.,9.));
#15278=CARTESIAN_POINT('',(-202.481967477543,-64.9977164154893,10.612583302492));
#15279=CARTESIAN_POINT('',(-202.486473126263,-64.9995333153038,10.887416697508));
#15280=CARTESIAN_POINT('',(-202.4825,-65.,9.));
#15281=CARTESIAN_POINT('Ctrl Pts',(-202.486473126263,-64.9995333153038,
10.887416697508));
#15282=CARTESIAN_POINT('Ctrl Pts',(-202.485824907356,-64.6075097677981,
10.9121057601508));
#15283=CARTESIAN_POINT('Ctrl Pts',(-202.57198392834,-64.2157559153882,10.9367948227936));
#15284=CARTESIAN_POINT('Ctrl Pts',(-202.746442451943,-63.8683429559854,
10.9614838854363));
#15285=CARTESIAN_POINT('Ctrl Pts',(-203.120736541707,-63.1229817393159,
11.0144533250378));
#15286=CARTESIAN_POINT('Ctrl Pts',(-203.901473783378,-62.5817219250026,
11.0674227646392));
#15287=CARTESIAN_POINT('Ctrl Pts',(-204.730768588446,-62.4926739871521,
11.1203922042406));
#15288=CARTESIAN_POINT('Ctrl Pts',(-205.560063393513,-62.4036260493017,
11.1733616438421));
#15289=CARTESIAN_POINT('Ctrl Pts',(-206.437915761975,-62.7667899879141,
11.2263310834435));
#15290=CARTESIAN_POINT('Ctrl Pts',(-206.961923073917,-63.4156934830335,
11.279300523045));
#15291=CARTESIAN_POINT('Ctrl Pts',(-207.485930385859,-64.0645969781529,
11.3322699626464));
#15292=CARTESIAN_POINT('Ctrl Pts',(-207.65609264128,-64.9992400297792,11.3852394022478));
#15293=CARTESIAN_POINT('Ctrl Pts',(-207.39440841323,-65.7911874862032,11.4382088418493));
#15294=CARTESIAN_POINT('Ctrl Pts',(-207.13272418518,-66.5831349426273,11.4911782814507));
#15295=CARTESIAN_POINT('Ctrl Pts',(-206.439193473658,-67.2323868038489,
11.5441477210521));
#15296=CARTESIAN_POINT('Ctrl Pts',(-205.631726881101,-67.441329644961,11.5971171606536));
#15297=CARTESIAN_POINT('Ctrl Pts',(-204.824260288545,-67.650272486073,11.650086600255));
#15298=CARTESIAN_POINT('Ctrl Pts',(-203.902857814954,-67.4189063070754,
11.7030560398564));
#15299=CARTESIAN_POINT('Ctrl Pts',(-203.28988520506,-66.853288071455,11.7560254794579));
#15300=CARTESIAN_POINT('Ctrl Pts',(-202.783057000902,-66.3856141983139,
11.7998225521413));
#15301=CARTESIAN_POINT('Ctrl Pts',(-202.487089588759,-65.6894259636016,
11.8436196248246));
#15302=CARTESIAN_POINT('Ctrl Pts',(-202.480895630158,-64.9978964133877,
11.887416697508));
#15303=CARTESIAN_POINT('Ctrl Pts',(-202.478899831684,-65.0011462762536,
11.612583302492));
#15304=CARTESIAN_POINT('Ctrl Pts',(-202.478534641458,-65.0656230446933,
11.6084912925661));
#15305=CARTESIAN_POINT('Ctrl Pts',(-202.480793406997,-65.1300738112168,
11.6043992826403));
#15306=CARTESIAN_POINT('Ctrl Pts',(-202.485758378021,-65.1943154262143,
11.6003072727144));
#15307=CARTESIAN_POINT('Ctrl Pts',(-202.550027951534,-66.0258975599723,
11.547337833113));
#15308=CARTESIAN_POINT('Ctrl Pts',(-203.067756674727,-66.8224336952987,
11.4943683935115));
#15309=CARTESIAN_POINT('Ctrl Pts',(-203.801620594161,-67.2187961191196,
11.4413989539101));
#15310=CARTESIAN_POINT('Ctrl Pts',(-204.535484513596,-67.6151585429404,
11.3884295143086));
#15311=CARTESIAN_POINT('Ctrl Pts',(-205.485483629272,-67.6113472552559,
11.3354600747072));
#15312=CARTESIAN_POINT('Ctrl Pts',(-206.216143655536,-67.2091093290415,
11.2824906351058));
#15313=CARTESIAN_POINT('Ctrl Pts',(-206.9468036818,-66.8068714028271,11.2295211955043));
#15314=CARTESIAN_POINT('Ctrl Pts',(-207.458124618651,-66.0062068380828,
11.1765517559029));
#15315=CARTESIAN_POINT('Ctrl Pts',(-207.515719806102,-65.1741357968564,
11.1235823163015));
#15316=CARTESIAN_POINT('Ctrl Pts',(-207.573314993552,-64.3420647556299,
11.0706128767));
#15317=CARTESIAN_POINT('Ctrl Pts',(-207.177184431601,-63.4785872379213,
11.0176434370986));
#15318=CARTESIAN_POINT('Ctrl Pts',(-206.508912156113,-62.9795165123932,
10.9646739974972));
#15319=CARTESIAN_POINT('Ctrl Pts',(-205.840639880625,-62.4804457868651,
10.9117045578957));
#15320=CARTESIAN_POINT('Ctrl Pts',(-204.9002258916,-62.3457818535176,10.8587351182943));
#15321=CARTESIAN_POINT('Ctrl Pts',(-204.1187507062,-62.6372539068417,10.8057656786929));
#15322=CARTESIAN_POINT('Ctrl Pts',(-203.3372755208,-62.9287259601658,10.7527962390914));
#15323=CARTESIAN_POINT('Ctrl Pts',(-202.714739139025,-63.6463340001615,
10.69982679949));
#15324=CARTESIAN_POINT('Ctrl Pts',(-202.536508759301,-64.4611305115731,
10.6468573598885));
#15325=CARTESIAN_POINT('Ctrl Pts',(-202.498067233329,-64.6368694697899,
10.6354326740897));
#15326=CARTESIAN_POINT('Ctrl Pts',(-202.480294730592,-64.8171296155769,
10.6240079882908));
#15327=CARTESIAN_POINT('Ctrl Pts',(-202.481967477543,-64.9977164154893,
10.612583302492));
#15328=CARTESIAN_POINT('Origin',(-205.,-65.,9.));
#15329=CARTESIAN_POINT('',(-202.48654680791,-65.0001194272881,9.61258330249198));
#15330=CARTESIAN_POINT('',(-202.482611587334,-65.0023130412151,9.88741669750802));
#15331=CARTESIAN_POINT('',(-202.4825,-65.,9.));
#15332=CARTESIAN_POINT('Ctrl Pts',(-202.482611587334,-65.0023130412151,
9.88741669750802));
#15333=CARTESIAN_POINT('Ctrl Pts',(-202.488432663582,-64.3663757716566,
9.92762245587551));
#15334=CARTESIAN_POINT('Ctrl Pts',(-202.73327779399,-63.7264479410027,9.96782821424301));
#15335=CARTESIAN_POINT('Ctrl Pts',(-203.168440123924,-63.2666339947897,
10.0080339726105));
#15336=CARTESIAN_POINT('Ctrl Pts',(-203.741748666983,-62.6608479571479,
10.0610034122119));
#15337=CARTESIAN_POINT('Ctrl Pts',(-204.645390451181,-62.3676852839176,
10.1139728518134));
#15338=CARTESIAN_POINT('Ctrl Pts',(-205.46514113255,-62.5215301061983,10.1669422914148));
#15339=CARTESIAN_POINT('Ctrl Pts',(-206.284891813918,-62.675374928479,10.2199117310162));
#15340=CARTESIAN_POINT('Ctrl Pts',(-207.020751392457,-63.2762272462707,
10.2728811706177));
#15341=CARTESIAN_POINT('Ctrl Pts',(-207.33540594964,-64.0486597148988,10.3258506102191));
#15342=CARTESIAN_POINT('Ctrl Pts',(-207.650060506823,-64.8210921835268,
10.3788200498206));
#15343=CARTESIAN_POINT('Ctrl Pts',(-207.543510042649,-65.7651048029912,
10.431789489422));
#15344=CARTESIAN_POINT('Ctrl Pts',(-207.06459669445,-66.4479674640464,10.4847589290234));
#15345=CARTESIAN_POINT('Ctrl Pts',(-206.585683346251,-67.1308301251015,
10.5377283686249));
#15346=CARTESIAN_POINT('Ctrl Pts',(-205.734407114026,-67.5525428277475,
10.5906978082263));
#15347=CARTESIAN_POINT('Ctrl Pts',(-204.900988265359,-67.5197948257892,
10.6436672478277));
#15348=CARTESIAN_POINT('Ctrl Pts',(-204.067569416691,-67.4870468238309,
10.6966366874292));
#15349=CARTESIAN_POINT('Ctrl Pts',(-203.25200795158,-66.9998381172684,10.7496061270306));
#15350=CARTESIAN_POINT('Ctrl Pts',(-202.828152687953,-66.2815024544743,
10.802575566632));
#15351=CARTESIAN_POINT('Ctrl Pts',(-202.601856417471,-65.8979831369297,
10.8308559435907));
#15352=CARTESIAN_POINT('Ctrl Pts',(-202.487215636228,-65.4485812949919,
10.8591363205494));
#15353=CARTESIAN_POINT('Ctrl Pts',(-202.486473126263,-64.9995333153038,
10.887416697508));
#15354=CARTESIAN_POINT('Ctrl Pts',(-202.481967477543,-64.9977164154893,
10.612583302492));
#15355=CARTESIAN_POINT('Ctrl Pts',(-202.488050258416,-65.6544026714131,
10.5710385486894));
#15356=CARTESIAN_POINT('Ctrl Pts',(-202.75126577681,-66.3154084126017,10.5294937948868));
#15357=CARTESIAN_POINT('Ctrl Pts',(-203.212768047943,-66.7790366404615,
10.4879490410842));
#15358=CARTESIAN_POINT('Ctrl Pts',(-203.801182093982,-67.3701612751106,
10.4349796014828));
#15359=CARTESIAN_POINT('Ctrl Pts',(-204.711934563733,-67.6404255615813,
10.3820101618814));
#15360=CARTESIAN_POINT('Ctrl Pts',(-205.527541614709,-67.4659418612995,
10.3290407222799));
#15361=CARTESIAN_POINT('Ctrl Pts',(-206.343148665684,-67.2914581610176,
10.2760712826785));
#15362=CARTESIAN_POINT('Ctrl Pts',(-207.063610297884,-66.6722264739832,
10.2231018430771));
#15363=CARTESIAN_POINT('Ctrl Pts',(-207.358670925333,-65.8920991450205,
10.1701324034756));
#15364=CARTESIAN_POINT('Ctrl Pts',(-207.653731552782,-65.1119718160577,
10.1171629638742));
#15365=CARTESIAN_POINT('Ctrl Pts',(-207.523391175481,-64.1709488451667,
10.0641935242728));
#15366=CARTESIAN_POINT('Ctrl Pts',(-207.027397093989,-63.5003899033944,
10.0112240846713));
#15367=CARTESIAN_POINT('Ctrl Pts',(-206.531403012498,-62.829830961622,9.95825464506989));
#15368=CARTESIAN_POINT('Ctrl Pts',(-205.669755226818,-62.4297360489682,
9.90528520546845));
#15369=CARTESIAN_POINT('Ctrl Pts',(-204.837428266674,-62.4835064375044,
9.85231576586702));
#15370=CARTESIAN_POINT('Ctrl Pts',(-204.005101306531,-62.5372768260406,
9.79934632626558));
#15371=CARTESIAN_POINT('Ctrl Pts',(-203.202095171924,-63.0449125157668,
9.74637688666414));
#15372=CARTESIAN_POINT('Ctrl Pts',(-202.796503387442,-63.7737161433821,
9.69340744706271));
#15373=CARTESIAN_POINT('Ctrl Pts',(-202.590210795132,-64.1444011409031,
9.66646606553913));
#15374=CARTESIAN_POINT('Ctrl Pts',(-202.486727528942,-64.5723013010034,
9.63952468401556));
#15375=CARTESIAN_POINT('Ctrl Pts',(-202.48654680791,-65.0001194272881,9.61258330249198));
#15376=CARTESIAN_POINT('Origin',(-205.,-65.,9.));
#15377=CARTESIAN_POINT('',(-202.481528147891,-65.0022302324439,8.61258330249198));
#15378=CARTESIAN_POINT('',(-202.478564020843,-64.9992065504904,8.88741669750802));
#15379=CARTESIAN_POINT('',(-202.4825,-65.,9.));
#15380=CARTESIAN_POINT('Ctrl Pts',(-202.478564020843,-64.9992065504904,
8.88741669750802));
#15381=CARTESIAN_POINT('Ctrl Pts',(-202.478385164604,-64.9558433406332,
8.8901697119988));
#15382=CARTESIAN_POINT('Ctrl Pts',(-202.479406771777,-64.9124887333215,
8.89292272648958));
#15383=CARTESIAN_POINT('Ctrl Pts',(-202.481655288571,-64.8691978513664,
8.89567574098036));
#15384=CARTESIAN_POINT('Ctrl Pts',(-202.52491792845,-64.03625862613,8.94864518058179));
#15385=CARTESIAN_POINT('Ctrl Pts',(-203.022379735769,-63.2269103837877,
9.00161462018323));
#15386=CARTESIAN_POINT('Ctrl Pts',(-203.746006998067,-62.8121538356702,
9.05458405978466));
#15387=CARTESIAN_POINT('Ctrl Pts',(-204.469634260364,-62.3973972875527,
9.1075534993861));
#15388=CARTESIAN_POINT('Ctrl Pts',(-205.41942697764,-62.3772324336601,9.16052293898754));
#15389=CARTESIAN_POINT('Ctrl Pts',(-206.160005476114,-62.7609027303274,
9.21349237858897));
#15390=CARTESIAN_POINT('Ctrl Pts',(-206.900583974588,-63.1445730269947,
9.26646181819041));
#15391=CARTESIAN_POINT('Ctrl Pts',(-207.43194825426,-63.932078474222,9.31943125779184));
#15392=CARTESIAN_POINT('Ctrl Pts',(-207.510523898802,-64.7624309758931,
9.37240069739327));
#15393=CARTESIAN_POINT('Ctrl Pts',(-207.589099543344,-65.5927834775642,
9.42537013699471));
#15394=CARTESIAN_POINT('Ctrl Pts',(-207.214886552757,-66.4659830336792,
9.47833957659615));
#15395=CARTESIAN_POINT('Ctrl Pts',(-206.559422070674,-66.9817598475003,
9.53130901619758));
#15396=CARTESIAN_POINT('Ctrl Pts',(-205.903957588592,-67.4975366613213,
9.58427845579902));
#15397=CARTESIAN_POINT('Ctrl Pts',(-204.967241615015,-67.6558907328485,
9.63724789540045));
#15398=CARTESIAN_POINT('Ctrl Pts',(-204.178659517491,-67.3842334406392,
9.69021733500189));
#15399=CARTESIAN_POINT('Ctrl Pts',(-203.390077419966,-67.1125761484299,
9.74318677460333));
#15400=CARTESIAN_POINT('Ctrl Pts',(-202.749629198494,-66.410907492484,9.79615621420476));
#15401=CARTESIAN_POINT('Ctrl Pts',(-202.550892738719,-65.6008684634844,
9.8491256538062));
#15402=CARTESIAN_POINT('Ctrl Pts',(-202.503004582053,-65.4056789347486,
9.86188933504014));
#15403=CARTESIAN_POINT('Ctrl Pts',(-202.480763634088,-65.2041970728315,
9.87465301627408));
#15404=CARTESIAN_POINT('Ctrl Pts',(-202.482611587334,-65.0023130412151,
9.88741669750802));
#15405=CARTESIAN_POINT('Ctrl Pts',(-202.48654680791,-65.0001194272881,9.61258330249198));
#15406=CARTESIAN_POINT('Ctrl Pts',(-202.486372213392,-65.4134343505764,
9.58655524441412));
#15407=CARTESIAN_POINT('Ctrl Pts',(-202.582614889168,-65.8266727077302,
9.56052718633626));
#15408=CARTESIAN_POINT('Ctrl Pts',(-202.775719574576,-66.188169183086,9.5344991282584));
#15409=CARTESIAN_POINT('Ctrl Pts',(-203.168704980553,-66.9238470296702,
9.48152968865696));
#15410=CARTESIAN_POINT('Ctrl Pts',(-203.962853226864,-67.4452311573341,
9.42856024905553));
#15411=CARTESIAN_POINT('Ctrl Pts',(-204.794131195417,-67.5133219956579,
9.37559080945409));
#15412=CARTESIAN_POINT('Ctrl Pts',(-205.62540916397,-67.5814128339818,9.32262136985265));
#15413=CARTESIAN_POINT('Ctrl Pts',(-206.493816854764,-67.1962103829656,
9.26965193025122));
#15414=CARTESIAN_POINT('Ctrl Pts',(-207.001281035346,-66.534289293491,9.21668249064978));
#15415=CARTESIAN_POINT('Ctrl Pts',(-207.508745215928,-65.8723682040165,
9.16371305104835));
#15416=CARTESIAN_POINT('Ctrl Pts',(-207.655265886299,-64.9337284760836,
9.11074361144692));
#15417=CARTESIAN_POINT('Ctrl Pts',(-207.373678789975,-64.1486373154858,
9.05777417184549));
#15418=CARTESIAN_POINT('Ctrl Pts',(-207.092091693651,-63.3635461548879,
9.00480473224405));
#15419=CARTESIAN_POINT('Ctrl Pts',(-206.382396830632,-62.7320035616251,
8.95183529264261));
#15420=CARTESIAN_POINT('Ctrl Pts',(-205.569914360071,-62.5435051311385,
8.89886585304118));
#15421=CARTESIAN_POINT('Ctrl Pts',(-204.75743188951,-62.3550067006518,8.84589641343974));
#15422=CARTESIAN_POINT('Ctrl Pts',(-203.842161811406,-62.6095524329414,
8.79292697383831));
#15423=CARTESIAN_POINT('Ctrl Pts',(-203.243658814669,-63.1904599868281,
8.73995753423687));
#15424=CARTESIAN_POINT('Ctrl Pts',(-202.763923958874,-63.6560910749164,
8.69749945698857));
#15425=CARTESIAN_POINT('Ctrl Pts',(-202.487710433184,-64.3314080676777,
8.65504137974028));
#15426=CARTESIAN_POINT('Ctrl Pts',(-202.481528147891,-65.0022302324439,
8.61258330249198));
#15427=CARTESIAN_POINT('Origin',(-205.,-65.,9.));
#15428=CARTESIAN_POINT('',(-202.479185579191,-64.9986328469134,7.61258330249198));
#15429=CARTESIAN_POINT('',(-202.484985611247,-64.9981409264881,7.88741669750801));
#15430=CARTESIAN_POINT('',(-202.4825,-65.,9.));
#15431=CARTESIAN_POINT('Ctrl Pts',(-202.484985611247,-64.9981409264881,
7.88741669750801));
#15432=CARTESIAN_POINT('Ctrl Pts',(-202.483005664854,-64.7084761452466,
7.90568640772351));
#15433=CARTESIAN_POINT('Ctrl Pts',(-202.529198919473,-64.4194234219896,
7.92395611793902));
#15434=CARTESIAN_POINT('Ctrl Pts',(-202.626321234454,-64.1486373242474,
7.94222582815452));
#15435=CARTESIAN_POINT('Ctrl Pts',(-202.90790832788,-63.3635461717291,7.99519526775595));
#15436=CARTESIAN_POINT('Ctrl Pts',(-203.617603183594,-62.7320035849656,
8.04816470735739));
#15437=CARTESIAN_POINT('Ctrl Pts',(-204.430085645794,-62.5435051564189,
8.10113414695882));
#15438=CARTESIAN_POINT('Ctrl Pts',(-205.242568107994,-62.3550067278721,
8.15410358656026));
#15439=CARTESIAN_POINT('Ctrl Pts',(-206.157838176679,-62.6095524575421,
8.20707302616169));
#15440=CARTESIAN_POINT('Ctrl Pts',(-206.756341167256,-63.1904600054505,
8.26004246576313));
#15441=CARTESIAN_POINT('Ctrl Pts',(-207.354844157833,-63.771367553359,8.31301190536457));
#15442=CARTESIAN_POINT('Ctrl Pts',(-207.636580070302,-64.6786369195059,
8.365981344966));
#15443=CARTESIAN_POINT('Ctrl Pts',(-207.472402736839,-65.4963808966307,
8.41895078456743));
#15444=CARTESIAN_POINT('Ctrl Pts',(-207.308225403377,-66.3141248737555,
8.47192022416887));
#15445=CARTESIAN_POINT('Ctrl Pts',(-206.698134823983,-67.0423434618581,
8.52488966377031));
#15446=CARTESIAN_POINT('Ctrl Pts',(-205.921793110823,-67.3472253297266,
8.57785910337174));
#15447=CARTESIAN_POINT('Ctrl Pts',(-205.145451397663,-67.652107197595,8.63082854297318));
#15448=CARTESIAN_POINT('Ctrl Pts',(-204.202858550738,-67.5336523452293,
8.68379798257461));
#15449=CARTESIAN_POINT('Ctrl Pts',(-203.526093863495,-67.0461598149813,
8.73676742217605));
#15450=CARTESIAN_POINT('Ctrl Pts',(-202.88450309927,-66.5840040451373,8.7869838472867));
#15451=CARTESIAN_POINT('Ctrl Pts',(-202.481826452252,-65.790174192559,8.83720027239736));
#15452=CARTESIAN_POINT('Ctrl Pts',(-202.478564020843,-64.9992065504904,
8.88741669750802));
#15453=CARTESIAN_POINT('Ctrl Pts',(-202.481528147891,-65.0022302324439,
8.61258330249198));
#15454=CARTESIAN_POINT('Ctrl Pts',(-202.479997597166,-65.168305931236,8.60207194013884));
#15455=CARTESIAN_POINT('Ctrl Pts',(-202.495017556434,-65.3341061371053,
8.5915605777857));
#15456=CARTESIAN_POINT('Ctrl Pts',(-202.527597237717,-65.4963809017392,
8.58104921543256));
#15457=CARTESIAN_POINT('Ctrl Pts',(-202.691774572869,-66.3141248872796,
8.52807977583112));
#15458=CARTESIAN_POINT('Ctrl Pts',(-203.301865158541,-67.0423434828765,
8.47511033622969));
#15459=CARTESIAN_POINT('Ctrl Pts',(-204.078206879691,-67.3472253538825,
8.42214089662826));
#15460=CARTESIAN_POINT('Ctrl Pts',(-204.85454860084,-67.6521072248885,8.36917145702682));
#15461=CARTESIAN_POINT('Ctrl Pts',(-205.797141457466,-67.5336523713038,
8.31620201742538));
#15462=CARTESIAN_POINT('Ctrl Pts',(-206.473906151673,-67.0461598360388,
8.26323257782395));
#15463=CARTESIAN_POINT('Ctrl Pts',(-207.150670845881,-66.5586673007738,
8.21026313822251));
#15464=CARTESIAN_POINT('Ctrl Pts',(-207.561607377671,-65.7021370838286,
8.15729369862108));
#15465=CARTESIAN_POINT('Ctrl Pts',(-207.518344737346,-64.8691978500202,
8.10432425901964));
#15466=CARTESIAN_POINT('Ctrl Pts',(-207.475082097022,-64.0362586162118,
8.05135481941821));
#15467=CARTESIAN_POINT('Ctrl Pts',(-206.977620284583,-63.2269103655403,
7.99838537981677));
#15468=CARTESIAN_POINT('Ctrl Pts',(-206.253993014839,-62.8121538131544,
7.94541594021533));
#15469=CARTESIAN_POINT('Ctrl Pts',(-205.530365745094,-62.3973972607686,
7.89244650061389));
#15470=CARTESIAN_POINT('Ctrl Pts',(-204.580573018043,-62.3772324066685,
7.83947706101246));
#15471=CARTESIAN_POINT('Ctrl Pts',(-203.839994511948,-62.7609027072843,
7.78650762141103));
#15472=CARTESIAN_POINT('Ctrl Pts',(-203.099416005852,-63.1445730079001,
7.7335381818096));
#15473=CARTESIAN_POINT('Ctrl Pts',(-202.568051720712,-63.9320784632318,
7.68056874220816));
#15474=CARTESIAN_POINT('Ctrl Pts',(-202.489476075362,-64.7624309734483,
7.62759930260672));
#15475=CARTESIAN_POINT('Ctrl Pts',(-202.48205109026,-64.8408949172022,7.62259396923514));
#15476=CARTESIAN_POINT('Ctrl Pts',(-202.478669170703,-64.9197414532653,
7.61758863586356));
#15477=CARTESIAN_POINT('Ctrl Pts',(-202.479185579191,-64.9986328469134,
7.61258330249198));
#15478=CARTESIAN_POINT('Origin',(-205.,-65.,9.));
#15479=CARTESIAN_POINT('',(-202.485704986804,-64.9985525930702,6.61258330249198));
#15480=CARTESIAN_POINT('',(-202.485300085822,-65.0017052192927,6.88741669750801));
#15481=CARTESIAN_POINT('',(-202.4825,-65.,9.));
#15482=CARTESIAN_POINT('Ctrl Pts',(-202.485300085822,-65.0017052192927,
6.88741669750801));
#15483=CARTESIAN_POINT('Ctrl Pts',(-202.488631949774,-64.465856140259,6.92120310344824));
#15484=CARTESIAN_POINT('Ctrl Pts',(-202.656234520208,-63.9281040224856,
6.95498950938846));
#15485=CARTESIAN_POINT('Ctrl Pts',(-202.972602926875,-63.5003899188273,
6.98877591532868));
#15486=CARTESIAN_POINT('Ctrl Pts',(-203.468597003262,-62.8298309839558,
7.04174535493012));
#15487=CARTESIAN_POINT('Ctrl Pts',(-204.330244780075,-62.4297360754195,
7.09471479453155));
#15488=CARTESIAN_POINT('Ctrl Pts',(-205.162571731653,-62.4835064634023,
7.14768423413298));
#15489=CARTESIAN_POINT('Ctrl Pts',(-205.99489868323,-62.537276851385,7.20065367373442));
#15490=CARTESIAN_POINT('Ctrl Pts',(-206.797904809573,-63.044912535887,7.25362311333586));
#15491=CARTESIAN_POINT('Ctrl Pts',(-207.203496589882,-63.773716156002,7.30659255293729));
#15492=CARTESIAN_POINT('Ctrl Pts',(-207.60908837019,-64.502519776117,7.35956199253873));
#15493=CARTESIAN_POINT('Ctrl Pts',(-207.617265804465,-65.4524913318451,
7.41253143214016));
#15494=CARTESIAN_POINT('Ctrl Pts',(-207.224280402533,-66.1881691708582,
7.46550087174159));
#15495=CARTESIAN_POINT('Ctrl Pts',(-206.831295000601,-66.9238470098713,
7.51847031134303));
#15496=CARTESIAN_POINT('Ctrl Pts',(-206.037146762462,-67.4452311321696,
7.57143975094447));
#15497=CARTESIAN_POINT('Ctrl Pts',(-205.205868802464,-67.5133219697927,
7.6244091905459));
#15498=CARTESIAN_POINT('Ctrl Pts',(-204.374590842466,-67.5814128074158,
7.67737863014734));
#15499=CARTESIAN_POINT('Ctrl Pts',(-203.506183160609,-67.1962103603639,
7.73034806974877));
#15500=CARTESIAN_POINT('Ctrl Pts',(-202.998718985249,-66.5342892777013,
7.78331750935021));
#15501=CARTESIAN_POINT('Ctrl Pts',(-202.666284477908,-66.1006716556147,
7.81801723873614));
#15502=CARTESIAN_POINT('Ctrl Pts',(-202.488746130884,-65.5483023359006,
7.85271696812208));
#15503=CARTESIAN_POINT('Ctrl Pts',(-202.484985611247,-64.9981409264881,
7.88741669750801));
#15504=CARTESIAN_POINT('Ctrl Pts',(-202.479185579191,-64.9986328469134,
7.61258330249198));
#15505=CARTESIAN_POINT('Ctrl Pts',(-202.484134115022,-65.7546174946183,
7.56461919626212));
#15506=CARTESIAN_POINT('Ctrl Pts',(-202.847051370263,-66.5147212446862,
7.51665509003227));
#15507=CARTESIAN_POINT('Ctrl Pts',(-203.440577913277,-66.9817598678951,
7.46869098380242));
#15508=CARTESIAN_POINT('Ctrl Pts',(-204.096042402105,-67.4975366870241,
7.41572154420098));
#15509=CARTESIAN_POINT('Ctrl Pts',(-205.032758385322,-67.655890760181,7.36275210459954));
#15510=CARTESIAN_POINT('Ctrl Pts',(-205.821340490962,-67.3842334651759,
7.30978266499811));
#15511=CARTESIAN_POINT('Ctrl Pts',(-206.609922596602,-67.1125761701709,
7.25681322539667));
#15512=CARTESIAN_POINT('Ctrl Pts',(-207.250370824665,-66.410907507004,7.20384378579524));
#15513=CARTESIAN_POINT('Ctrl Pts',(-207.449107286486,-65.600868469668,7.1508743461938));
#15514=CARTESIAN_POINT('Ctrl Pts',(-207.647843748306,-64.7908294323321,
7.09790490659237));
#15515=CARTESIAN_POINT('Ctrl Pts',(-207.404868443885,-63.8724200208271,
7.04493546699093));
#15516=CARTESIAN_POINT('Ctrl Pts',(-206.831559894925,-63.2666339769511,
6.99196602738949));
#15517=CARTESIAN_POINT('Ctrl Pts',(-206.258251345965,-62.660847933075,6.93899658778806));
#15518=CARTESIAN_POINT('Ctrl Pts',(-205.354609552468,-62.3676852568278,
6.88602714818662));
#15519=CARTESIAN_POINT('Ctrl Pts',(-204.534858862664,-62.5215300806918,
6.83305770858519));
#15520=CARTESIAN_POINT('Ctrl Pts',(-203.715108172859,-62.6753749045558,
6.78008826898375));
#15521=CARTESIAN_POINT('Ctrl Pts',(-202.979248586747,-63.276227228531,6.72711882938232));
#15522=CARTESIAN_POINT('Ctrl Pts',(-202.664594026326,-64.0486597051084,
6.67414938978088));
#15523=CARTESIAN_POINT('Ctrl Pts',(-202.542686940035,-64.3479243731608,
6.65362736068458));
#15524=CARTESIAN_POINT('Ctrl Pts',(-202.484004060027,-64.6729437646861,
6.63310533158828));
#15525=CARTESIAN_POINT('Ctrl Pts',(-202.485704986804,-64.9985525930702,
6.61258330249198));
#15526=CARTESIAN_POINT('Origin',(-205.,-65.,9.));
#15527=CARTESIAN_POINT('',(-202.484474743425,-65.0020481251356,5.61258330249198));
#15528=CARTESIAN_POINT('',(-202.478781684044,-65.0010375248543,5.88741669750801));
#15529=CARTESIAN_POINT('',(-202.4825,-65.,9.));
#15530=CARTESIAN_POINT('Ctrl Pts',(-202.478781684044,-65.0010375248543,
5.88741669750801));
#15531=CARTESIAN_POINT('Ctrl Pts',(-202.482826051254,-64.2242774991166,
5.93671979917295));
#15532=CARTESIAN_POINT('Ctrl Pts',(-202.869070789817,-63.4440435255548,
5.9860229008379));
#15533=CARTESIAN_POINT('Ctrl Pts',(-203.491087859415,-62.9795165331866,
6.03532600250284));
#15534=CARTESIAN_POINT('Ctrl Pts',(-204.159360128026,-62.4804458127945,
6.08829544210427));
#15535=CARTESIAN_POINT('Ctrl Pts',(-205.099774107373,-62.3457818808328,
6.14126488170571));
#15536=CARTESIAN_POINT('Ctrl Pts',(-205.881249284731,-62.6372539311573,
6.19423432130715));
#15537=CARTESIAN_POINT('Ctrl Pts',(-206.662724462089,-62.9287259814817,
6.24720376090858));
#15538=CARTESIAN_POINT('Ctrl Pts',(-207.285260837457,-63.6463340140924,
6.30017320051002));
#15539=CARTESIAN_POINT('Ctrl Pts',(-207.463491215347,-64.4611305171187,
6.35314264011145));
#15540=CARTESIAN_POINT('Ctrl Pts',(-207.641721593236,-65.2759270201451,
6.40611207971288));
#15541=CARTESIAN_POINT('Ctrl Pts',(-207.375645973648,-66.1879119935872,
6.45908151931432));
#15542=CARTESIAN_POINT('Ctrl Pts',(-206.787231933664,-66.7790366221529,
6.51205095891575));
#15543=CARTESIAN_POINT('Ctrl Pts',(-206.198817893681,-67.3701612507187,
6.56502039851719));
#15544=CARTESIAN_POINT('Ctrl Pts',(-205.288065433302,-67.640425534408,6.61798983811863));
#15545=CARTESIAN_POINT('Ctrl Pts',(-204.47245839072,-67.4659418359219,6.67095927772007));
#15546=CARTESIAN_POINT('Ctrl Pts',(-203.656851348138,-67.2914581374357,
6.7239287173215));
#15547=CARTESIAN_POINT('Ctrl Pts',(-202.936389723353,-66.6722264567739,
6.77689815692293));
#15548=CARTESIAN_POINT('Ctrl Pts',(-202.64132909894,-65.8920991358397,6.82986759652437));
#15549=CARTESIAN_POINT('Ctrl Pts',(-202.53447205207,-65.6095738010406,6.84905063018558));
#15550=CARTESIAN_POINT('Ctrl Pts',(-202.483408341005,-65.3059462486174,
6.8682336638468));
#15551=CARTESIAN_POINT('Ctrl Pts',(-202.485300085822,-65.0017052192927,
6.88741669750801));
#15552=CARTESIAN_POINT('Ctrl Pts',(-202.485704986804,-64.9985525930702,
6.61258330249198));
#15553=CARTESIAN_POINT('Ctrl Pts',(-202.488394324643,-65.5133731923927,
6.58013589198685));
#15554=CARTESIAN_POINT('Ctrl Pts',(-202.642036046849,-66.0296673142372,
6.54768848148171));
#15555=CARTESIAN_POINT('Ctrl Pts',(-202.935403284303,-66.4479674789478,
6.51524107097658));
#15556=CARTESIAN_POINT('Ctrl Pts',(-203.414316637431,-67.1308301470305,
6.46227163137514));
#15557=CARTESIAN_POINT('Ctrl Pts',(-204.265592878416,-67.5525428540164,
6.40930219177371));
#15558=CARTESIAN_POINT('Ctrl Pts',(-205.09901173566,-67.5197948517211,6.35633275217227));
#15559=CARTESIAN_POINT('Ctrl Pts',(-205.932430592905,-67.4870468494258,
6.30336331257083));
#15560=CARTESIAN_POINT('Ctrl Pts',(-206.747992066409,-66.9998381378491,
6.2503938729694));
#15561=CARTESIAN_POINT('Ctrl Pts',(-207.171847334398,-66.2815024676625,
6.19742443336796));
#15562=CARTESIAN_POINT('Ctrl Pts',(-207.595702602388,-65.5631667974759,
6.14445499376652));
#15563=CARTESIAN_POINT('Ctrl Pts',(-207.627851664864,-64.6137041686792,
6.09148555416509));
#15564=CARTESIAN_POINT('Ctrl Pts',(-207.253557571248,-63.8683429443391,
6.03851611456365));
#15565=CARTESIAN_POINT('Ctrl Pts',(-206.879263477633,-63.122981719999,5.98554667496222));
#15566=CARTESIAN_POINT('Ctrl Pts',(-206.098526227927,-62.5817219001155,
5.93257723536078));
#15567=CARTESIAN_POINT('Ctrl Pts',(-205.269231414325,-62.4926739613487,
5.87960779575935));
#15568=CARTESIAN_POINT('Ctrl Pts',(-204.439936600723,-62.4036260225818,
5.82663835615791));
#15569=CARTESIAN_POINT('Ctrl Pts',(-203.562084223227,-62.7667899649316,
5.77366891655648));
#15570=CARTESIAN_POINT('Ctrl Pts',(-203.038076905892,-63.4156934667291,
5.72069947695504));
#15571=CARTESIAN_POINT('Ctrl Pts',(-202.68155896544,-63.8571868053907,5.68466075213402));
#15572=CARTESIAN_POINT('Ctrl Pts',(-202.488836240528,-64.4309492584116,
5.648622027313));
#15573=CARTESIAN_POINT('Ctrl Pts',(-202.484474743425,-65.0020481251356,
5.61258330249198));
#15574=CARTESIAN_POINT('Origin',(-205.,-65.,9.));
#15575=CARTESIAN_POINT('',(-202.478344395066,-65.0004148924675,4.61258330249198));
#15576=CARTESIAN_POINT('',(-202.482172797578,-64.9977007737485,4.88741669750801));
#15577=CARTESIAN_POINT('',(-202.4825,-65.,9.));
#15578=CARTESIAN_POINT('Ctrl Pts',(-202.482172797578,-64.9977007737485,
4.88741669750801));
#15579=CARTESIAN_POINT('Ctrl Pts',(-202.480439688195,-64.8103463528036,
4.89926705529624));
#15580=CARTESIAN_POINT('Ctrl Pts',(-202.49957664238,-64.6233426993509,4.91111741308446));
#15581=CARTESIAN_POINT('Ctrl Pts',(-202.540911780016,-64.4413816920215,
4.92296777087269));
#15582=CARTESIAN_POINT('Ctrl Pts',(-202.725674056022,-63.6280414739628,
4.97593721047413));
#15583=CARTESIAN_POINT('Ctrl Pts',(-203.353948221845,-62.9154515500352,
5.02890665007556));
#15584=CARTESIAN_POINT('Ctrl Pts',(-204.137736910917,-62.6302591591322,
5.08187608967699));
#15585=CARTESIAN_POINT('Ctrl Pts',(-204.92152559999,-62.3450667682292,5.13484552927843));
#15586=CARTESIAN_POINT('Ctrl Pts',(-205.860828812312,-62.4872719103509,
5.18781496887987));
#15587=CARTESIAN_POINT('Ctrl Pts',(-206.525075204553,-62.9916885430472,
5.2407844084813));
#15588=CARTESIAN_POINT('Ctrl Pts',(-207.189321596795,-63.4961051757435,
5.29375384808274));
#15589=CARTESIAN_POINT('Ctrl Pts',(-207.578511168956,-64.3627332990145,
5.34672328768417));
#15590=CARTESIAN_POINT('Ctrl Pts',(-207.514241596105,-65.1943154242145,
5.39969272728561));
#15591=CARTESIAN_POINT('Ctrl Pts',(-207.449972023253,-66.0258975494145,
5.45266216688704));
#15592=CARTESIAN_POINT('Ctrl Pts',(-206.932243305388,-66.8224336765435,
5.50563160648848));
#15593=CARTESIAN_POINT('Ctrl Pts',(-206.198379393506,-67.2187960962853,
5.55860104608992));
#15594=CARTESIAN_POINT('Ctrl Pts',(-205.464515481624,-67.6151585160272,
5.61157048569135));
#15595=CARTESIAN_POINT('Ctrl Pts',(-204.514516375724,-67.6113472283819,
5.66453992529279));
#15596=CARTESIAN_POINT('Ctrl Pts',(-203.78385635698,-67.209109306307,5.71750936489422));
#15597=CARTESIAN_POINT('Ctrl Pts',(-203.053196338235,-66.8068713842322,
5.77047880449566));
#15598=CARTESIAN_POINT('Ctrl Pts',(-202.541875406646,-66.0062068277278,
5.82344824409709));
#15599=CARTESIAN_POINT('Ctrl Pts',(-202.484280219788,-65.1741357950644,
5.87641768369853));
#15600=CARTESIAN_POINT('Ctrl Pts',(-202.480293705675,-65.1165430847041,
5.88008402163502));
#15601=CARTESIAN_POINT('Ctrl Pts',(-202.478480931831,-65.0587999100541,
5.88375035957152));
#15602=CARTESIAN_POINT('Ctrl Pts',(-202.478781684044,-65.0010375248543,
5.88741669750801));
#15603=CARTESIAN_POINT('Ctrl Pts',(-202.484474743425,-65.0020481251356,
5.61258330249198));
#15604=CARTESIAN_POINT('Ctrl Pts',(-202.482425745747,-65.2703459650826,
5.59565258771156));
#15605=CARTESIAN_POINT('Ctrl Pts',(-202.521948972994,-65.5380559387795,
5.57872187293115));
#15606=CARTESIAN_POINT('Ctrl Pts',(-202.605591562129,-65.7911874943456,
5.56179115815073));
#15607=CARTESIAN_POINT('Ctrl Pts',(-202.867275792872,-66.5831349589198,
5.5088217185493));
#15608=CARTESIAN_POINT('Ctrl Pts',(-203.560806511531,-67.232386826823,5.45585227894786));
#15609=CARTESIAN_POINT('Ctrl Pts',(-204.368273112397,-67.4413296700853,
5.40288283934643));
#15610=CARTESIAN_POINT('Ctrl Pts',(-205.175739713264,-67.6502725133476,
5.34991339974499));
#15611=CARTESIAN_POINT('Ctrl Pts',(-206.097142196337,-67.4189063319689,
5.29694396014355));
#15612=CARTESIAN_POINT('Ctrl Pts',(-206.710114812539,-66.8532880905275,
5.24397452054212));
#15613=CARTESIAN_POINT('Ctrl Pts',(-207.323087428742,-66.2876698490862,
5.19100508094068));
#15614=CARTESIAN_POINT('Ctrl Pts',(-207.627630178073,-65.3877995475822,
5.13803564133925));
#15615=CARTESIAN_POINT('Ctrl Pts',(-207.484142366145,-64.5661727033922,
5.08506620173781));
#15616=CARTESIAN_POINT('Ctrl Pts',(-207.340654554217,-63.7445458592023,
5.03209676213638));
#15617=CARTESIAN_POINT('Ctrl Pts',(-206.74913618103,-63.0011624723264,4.97912732253494));
#15618=CARTESIAN_POINT('Ctrl Pts',(-205.980735963214,-62.6767853329884,
4.92615788293351));
#15619=CARTESIAN_POINT('Ctrl Pts',(-205.212335745398,-62.3524081936504,
4.87318844333207));
#15620=CARTESIAN_POINT('Ctrl Pts',(-204.267053682953,-62.4470373018503,
4.82021900373063));
#15621=CARTESIAN_POINT('Ctrl Pts',(-203.578201790692,-62.9172952032119,
4.7672495641292));
#15622=CARTESIAN_POINT('Ctrl Pts',(-202.907738797946,-63.3749995710904,
4.71569414358346));
#15623=CARTESIAN_POINT('Ctrl Pts',(-202.480197907909,-64.1885455944467,
4.66413872303772));
#15624=CARTESIAN_POINT('Ctrl Pts',(-202.478344395066,-65.0004148924675,
4.61258330249198));
#15625=CARTESIAN_POINT('Origin',(-205.,-65.,9.));
#15626=CARTESIAN_POINT('',(-202.483242763103,-64.9977147872857,3.61258330249198));
#15627=CARTESIAN_POINT('',(-202.486532876632,-65.000230478593,3.88741669750801));
#15628=CARTESIAN_POINT('',(-202.4825,-65.,9.));
#15629=CARTESIAN_POINT('Ctrl Pts',(-202.486532876632,-65.000230478593,3.88741669750801));
#15630=CARTESIAN_POINT('Ctrl Pts',(-202.48688726354,-64.5656588769883,3.91478375102096));
#15631=CARTESIAN_POINT('Ctrl Pts',(-202.593847112874,-64.1309238627515,
3.94215080453391));
#15632=CARTESIAN_POINT('Ctrl Pts',(-202.806413602928,-63.7560755624945,
3.96951785804685));
#15633=CARTESIAN_POINT('Ctrl Pts',(-203.217839986513,-63.0305497257151,
4.02248729764829));
#15634=CARTESIAN_POINT('Ctrl Pts',(-204.024893351068,-62.5293734155429,
4.07545673724972));
#15635=CARTESIAN_POINT('Ctrl Pts',(-204.857624944432,-62.482283051804,4.12842617685116));
#15636=CARTESIAN_POINT('Ctrl Pts',(-205.690356537796,-62.435192688065,4.18139561645259));
#15637=CARTESIAN_POINT('Ctrl Pts',(-206.548766359968,-62.8421882707593,
4.23436505605403));
#15638=CARTESIAN_POINT('Ctrl Pts',(-207.039364145592,-63.5167052992251,
4.28733449565546));
#15639=CARTESIAN_POINT('Ctrl Pts',(-207.529961931215,-64.1912223276909,
4.3403039352569));
#15640=CARTESIAN_POINT('Ctrl Pts',(-207.652747680291,-65.1332608019282,
4.39327337485833));
#15641=CARTESIAN_POINT('Ctrl Pts',(-207.351437091621,-65.9109955498349,
4.44624281445977));
#15642=CARTESIAN_POINT('Ctrl Pts',(-207.05012650295,-66.6887302977416,4.4992122540612));
#15643=CARTESIAN_POINT('Ctrl Pts',(-206.324719576535,-67.3021613193176,
4.55218169366264));
#15644=CARTESIAN_POINT('Ctrl Pts',(-205.50773879358,-67.4700952623667,4.60515113326408));
#15645=CARTESIAN_POINT('Ctrl Pts',(-204.690758010624,-67.6380292054158,
4.65812057286551));
#15646=CARTESIAN_POINT('Ctrl Pts',(-203.782203371129,-67.3604660699379,
4.71109001246695));
#15647=CARTESIAN_POINT('Ctrl Pts',(-203.198551244476,-66.764639246104,4.76405945206838));
#15648=CARTESIAN_POINT('Ctrl Pts',(-202.745474154612,-66.3021111903028,
4.80517853388159));
#15649=CARTESIAN_POINT('Ctrl Pts',(-202.488186444403,-65.6477943743447,
4.8462976156948));
#15650=CARTESIAN_POINT('Ctrl Pts',(-202.482172797578,-64.9977007737485,
4.88741669750801));
#15651=CARTESIAN_POINT('Ctrl Pts',(-202.478344395066,-65.0004148924675,
4.61258330249198));
#15652=CARTESIAN_POINT('Ctrl Pts',(-202.478293558463,-65.0226821661311,
4.61116928343628));
#15653=CARTESIAN_POINT('Ctrl Pts',(-202.478562944938,-65.0449481784791,
4.60975526438059));
#15654=CARTESIAN_POINT('Ctrl Pts',(-202.479156325318,-65.0672055531675,
4.60834124532489));
#15655=CARTESIAN_POINT('Ctrl Pts',(-202.501384474282,-65.9009713072382,
4.55537180572346));
#15656=CARTESIAN_POINT('Ctrl Pts',(-202.978262494288,-66.7226161208565,
4.50240236612202));
#15657=CARTESIAN_POINT('Ctrl Pts',(-203.691192165945,-67.1555026031265,
4.44943292652058));
#15658=CARTESIAN_POINT('Ctrl Pts',(-204.404121837602,-67.5883890853966,
4.39646348691915));
#15659=CARTESIAN_POINT('Ctrl Pts',(-205.353103160912,-67.6325172363185,
4.34349404731772));
#15660=CARTESIAN_POINT('Ctrl Pts',(-206.103128400557,-67.2676589581362,
4.29052460771628));
#15661=CARTESIAN_POINT('Ctrl Pts',(-206.853153640202,-66.9028006799539,
4.23755516811485));
#15662=CARTESIAN_POINT('Ctrl Pts',(-207.404222796182,-66.1289559726674,
4.18458572851341));
#15663=CARTESIAN_POINT('Ctrl Pts',(-207.50372884698,-65.3008509255024,4.13161628891197));
#15664=CARTESIAN_POINT('Ctrl Pts',(-207.603234897779,-64.4727458783375,
4.07864684931054));
#15665=CARTESIAN_POINT('Ctrl Pts',(-207.251177843396,-63.5903804912942,
4.02567740970911));
#15666=CARTESIAN_POINT('Ctrl Pts',(-206.608938670144,-63.0582261268744,
3.97270797010767));
#15667=CARTESIAN_POINT('Ctrl Pts',(-205.966699496891,-62.5260717624545,
3.91973853050623));
#15668=CARTESIAN_POINT('Ctrl Pts',(-205.034278204769,-62.3441284206583,
3.86676909090479));
#15669=CARTESIAN_POINT('Ctrl Pts',(-204.239091503311,-62.59579791241,3.81379965130336));
#15670=CARTESIAN_POINT('Ctrl Pts',(-203.443904801853,-62.8474674041617,
3.76083021170192));
#15671=CARTESIAN_POINT('Ctrl Pts',(-202.785952691059,-63.5327497294614,
3.70786077210049));
#15672=CARTESIAN_POINT('Ctrl Pts',(-202.566836741692,-64.3375153003988,
3.65489133249905));
#15673=CARTESIAN_POINT('Ctrl Pts',(-202.508498926336,-64.5517775000122,
3.64078865583003));
#15674=CARTESIAN_POINT('Ctrl Pts',(-202.481267868868,-64.7745092304446,
3.626685979161));
#15675=CARTESIAN_POINT('Ctrl Pts',(-202.483242763103,-64.9977147872857,
3.61258330249198));
#15676=CARTESIAN_POINT('Origin',(-205.,-65.,9.));
#15677=CARTESIAN_POINT('',(-202.486312984545,-65.0008035915154,2.61258330249198));
#15678=CARTESIAN_POINT('',(-202.481325023787,-65.002196172282,2.88741669750801));
#15679=CARTESIAN_POINT('',(-202.4825,-65.,9.));
#15680=CARTESIAN_POINT('Ctrl Pts',(-202.481325023787,-65.002196172282,2.88741669750801));
#15681=CARTESIAN_POINT('Ctrl Pts',(-202.487529219197,-64.3247893018804,
2.93030044674568));
#15682=CARTESIAN_POINT('Ctrl Pts',(-202.769932024913,-63.6428224125831,
2.97318419598334));
#15683=CARTESIAN_POINT('Ctrl Pts',(-203.258234470432,-63.1764260021977,
3.01606794522101));
#15684=CARTESIAN_POINT('Ctrl Pts',(-203.861379189701,-62.6003393276553,
3.06903738482244));
#15685=CARTESIAN_POINT('Ctrl Pts',(-204.778662179042,-62.3531455904109,
3.12200682442388));
#15686=CARTESIAN_POINT('Ctrl Pts',(-205.589606043438,-62.5481570193482,
3.17497626402531));
#15687=CARTESIAN_POINT('Ctrl Pts',(-206.400549907833,-62.7431684482854,
3.22794570362675));
#15688=CARTESIAN_POINT('Ctrl Pts',(-207.105154647285,-63.3803850434044,
3.28091514322819));
#15689=CARTESIAN_POINT('Ctrl Pts',(-207.380433386275,-64.1677102779642,
3.33388458282962));
#15690=CARTESIAN_POINT('Ctrl Pts',(-207.655712125266,-64.9550355125241,
3.38685402243106));
#15691=CARTESIAN_POINT('Ctrl Pts',(-207.501664863796,-65.8924693865247,
3.43982346203249));
#15692=CARTESIAN_POINT('Ctrl Pts',(-206.98890600592,-66.5502974511473,3.49279290163393));
#15693=CARTESIAN_POINT('Ctrl Pts',(-206.476147148043,-67.2081255157699,
3.54576234123536));
#15694=CARTESIAN_POINT('Ctrl Pts',(-205.60467669376,-67.5863477710145,3.5987317808368));
#15695=CARTESIAN_POINT('Ctrl Pts',(-204.773971829058,-67.5115892486015,
3.65170122043824));
#15696=CARTESIAN_POINT('Ctrl Pts',(-203.943266964357,-67.4368307261884,
3.70467066003967));
#15697=CARTESIAN_POINT('Ctrl Pts',(-203.153327689236,-66.9090914261176,
3.7576400996411));
#15698=CARTESIAN_POINT('Ctrl Pts',(-202.766257752983,-66.170284094389,3.81060953924254));
#15699=CARTESIAN_POINT('Ctrl Pts',(-202.57917036777,-65.8131870457086,3.83621192533103));
#15700=CARTESIAN_POINT('Ctrl Pts',(-202.486201341108,-65.4067802711058,
3.86181431141952));
#15701=CARTESIAN_POINT('Ctrl Pts',(-202.486532876632,-65.000230478593,3.88741669750801));
#15702=CARTESIAN_POINT('Ctrl Pts',(-202.483242763103,-64.9977147872857,
3.61258330249198));
#15703=CARTESIAN_POINT('Ctrl Pts',(-202.488685541649,-65.6128659154395,
3.57371653955957));
#15704=CARTESIAN_POINT('Ctrl Pts',(-202.715960735313,-66.2316159695124,
3.53484977662716));
#15705=CARTESIAN_POINT('Ctrl Pts',(-203.125278860397,-66.6865912568974,
3.49598301369474));
#15706=CARTESIAN_POINT('Ctrl Pts',(-203.683116716411,-67.3066528258837,
3.44301357409331));
#15707=CARTESIAN_POINT('Ctrl Pts',(-204.57907221638,-67.6225271472811,3.39004413449187));
#15708=CARTESIAN_POINT('Ctrl Pts',(-205.402444366375,-67.4894191989927,
3.33707469489044));
#15709=CARTESIAN_POINT('Ctrl Pts',(-206.225816516371,-67.3563112507042,
3.284105255289));
#15710=CARTESIAN_POINT('Ctrl Pts',(-206.976605316395,-66.7742210327298,
3.23113581568757));
#15711=CARTESIAN_POINT('Ctrl Pts',(-207.310653375596,-66.009975444743,3.17816637608613));
#15712=CARTESIAN_POINT('Ctrl Pts',(-207.644701434797,-65.2457298567563,
3.1251969364847));
#15713=CARTESIAN_POINT('Ctrl Pts',(-207.562008753175,-64.2993288987573,
3.07222749688326));
#15714=CARTESIAN_POINT('Ctrl Pts',(-207.100481195153,-63.6045974878118,
3.01925805728183));
#15715=CARTESIAN_POINT('Ctrl Pts',(-206.638953637131,-62.9098660768664,
2.96628861768039));
#15716=CARTESIAN_POINT('Ctrl Pts',(-205.798591202707,-62.4668042129746,
2.91331917807895));
#15717=CARTESIAN_POINT('Ctrl Pts',(-204.964611332898,-62.4785089645746,
2.86034973847752));
#15718=CARTESIAN_POINT('Ctrl Pts',(-204.130631463088,-62.4902137161746,
2.80738029887608));
#15719=CARTESIAN_POINT('Ctrl Pts',(-203.303034157892,-62.9566850832665,
2.75441085927465));
#15720=CARTESIAN_POINT('Ctrl Pts',(-202.861185402517,-63.6640952267508,
2.70144141967321));
#15721=CARTESIAN_POINT('Ctrl Pts',(-202.614113073159,-64.0596637778368,
2.67182204727947));
#15722=CARTESIAN_POINT('Ctrl Pts',(-202.487656834806,-64.5305692119616,
2.64220267488572));
#15723=CARTESIAN_POINT('Ctrl Pts',(-202.486312984545,-65.0008035915154,
2.61258330249198));
#15724=CARTESIAN_POINT('Origin',(-205.,-65.,9.));
#15725=CARTESIAN_POINT('',(-202.480291602729,-65.0019224916823,1.61258330249198));
#15726=CARTESIAN_POINT('',(-202.479332426993,-64.9985362476049,1.88741669750801));
#15727=CARTESIAN_POINT('',(-202.4825,-65.,9.));
#15728=CARTESIAN_POINT('Ctrl Pts',(-202.479332426993,-64.9985362476049,
1.88741669750801));
#15729=CARTESIAN_POINT('Ctrl Pts',(-202.478740698757,-64.9129225001756,
1.89284770286896));
#15730=CARTESIAN_POINT('Ctrl Pts',(-202.48272375902,-64.8273644585912,1.89827870822991));
#15731=CARTESIAN_POINT('Ctrl Pts',(-202.491463034604,-64.7422950299795,
1.90370971359086));
#15732=CARTESIAN_POINT('Ctrl Pts',(-202.576698547997,-63.9125996676488,
1.9566791531923));
#15733=CARTESIAN_POINT('Ctrl Pts',(-203.114364484717,-63.1293831459998,
2.00964859279373));
#15734=CARTESIAN_POINT('Ctrl Pts',(-203.857997602776,-62.7516673617973,
2.06261803239517));
#15735=CARTESIAN_POINT('Ctrl Pts',(-204.601630720835,-62.3739515775949,
2.1155874719966));
#15736=CARTESIAN_POINT('Ctrl Pts',(-205.551231020233,-62.401736530839,2.16855691159804));
#15737=CARTESIAN_POINT('Ctrl Pts',(-206.271507118528,-62.8222858415902,
2.22152635119947));
#15738=CARTESIAN_POINT('Ctrl Pts',(-206.991783216823,-63.2428351523415,
2.27449579080091));
#15739=CARTESIAN_POINT('Ctrl Pts',(-207.482735114015,-64.0561488205997,
2.32746523040235));
#15740=CARTESIAN_POINT('Ctrl Pts',(-207.519313161291,-64.8894083635227,
2.38043467000378));
#15741=CARTESIAN_POINT('Ctrl Pts',(-207.555891208567,-65.7226679064456,
2.43340410960522));
#15742=CARTESIAN_POINT('Ctrl Pts',(-207.138095405927,-66.5758733240332,
2.48637354920665));
#15743=CARTESIAN_POINT('Ctrl Pts',(-206.457441035269,-67.057920041525,2.53934298880809));
#15744=CARTESIAN_POINT('Ctrl Pts',(-205.776786664612,-67.5399667590167,
2.59231242840953));
#15745=CARTESIAN_POINT('Ctrl Pts',(-204.833273725938,-67.6508547764125,
2.64528186801096));
#15746=CARTESIAN_POINT('Ctrl Pts',(-204.059403267518,-67.3397536362125,
2.6982513076124));
#15747=CARTESIAN_POINT('Ctrl Pts',(-203.285532809097,-67.0286524960126,
2.75122074721383));
#15748=CARTESIAN_POINT('Ctrl Pts',(-202.681304830931,-66.2955621982167,
2.80419018681527));
#15749=CARTESIAN_POINT('Ctrl Pts',(-202.523694066448,-65.4765272433986,
2.8571596264167));
#15750=CARTESIAN_POINT('Ctrl Pts',(-202.49368405727,-65.3205782091337,2.86724531678047));
#15751=CARTESIAN_POINT('Ctrl Pts',(-202.479865879124,-65.1615133044501,
2.87733100714424));
#15752=CARTESIAN_POINT('Ctrl Pts',(-202.481325023787,-65.002196172282,2.88741669750801));
#15753=CARTESIAN_POINT('Ctrl Pts',(-202.486312984545,-65.0008035915154,
2.61258330249198));
#15754=CARTESIAN_POINT('Ctrl Pts',(-202.485253576752,-65.3715070696305,
2.58923323528429));
#15755=CARTESIAN_POINT('Ctrl Pts',(-202.561948551986,-65.7417935032391,
2.5658831680766));
#15756=CARTESIAN_POINT('Ctrl Pts',(-202.718600795358,-66.0744240820748,
2.54253310086891));
#15757=CARTESIAN_POINT('Ctrl Pts',(-203.073965149126,-66.8289938740376,
2.48956366126747));
#15758=CARTESIAN_POINT('Ctrl Pts',(-203.840794062215,-67.3897845380866,
2.43659422166603));
#15759=CARTESIAN_POINT('Ctrl Pts',(-204.667577469299,-67.4997328895863,
2.3836247820646));
#15760=CARTESIAN_POINT('Ctrl Pts',(-205.494360876384,-67.6096812410859,
2.33065534246316));
#15761=CARTESIAN_POINT('Ctrl Pts',(-206.381098777463,-67.2687872800362,
2.27768590286173));
#15762=CARTESIAN_POINT('Ctrl Pts',(-206.92131542659,-66.6333146422909,2.22471646326029));
#15763=CARTESIAN_POINT('Ctrl Pts',(-207.461532075717,-65.9978420045456,
2.17174702365886));
#15764=CARTESIAN_POINT('Ctrl Pts',(-207.655227472892,-65.0677906901045,
2.11877758405742));
#15765=CARTESIAN_POINT('Ctrl Pts',(-207.413612828359,-64.2694915404195,
2.06580814445599));
#15766=CARTESIAN_POINT('Ctrl Pts',(-207.171998183825,-63.4711923907344,
2.01283870485455));
#15767=CARTESIAN_POINT('Ctrl Pts',(-206.495073497584,-62.8046454058054,
1.95986926525311));
#15768=CARTESIAN_POINT('Ctrl Pts',(-205.693137061413,-62.5753909354637,
1.90689982565168));
#15769=CARTESIAN_POINT('Ctrl Pts',(-204.891200625243,-62.346136465122,1.85393038605024));
#15770=CARTESIAN_POINT('Ctrl Pts',(-203.964252439144,-62.5541745093678,
1.80096094644881));
#15771=CARTESIAN_POINT('Ctrl Pts',(-203.337200786238,-63.104143779992,1.74799150684737));
#15772=CARTESIAN_POINT('Ctrl Pts',(-202.802880500195,-63.572780991349,1.70285543872891));
#15773=CARTESIAN_POINT('Ctrl Pts',(-202.486315214849,-64.289694612059,1.65771937061044));
#15774=CARTESIAN_POINT('Ctrl Pts',(-202.480291602729,-65.0019224916823,
1.61258330249198));
#15775=CARTESIAN_POINT('Origin',(-205.,-65.,9.));
#15776=CARTESIAN_POINT('',(-202.480232352617,-64.9981364767374,0.612583302491977));
#15777=CARTESIAN_POINT('',(-202.485823045017,-64.9986459985219,0.88741669750801));
#15778=CARTESIAN_POINT('',(-202.4825,-65.,9.));
#15779=CARTESIAN_POINT('',(-206.913465996665,-63.364012796625,0.));
#15780=CARTESIAN_POINT('Ctrl Pts',(-202.480232352617,-64.9981364767374,
0.612583302491977));
#15781=CARTESIAN_POINT('Ctrl Pts',(-202.486197484929,-65.7125427933529,
0.567297187132291));
#15782=CARTESIAN_POINT('Ctrl Pts',(-202.805075366122,-66.4315079379949,
0.522011071772604));
#15783=CARTESIAN_POINT('Ctrl Pts',(-203.342531992607,-66.9003622927727,
0.476724956412918));
#15784=CARTESIAN_POINT('Ctrl Pts',(-203.971174482448,-67.4487633254074,
0.423755516811482));
#15785=CARTESIAN_POINT('Ctrl Pts',(-204.898856465583,-67.6549855987664,
0.370786077210047));
#15786=CARTESIAN_POINT('Ctrl Pts',(-205.700051222351,-67.4230386418016,
0.317816637608611));
#15787=CARTESIAN_POINT('Ctrl Pts',(-206.501245979118,-67.1910916848368,
0.264847198007176));
#15788=CARTESIAN_POINT('Ctrl Pts',(-207.175953509519,-66.5209754975483,
0.21187775840574));
#15789=CARTESIAN_POINT('Ctrl Pts',(-207.415129522268,-65.7234141851915,
0.158908318804305));
#15790=CARTESIAN_POINT('Ctrl Pts',(-207.654305535017,-64.9258528728346,
0.10593887920287));
#15791=CARTESIAN_POINT('Ctrl Pts',(-207.457950030113,-64.0008464354095,
0.0529694396014348));
#15792=CARTESIAN_POINT('Ctrl Pts',(-206.913465996665,-63.364012796625,-2.46594462980148E-16));
#15793=CARTESIAN_POINT('',(-203.082854832445,-63.3612166619665,8.28281533331144E-15));
#15794=CARTESIAN_POINT('Origin',(-205.,-65.,0.));
#15795=CARTESIAN_POINT('Ctrl Pts',(-203.082851793447,-63.3612143523572,
5.48172618408671E-15));
#15796=CARTESIAN_POINT('Ctrl Pts',(-203.614822557714,-62.7406365668551,
0.0519060689144995));
#15797=CARTESIAN_POINT('Ctrl Pts',(-204.477412283426,-62.4011241208618,
0.103812137828994));
#15798=CARTESIAN_POINT('Ctrl Pts',(-205.289478531141,-62.4950491013773,
0.155718206743488));
#15799=CARTESIAN_POINT('Ctrl Pts',(-206.118181127201,-62.5908982705888,
0.208687646344923));
#15800=CARTESIAN_POINT('Ctrl Pts',(-206.894268948213,-63.1381259592108,
0.261657085946359));
#15801=CARTESIAN_POINT('Ctrl Pts',(-207.262498103941,-63.8863946495074,
0.314626525547794));
#15802=CARTESIAN_POINT('Ctrl Pts',(-207.630727259668,-64.634663339804,0.367595965149229));
#15803=CARTESIAN_POINT('Ctrl Pts',(-207.591097750112,-65.5839730317752,
0.420565404750665));
#15804=CARTESIAN_POINT('Ctrl Pts',(-207.161527602495,-66.298919576317,0.473534844352101));
#15805=CARTESIAN_POINT('Ctrl Pts',(-206.731957454879,-67.0138661208588,
0.526504283953536));
#15806=CARTESIAN_POINT('Ctrl Pts',(-205.912446669203,-67.4944495179713,
0.579473723554972));
#15807=CARTESIAN_POINT('Ctrl Pts',(-205.078774820569,-67.520492478951,0.632443163156408));
#15808=CARTESIAN_POINT('Ctrl Pts',(-204.245102971934,-67.5465354399307,
0.685412602757844));
#15809=CARTESIAN_POINT('Ctrl Pts',(-203.39727006034,-67.1180379647775,0.738382042359279));
#15810=CARTESIAN_POINT('Ctrl Pts',(-202.923859465156,-66.4313628808451,
0.791351481960714));
#15811=CARTESIAN_POINT('Ctrl Pts',(-202.637667457015,-66.0162455953229,
0.823373220476479));
#15812=CARTESIAN_POINT('Ctrl Pts',(-202.488311578843,-65.5067748931336,
0.855394958992245));
#15813=CARTESIAN_POINT('Ctrl Pts',(-202.485823045017,-64.9986459985219,
0.88741669750801));
#15814=CARTESIAN_POINT('Origin',(-205.,-65.,-2.20842344717744));
#15815=CARTESIAN_POINT('',(-201.92132715551,-64.9999599234514,16.2084234471775));
#15816=CARTESIAN_POINT('',(-201.931378654624,-64.9992193623962,16.2915765528226));
#15817=CARTESIAN_POINT('',(-201.9265,-64.9999999999997,-2.20842344717744));
#15818=CARTESIAN_POINT('',(-205.793799282533,-67.9692229537457,17.));
#15819=CARTESIAN_POINT('Ctrl Pts',(-201.931378654624,-64.9992193623962,
16.2915765528226));
#15820=CARTESIAN_POINT('Ctrl Pts',(-201.930449249078,-64.5288570727101,
16.315839943476));
#15821=CARTESIAN_POINT('Ctrl Pts',(-202.253363122225,-63.0329492967313,
16.3930727737308));
#15822=CARTESIAN_POINT('Ctrl Pts',(-204.58235400734,-61.3907532347673,16.5232750435871));
#15823=CARTESIAN_POINT('Ctrl Pts',(-207.810233625888,-62.6929017394991,
16.6821833623914));
#15824=CARTESIAN_POINT('Ctrl Pts',(-208.45647866392,-66.1152964431386,16.8410916811957));
#15825=CARTESIAN_POINT('Ctrl Pts',(-206.782006578242,-67.7050332130129,
16.9470305603986));
#15826=CARTESIAN_POINT('Ctrl Pts',(-205.793799282533,-67.9692229537457,
17.));
#15827=CARTESIAN_POINT('',(-204.206200717467,-67.9692229537457,17.));
#15828=CARTESIAN_POINT('Origin',(-205.,-65.,17.));
#15829=CARTESIAN_POINT('Ctrl Pts',(-201.92132715551,-64.9999599234514,16.2084234471775));
#15830=CARTESIAN_POINT('Ctrl Pts',(-201.921326964282,-64.9985177121332,
16.2084984707981));
#15831=CARTESIAN_POINT('Ctrl Pts',(-201.921978795173,-63.9788214197569,
16.2615429340201));
#15832=CARTESIAN_POINT('Ctrl Pts',(-203.036142175806,-61.9425259545107,
16.3675568368436));
#15833=CARTESIAN_POINT('Ctrl Pts',(-206.506723058425,-61.6929032655643,
16.5264651556479));
#15834=CARTESIAN_POINT('Ctrl Pts',(-208.5958014629,-64.4760115385876,16.6853734744522));
#15835=CARTESIAN_POINT('Ctrl Pts',(-207.396688180815,-67.7159880867316,
16.8432184225696));
#15836=CARTESIAN_POINT('Ctrl Pts',(-205.168807240445,-68.2310729455545,
16.9480939310855));
#15837=CARTESIAN_POINT('Ctrl Pts',(-204.204431258832,-67.9745848956374,
17.));
#15838=CARTESIAN_POINT('Origin',(-205.,-65.,-2.20842344717744));
#15839=CARTESIAN_POINT('',(-201.928225509175,-64.9973269163706,15.2084234471775));
#15840=CARTESIAN_POINT('',(-201.926883815323,-65.0028204616814,15.2915765528226));
#15841=CARTESIAN_POINT('',(-201.9265,-64.9999999999997,-2.20842344717744));
#15842=CARTESIAN_POINT('Ctrl Pts',(-201.926883815323,-65.0028204616813,
15.2915765528226));
#15843=CARTESIAN_POINT('Ctrl Pts',(-201.933858564409,-64.2344951248146,
15.3313566392007));
#15844=CARTESIAN_POINT('Ctrl Pts',(-202.61466622664,-62.4320797304894,15.4241061651802));
#15845=CARTESIAN_POINT('Ctrl Pts',(-205.641600447141,-61.4231649792265,
15.5698251307612));
#15846=CARTESIAN_POINT('Ctrl Pts',(-208.354330260832,-63.6021006605898,
15.7287334495655));
#15847=CARTESIAN_POINT('Ctrl Pts',(-207.991779545523,-67.0626823173804,
15.8876417683699));
#15848=CARTESIAN_POINT('Ctrl Pts',(-204.886538848565,-68.6320809475727,
16.0465500871742));
#15849=CARTESIAN_POINT('Ctrl Pts',(-202.343324085074,-67.1406706620033,
16.1811950153251));
#15850=CARTESIAN_POINT('Ctrl Pts',(-201.93247823553,-65.5557055973133,16.2628705038745));
#15851=CARTESIAN_POINT('Ctrl Pts',(-201.931378654624,-64.9992193623962,
16.2915765528226));
#15852=CARTESIAN_POINT('Ctrl Pts',(-201.928225509175,-64.9973269163706,
15.2084234471775));
#15853=CARTESIAN_POINT('Ctrl Pts',(-201.925723596777,-64.6958495188348,
15.2240151665228));
#15854=CARTESIAN_POINT('Ctrl Pts',(-202.105046180913,-63.3730808756464,
15.2925763254695));
#15855=CARTESIAN_POINT('Ctrl Pts',(-204.001159743508,-61.5060359832025,
15.4141069240177));
#15856=CARTESIAN_POINT('Ctrl Pts',(-207.396164971614,-62.2679882236812,
15.5730152428221));
#15857=CARTESIAN_POINT('Ctrl Pts',(-208.594390890487,-65.5346291179969,
15.7319235616264));
#15858=CARTESIAN_POINT('Ctrl Pts',(-206.497323624104,-68.3111057941983,
15.8908318804307));
#15859=CARTESIAN_POINT('Ctrl Pts',(-203.02915628941,-68.0521657341669,16.0496651756144));
#15860=CARTESIAN_POINT('Ctrl Pts',(-201.921461978279,-66.0167720257951,
16.1555290311966));
#15861=CARTESIAN_POINT('Ctrl Pts',(-201.92132715551,-64.9999599234514,16.2084234471775));
#15862=CARTESIAN_POINT('Origin',(-205.,-65.,-2.20842344717744));
#15863=CARTESIAN_POINT('',(-201.930817979872,-65.0014123516849,14.2084234471775));
#15864=CARTESIAN_POINT('',(-201.921592942543,-64.9991754636855,14.2915765528226));
#15865=CARTESIAN_POINT('',(-201.9265,-64.9999999999997,-2.20842344717744));
#15866=CARTESIAN_POINT('Ctrl Pts',(-201.921592942543,-64.9991754636855,
14.2915765528226));
#15867=CARTESIAN_POINT('Ctrl Pts',(-201.92143307583,-64.9544248847186,14.293903895324));
#15868=CARTESIAN_POINT('Ctrl Pts',(-201.942607559848,-63.8913226189859,
14.3492006774268));
#15869=CARTESIAN_POINT('Ctrl Pts',(-203.167704028449,-61.8618209334909,
14.4574668991311));
#15870=CARTESIAN_POINT('Ctrl Pts',(-206.64567409827,-61.7600568166538,14.6163752179354));
#15871=CARTESIAN_POINT('Ctrl Pts',(-208.614908982248,-64.6286359675596,
14.7752835367397));
#15872=CARTESIAN_POINT('Ctrl Pts',(-207.270034820723,-67.8376783991727,
14.934191855544));
#15873=CARTESIAN_POINT('Ctrl Pts',(-203.844019947069,-68.4451671656806,
15.0931001743483));
#15874=CARTESIAN_POINT('Ctrl Pts',(-202.070137442914,-66.5327694250874,
15.2122284067745));
#15875=CARTESIAN_POINT('Ctrl Pts',(-201.924571290698,-65.2575638567064,
15.2783871995992));
#15876=CARTESIAN_POINT('Ctrl Pts',(-201.926883815323,-65.0028204616813,
15.2915765528226));
#15877=CARTESIAN_POINT('Ctrl Pts',(-201.930817979872,-65.0014123516849,
14.2084234471775));
#15878=CARTESIAN_POINT('Ctrl Pts',(-201.933314343602,-64.3986294258202,
14.2395318622475));
#15879=CARTESIAN_POINT('Ctrl Pts',(-202.39654106013,-62.7659248440265,14.323609716919));
#15880=CARTESIAN_POINT('Ctrl Pts',(-205.050996575713,-61.3664239142234,
14.4606570111919));
#15881=CARTESIAN_POINT('Ctrl Pts',(-208.082123040074,-63.0749042303987,
14.6195653299962));
#15882=CARTESIAN_POINT('Ctrl Pts',(-208.287593522688,-66.548290973518,14.7784736488005));
#15883=CARTESIAN_POINT('Ctrl Pts',(-205.479035063749,-68.6022215651833,
14.9373819676048));
#15884=CARTESIAN_POINT('Ctrl Pts',(-202.549962560241,-67.4761806836253,
15.0806985670638));
#15885=CARTESIAN_POINT('Ctrl Pts',(-201.934223294258,-65.7200527158195,
15.1710457269214));
#15886=CARTESIAN_POINT('Ctrl Pts',(-201.928225509175,-64.9973269163706,
15.2084234471775));
#15887=CARTESIAN_POINT('Origin',(-205.,-65.,-2.20842344717744));
#15888=CARTESIAN_POINT('',(-201.923048984138,-65.0020215843026,13.2084234471775));
#15889=CARTESIAN_POINT('',(-201.929343708848,-64.9976509895539,13.2915765528226));
#15890=CARTESIAN_POINT('',(-201.9265,-64.9999999999997,-2.20842344717744));
#15891=CARTESIAN_POINT('Ctrl Pts',(-201.929343708848,-64.9976509895539,
13.2915765528225));
#15892=CARTESIAN_POINT('Ctrl Pts',(-201.926890311751,-64.6523061159044,
13.3094205910487));
#15893=CARTESIAN_POINT('Ctrl Pts',(-202.14012767651,-63.2847573174409,13.3802340688762));
#15894=CARTESIAN_POINT('Ctrl Pts',(-204.150352533451,-61.4667896441583,
13.5040169863052));
#15895=CARTESIAN_POINT('Ctrl Pts',(-207.509958448151,-62.3721520583455,
13.6629253051096));
#15896=CARTESIAN_POINT('Ctrl Pts',(-208.568462516575,-65.6866960888727,
13.8218336239139));
#15897=CARTESIAN_POINT('Ctrl Pts',(-206.355440022032,-68.371684831825,13.9807419427182));
#15898=CARTESIAN_POINT('Ctrl Pts',(-202.950376476172,-67.9714987504005,
14.1373229190211));
#15899=CARTESIAN_POINT('Ctrl Pts',(-201.925071582081,-65.9729312232913,
14.2409344557225));
#15900=CARTESIAN_POINT('Ctrl Pts',(-201.921592942543,-64.9991754636855,
14.2915765528226));
#15901=CARTESIAN_POINT('Ctrl Pts',(-201.923048984138,-65.0020215843026,
13.2084234471775));
#15902=CARTESIAN_POINT('Ctrl Pts',(-201.92987213238,-64.1043840848538,13.2550485579722));
#15903=CARTESIAN_POINT('Ctrl Pts',(-202.817794830182,-62.1752162381125,
13.3546431083684));
#15904=CARTESIAN_POINT('Ctrl Pts',(-206.096501589105,-61.5354422759257,
13.5072070983661));
#15905=CARTESIAN_POINT('Ctrl Pts',(-208.506292006242,-64.0453312989241,
13.6661154171704));
#15906=CARTESIAN_POINT('Ctrl Pts',(-207.701553100804,-67.4304499187966,
13.8250237359747));
#15907=CARTESIAN_POINT('Ctrl Pts',(-204.420060507976,-68.5873592139186,
13.983932054779));
#15908=CARTESIAN_POINT('Ctrl Pts',(-202.208561914266,-66.8727735695644,
14.1117319585133));
#15909=CARTESIAN_POINT('Ctrl Pts',(-201.929063693496,-65.4250100277401,
14.1865624226461));
#15910=CARTESIAN_POINT('Ctrl Pts',(-201.930817979872,-65.0014123516849,
14.2084234471775));
#15911=CARTESIAN_POINT('Origin',(-205.,-65.,-2.20842344717744));
#15912=CARTESIAN_POINT('',(-201.924541298626,-64.9974318278238,12.2084234471775));
#15913=CARTESIAN_POINT('',(-201.930084794051,-65.0019865735648,12.2915765528226));
#15914=CARTESIAN_POINT('',(-201.9265,-64.9999999999997,-2.20842344717744));
#15915=CARTESIAN_POINT('Ctrl Pts',(-201.930084794051,-65.0019865735648,
12.2915765528226));
#15916=CARTESIAN_POINT('Ctrl Pts',(-201.933904603767,-64.3559473602958,
12.3249372867734));
#15917=CARTESIAN_POINT('Ctrl Pts',(-202.449144797282,-62.6785687029257,
12.4112674603257));
#15918=CARTESIAN_POINT('Ctrl Pts',(-205.205168530226,-61.3718624466171,
12.5505670734794));
#15919=CARTESIAN_POINT('Ctrl Pts',(-208.161051598535,-63.2074518072919,
12.7094753922837));
#15920=CARTESIAN_POINT('Ctrl Pts',(-208.218917891802,-66.6864293160267,
12.868383711088));
#15921=CARTESIAN_POINT('Ctrl Pts',(-205.32571623889,-68.6193072768529,13.0272920298923));
#15922=CARTESIAN_POINT('Ctrl Pts',(-202.492314928424,-67.3895978490803,
13.1683563104705));
#15923=CARTESIAN_POINT('Ctrl Pts',(-201.934173140205,-65.6774509959268,
13.2564511514472));
#15924=CARTESIAN_POINT('Ctrl Pts',(-201.929343708848,-64.9976509895539,
13.2915765528225));
#15925=CARTESIAN_POINT('Ctrl Pts',(-201.924541298626,-64.9974318278238,
12.2084234471775));
#15926=CARTESIAN_POINT('Ctrl Pts',(-201.9229576152,-64.8206202024618,12.2175958140955));
#15927=CARTESIAN_POINT('Ctrl Pts',(-202.017351259948,-63.6244303792901,
12.279737620615));
#15928=CARTESIAN_POINT('Ctrl Pts',(-203.586717658077,-61.6521486021326,
12.3948488667359));
#15929=CARTESIAN_POINT('Ctrl Pts',(-207.048871845595,-61.9987335805548,
12.5537571855402));
#15930=CARTESIAN_POINT('Ctrl Pts',(-208.632643224891,-65.0968460677781,
12.7126655043445));
#15931=CARTESIAN_POINT('Ctrl Pts',(-206.886047896905,-68.1061711625154,
12.8715738231488));
#15932=CARTESIAN_POINT('Ctrl Pts',(-203.410344937013,-68.2677932524411,
13.0304821419532));
#15933=CARTESIAN_POINT('Ctrl Pts',(-201.984214425865,-66.265134355684,13.1427653499627));
#15934=CARTESIAN_POINT('Ctrl Pts',(-201.922120551042,-65.1241640810951,
13.2020791183708));
#15935=CARTESIAN_POINT('Ctrl Pts',(-201.923048984138,-65.0020215843026,
13.2084234471775));
#15936=CARTESIAN_POINT('Origin',(-205.,-65.,-2.20842344717744));
#15937=CARTESIAN_POINT('',(-201.931350607177,-64.9994302461114,11.2084234471775));
#15938=CARTESIAN_POINT('',(-201.922104720032,-65.0013994359743,11.2915765528226));
#15939=CARTESIAN_POINT('',(-201.9265,-64.9999999999997,-2.20842344717744));
#15940=CARTESIAN_POINT('Ctrl Pts',(-201.922104720032,-65.0013994359743,
11.2915765528226));
#15941=CARTESIAN_POINT('Ctrl Pts',(-201.927430148624,-64.0611595253334,
11.3404539824981));
#15942=CARTESIAN_POINT('Ctrl Pts',(-202.890890769671,-62.0925255947041,
11.4423008517751));
#15943=CARTESIAN_POINT('Ctrl Pts',(-206.242557904149,-61.585102331427,11.5971171606536));
#15944=CARTESIAN_POINT('Ctrl Pts',(-208.543651054332,-64.1950071819504,
11.7560254794579));
#15945=CARTESIAN_POINT('Ctrl Pts',(-207.59596452456,-67.5429204508222,11.9149337982622));
#15946=CARTESIAN_POINT('Ctrl Pts',(-204.268326733228,-68.5595126720785,
12.0738421170665));
#15947=CARTESIAN_POINT('Ctrl Pts',(-202.169249466841,-66.7844550251247,
12.1993897019199));
#15948=CARTESIAN_POINT('Ctrl Pts',(-201.927839593915,-65.3817142135618,
12.271967847172));
#15949=CARTESIAN_POINT('Ctrl Pts',(-201.930084794051,-65.0019865735648,
12.2915765528226));
#15950=CARTESIAN_POINT('Ctrl Pts',(-201.931350607177,-64.9994302461114,
11.2084234471775));
#15951=CARTESIAN_POINT('Ctrl Pts',(-201.930559226518,-64.5208267214804,
11.2331125098202));
#15952=CARTESIAN_POINT('Ctrl Pts',(-202.261422759148,-63.0164333097365,
11.3107710120644));
#15953=CARTESIAN_POINT('Ctrl Pts',(-204.612026051834,-61.3868362650263,
11.4413989539101));
#15954=CARTESIAN_POINT('Ctrl Pts',(-207.82721483571,-62.7169467301605,11.6003072727144));
#15955=CARTESIAN_POINT('Ctrl Pts',(-208.450444657403,-66.140134915869,11.7592155915187));
#15956=CARTESIAN_POINT('Ctrl Pts',(-205.910345382095,-68.5180601537614,
11.918123910323));
#15957=CARTESIAN_POINT('Ctrl Pts',(-202.730442754502,-67.7195796399602,
12.0678598622093));
#15958=CARTESIAN_POINT('Ctrl Pts',(-201.932103217895,-65.8416884604287,
12.1646263744941));
#15959=CARTESIAN_POINT('Ctrl Pts',(-201.924541298626,-64.9974318278238,
12.2084234471775));
#15960=CARTESIAN_POINT('Origin',(-205.,-65.,-2.20842344717744));
#15961=CARTESIAN_POINT('',(-201.926636231845,-65.0028238856699,10.2084234471775));
#15962=CARTESIAN_POINT('',(-201.925849867817,-64.9972120766658,10.2915765528225));
#15963=CARTESIAN_POINT('',(-201.9265,-64.9999999999997,-2.20842344717744));
#15964=CARTESIAN_POINT('Ctrl Pts',(-201.925849867817,-64.9972120766658,
10.2915765528225));
#15965=CARTESIAN_POINT('Ctrl Pts',(-201.923807687974,-64.7767419557002,
10.3030012386214));
#15966=CARTESIAN_POINT('Ctrl Pts',(-202.04610426792,-63.5363314374797,10.3673953640217));
#15967=CARTESIAN_POINT('Ctrl Pts',(-203.73008217778,-61.5951820963824,10.4847589290234));
#15968=CARTESIAN_POINT('Ctrl Pts',(-207.17440677989,-62.0883971102576,10.6436672478277));
#15969=CARTESIAN_POINT('Ctrl Pts',(-208.625259549091,-65.2509371110651,
10.802575566632));
#15970=CARTESIAN_POINT('Ctrl Pts',(-206.752514882462,-68.1834207731203,
10.9614838854363));
#15971=CARTESIAN_POINT('Ctrl Pts',(-203.273084159089,-68.1973798508147,
11.1203922042406));
#15972=CARTESIAN_POINT('Ctrl Pts',(-201.960112831003,-66.1773468477829,
11.2304230933694));
#15973=CARTESIAN_POINT('Ctrl Pts',(-201.921658876075,-65.0801161580395,
11.2874845428967));
#15974=CARTESIAN_POINT('Ctrl Pts',(-201.922104720032,-65.0013994359743,
11.2915765528226));
#15975=CARTESIAN_POINT('Ctrl Pts',(-201.926636231845,-65.0028238856699,
10.2084234471775));
#15976=CARTESIAN_POINT('Ctrl Pts',(-201.933742916194,-64.2264373124871,
10.248629205545));
#15977=CARTESIAN_POINT('Ctrl Pts',(-202.62647814666,-62.4159028227408,10.3418044035139));
#15978=CARTESIAN_POINT('Ctrl Pts',(-205.670288212686,-61.4284191634349,
10.4879490410842));
#15979=CARTESIAN_POINT('Ctrl Pts',(-208.365419590609,-63.6290780695714,
10.6468573598886));
#15980=CARTESIAN_POINT('Ctrl Pts',(-207.975171902461,-67.0865828790137,
10.8057656786928));
#15981=CARTESIAN_POINT('Ctrl Pts',(-204.857319867018,-68.6311318262819,
10.9646739974972));
#15982=CARTESIAN_POINT('Ctrl Pts',(-202.334362656145,-67.1239410478955,
11.0988932536587));
#15983=CARTESIAN_POINT('Ctrl Pts',(-201.932257103454,-65.5476522781161,
11.1801430702188));
#15984=CARTESIAN_POINT('Ctrl Pts',(-201.931350607177,-64.9994302461114,
11.2084234471775));
#15985=CARTESIAN_POINT('Origin',(-205.,-65.,-2.20842344717744));
#15986=CARTESIAN_POINT('',(-201.921694744017,-64.9990313139748,9.20842344717746));
#15987=CARTESIAN_POINT('',(-201.931440561712,-65.000145803285,9.29157655282255));
#15988=CARTESIAN_POINT('',(-201.9265,-64.9999999999997,-2.20842344717744));
#15989=CARTESIAN_POINT('Ctrl Pts',(-201.931440561712,-65.000145803285,9.29157655282255));
#15990=CARTESIAN_POINT('Ctrl Pts',(-201.931661195711,-64.4778423231913,
9.31851793434612));
#15991=CARTESIAN_POINT('Ctrl Pts',(-202.306392174211,-62.9283411178457,
9.39842875547113));
#15992=CARTESIAN_POINT('Ctrl Pts',(-204.76572719775,-61.3736254349403,9.53130901619758));
#15993=CARTESIAN_POINT('Ctrl Pts',(-207.921565691441,-62.8389978846421,
9.69021733500189));
#15994=CARTESIAN_POINT('Ctrl Pts',(-208.398945412955,-66.2855529206304,
9.8491256538062));
#15995=CARTESIAN_POINT('Ctrl Pts',(-205.760209969182,-68.5535274073437,
10.0080339726105));
#15996=CARTESIAN_POINT('Ctrl Pts',(-202.66434118819,-67.6348334757972,10.155517605616));
#15997=CARTESIAN_POINT('Ctrl Pts',(-201.933276055309,-65.7989301333022,
10.25003179902));
#15998=CARTESIAN_POINT('Ctrl Pts',(-201.925849867817,-64.9972120766658,
10.2915765528225));
#15999=CARTESIAN_POINT('Ctrl Pts',(-201.921694744017,-64.9990313139748,
9.20842344717746));
#16000=CARTESIAN_POINT('Ctrl Pts',(-201.921476386658,-64.9460911648205,
9.21117646166824));
#16001=CARTESIAN_POINT('Ctrl Pts',(-201.946721039892,-63.8747674146739,
9.26689891576045));
#16002=CARTESIAN_POINT('Ctrl Pts',(-203.192942594908,-61.8472203542135,
9.3755908094541));
#16003=CARTESIAN_POINT('Ctrl Pts',(-206.671617371331,-61.7733653252889,
9.5344991282584));
#16004=CARTESIAN_POINT('Ctrl Pts',(-208.61777202504,-64.6576529027109,9.69340744706271));
#16005=CARTESIAN_POINT('Ctrl Pts',(-207.247193721282,-67.8558004725847,
9.85231576586701));
#16006=CARTESIAN_POINT('Ctrl Pts',(-203.816413330272,-68.4357820878843,
10.0112240846713));
#16007=CARTESIAN_POINT('Ctrl Pts',(-202.064218192827,-66.5160946473908,
10.1299266451081));
#16008=CARTESIAN_POINT('Ctrl Pts',(-201.924380150693,-65.2492948176156,
10.1956597659435));
#16009=CARTESIAN_POINT('Ctrl Pts',(-201.926636231845,-65.0028238856699,
10.2084234471775));
#16010=CARTESIAN_POINT('Origin',(-205.,-65.,-2.20842344717744));
#16011=CARTESIAN_POINT('',(-201.929534568487,-64.9977303426259,8.20842344717746));
#16012=CARTESIAN_POINT('',(-201.925313510444,-65.0027227882489,8.29157655282255));
#16013=CARTESIAN_POINT('',(-201.9265,-64.9999999999997,-2.20842344717744));
#16014=CARTESIAN_POINT('Ctrl Pts',(-201.925313510444,-65.0027227882489,
8.29157655282255));
#16015=CARTESIAN_POINT('Ctrl Pts',(-201.932861178308,-64.1837468504499,
8.33403463007084));
#16016=CARTESIAN_POINT('Ctrl Pts',(-202.690778756775,-62.3307071827764,
8.42946214692057));
#16017=CARTESIAN_POINT('Ctrl Pts',(-205.821270902666,-61.4600861117225,
8.57785910337174));
#16018=CARTESIAN_POINT('Ctrl Pts',(-208.420572386066,-63.7731500565804,
8.73676742217605));
#16019=CARTESIAN_POINT('Ctrl Pts',(-207.883931336951,-67.2109763173173,
8.89567574098036));
#16020=CARTESIAN_POINT('Ctrl Pts',(-204.703334271224,-68.6218042019629,
9.05458405978466));
#16021=CARTESIAN_POINT('Ctrl Pts',(-202.287845189519,-67.0359571342454,
9.18655099706539));
#16022=CARTESIAN_POINT('Ctrl Pts',(-201.931227407294,-65.504742989671,9.26554849474469));
#16023=CARTESIAN_POINT('Ctrl Pts',(-201.931440561712,-65.000145803285,9.29157655282255));
#16024=CARTESIAN_POINT('Ctrl Pts',(-201.929534568487,-64.9977303426259,
8.20842344717746));
#16025=CARTESIAN_POINT('Ctrl Pts',(-201.92711734297,-64.6440919294598,8.22669315739296));
#16026=CARTESIAN_POINT('Ctrl Pts',(-202.147019439276,-63.2680620239934,
8.29793230720989));
#16027=CARTESIAN_POINT('Ctrl Pts',(-204.178729105786,-61.4600861481526,
8.42214089662826));
#16028=CARTESIAN_POINT('Ctrl Pts',(-207.530962539076,-62.3923756815873,
8.58104921543256));
#16029=CARTESIAN_POINT('Ctrl Pts',(-208.562837804587,-65.7153060452649,
8.73995753423686));
#16030=CARTESIAN_POINT('Ctrl Pts',(-206.328343191953,-68.3824518214713,
8.89886585304117));
#16031=CARTESIAN_POINT('Ctrl Pts',(-202.935848001202,-67.9561197966926,
9.0550211573547));
#16032=CARTESIAN_POINT('Ctrl Pts',(-201.925677696523,-65.9646873409452,
9.1582070220668));
#16033=CARTESIAN_POINT('Ctrl Pts',(-201.921694744017,-64.9990313139748,
9.20842344717746));
#16034=CARTESIAN_POINT('Origin',(-205.,-65.,-2.20842344717744));
#16035=CARTESIAN_POINT('',(-201.929918496038,-65.0020818238314,7.20842344717746));
#16036=CARTESIAN_POINT('',(-201.922453576025,-64.9983309056558,7.29157655282255));
#16037=CARTESIAN_POINT('',(-201.9265,-64.9999999999997,-2.20842344717744));
#16038=CARTESIAN_POINT('Ctrl Pts',(-201.922453576025,-64.9983309056558,
7.29157655282255));
#16039=CARTESIAN_POINT('Ctrl Pts',(-201.921823116646,-64.9020160304314,
7.29658188619413));
#16040=CARTESIAN_POINT('Ctrl Pts',(-201.969645702973,-63.7870736983909,
7.35455665916714));
#16041=CARTESIAN_POINT('Ctrl Pts',(-203.328382611466,-61.7733652920829,
7.4655008717416));
#16042=CARTESIAN_POINT('Ctrl Pts',(-206.807057423689,-61.8472203217673,
7.6244091905459));
#16043=CARTESIAN_POINT('Ctrl Pts',(-208.629042186982,-64.811508522489,7.78331750935021));
#16044=CARTESIAN_POINT('Ctrl Pts',(-207.123961634304,-67.9486036030623,
7.94222582815452));
#16045=CARTESIAN_POINT('Ctrl Pts',(-203.671656794376,-68.3824518562811,
8.10113414695882));
#16046=CARTESIAN_POINT('Ctrl Pts',(-202.034187830935,-66.4279300575628,
8.21758438851483));
#16047=CARTESIAN_POINT('Ctrl Pts',(-201.923444931436,-65.2054769730502,
8.28106519046941));
#16048=CARTESIAN_POINT('Ctrl Pts',(-201.925313510444,-65.0027227882489,
8.29157655282255));
#16049=CARTESIAN_POINT('Ctrl Pts',(-201.929918496038,-65.0020818238314,
7.20842344717746));
#16050=CARTESIAN_POINT('Ctrl Pts',(-201.933986215544,-64.3478883205901,
7.24220985311768));
#16051=CARTESIAN_POINT('Ctrl Pts',(-202.459399639161,-62.6621016376928,
7.32896569865933));
#16052=CARTESIAN_POINT('Ctrl Pts',(-205.234272799839,-61.3736254722602,
7.46869098380241));
#16053=CARTESIAN_POINT('Ctrl Pts',(-208.175332576579,-63.2328726734323,
7.62759930260673));
#16054=CARTESIAN_POINT('Ctrl Pts',(-208.205282937147,-66.7122024567848,
7.78650762141103));
#16055=CARTESIAN_POINT('Ctrl Pts',(-205.296665725724,-68.62180416469,7.94541594021533));
#16056=CARTESIAN_POINT('Ctrl Pts',(-202.481742349981,-67.3731793594825,
8.08605454880414));
#16057=CARTESIAN_POINT('Ctrl Pts',(-201.93412561401,-65.6693971119722,8.17372371779152));
#16058=CARTESIAN_POINT('Ctrl Pts',(-201.929534568487,-64.9977303426259,
8.20842344717746));
#16059=CARTESIAN_POINT('Origin',(-205.,-65.,-2.20842344717744));
#16060=CARTESIAN_POINT('',(-201.92196047901,-65.0012666663909,6.20842344717746));
#16061=CARTESIAN_POINT('',(-201.93041282103,-64.9982329274285,6.29157655282255));
#16062=CARTESIAN_POINT('',(-201.9265,-64.9999999999997,-2.20842344717744));
#16063=CARTESIAN_POINT('Ctrl Pts',(-201.93041282103,-64.9982329274285,6.29157655282255));
#16064=CARTESIAN_POINT('Ctrl Pts',(-201.928336237733,-64.6007120797469,
6.31209858191885));
#16065=CARTESIAN_POINT('Ctrl Pts',(-202.184897914724,-63.1797266043789,
6.38559005061658));
#16066=CARTESIAN_POINT('Ctrl Pts',(-204.329711780416,-61.428419126679,6.51205095891576));
#16067=CARTESIAN_POINT('Ctrl Pts',(-207.639355934117,-62.5021456237346,
6.67095927772006));
#16068=CARTESIAN_POINT('Ctrl Pts',(-208.529268066955,-65.8658770949486,
6.82986759652438));
#16069=CARTESIAN_POINT('Ctrl Pts',(-206.183586681908,-68.4357821232429,
6.98877591532867));
#16070=CARTESIAN_POINT('Ctrl Pts',(-202.860869822607,-67.8740689059555,
7.14267890076141));
#16071=CARTESIAN_POINT('Ctrl Pts',(-201.928495015897,-65.9212778032609,
7.24361244659269));
#16072=CARTESIAN_POINT('Ctrl Pts',(-201.922453576025,-64.9983309056558,
7.29157655282255));
#16073=CARTESIAN_POINT('Ctrl Pts',(-201.92196047901,-65.0012666663909,6.20842344717746));
#16074=CARTESIAN_POINT('Ctrl Pts',(-201.926898060984,-64.052956064959,6.25772654884239));
#16075=CARTESIAN_POINT('Ctrl Pts',(-202.905060811709,-62.0770176673835,
6.35999909010877));
#16076=CARTESIAN_POINT('Ctrl Pts',(-206.26991780915,-61.5951821314221,6.51524107097657));
#16077=CARTESIAN_POINT('Ctrl Pts',(-208.549995921993,-64.2234660895895,
6.67414938978088));
#16078=CARTESIAN_POINT('Ctrl Pts',(-207.575477451123,-67.5636676576622,
6.83305770858519));
#16079=CARTESIAN_POINT('Ctrl Pts',(-204.239790038642,-68.5535273707736,
6.9919660273895));
#16080=CARTESIAN_POINT('Ctrl Pts',(-202.162091241287,-66.7677599212191,
7.11708794025358));
#16081=CARTESIAN_POINT('Ctrl Pts',(-201.927608951769,-65.3735157080934,
7.18924041351624));
#16082=CARTESIAN_POINT('Ctrl Pts',(-201.929918496038,-65.0020818238314,
7.20842344717746));
#16083=CARTESIAN_POINT('Origin',(-205.,-65.,-2.20842344717744));
#16084=CARTESIAN_POINT('',(-201.926100533607,-64.9971929803835,5.20842344717745));
#16085=CARTESIAN_POINT('',(-201.928910873452,-65.0025004618091,5.29157655282255));
#16086=CARTESIAN_POINT('',(-201.9265,-64.9999999999997,-2.20842344717744));
#16087=CARTESIAN_POINT('Ctrl Pts',(-201.928910873452,-65.0025004618091,
5.29157655282255));
#16088=CARTESIAN_POINT('Ctrl Pts',(-201.934235624731,-64.3052721134968,
5.32761527764357));
#16089=CARTESIAN_POINT('Ctrl Pts',(-202.515343946683,-62.5752315257807,
5.41662344206602));
#16090=CARTESIAN_POINT('Ctrl Pts',(-205.387973952159,-61.3868362278423,
5.55860104608991));
#16091=CARTESIAN_POINT('Ctrl Pts',(-208.247472586089,-63.3692339117493,
5.71750936489423));
#16092=CARTESIAN_POINT('Ctrl Pts',(-208.129724649422,-66.8466997186291,
5.87641768369853));
#16093=CARTESIAN_POINT('Ctrl Pts',(-205.142680134451,-68.6311318636507,
6.03532600250283));
#16094=CARTESIAN_POINT('Ctrl Pts',(-202.427479427965,-67.286051871031,6.17371229221084));
#16095=CARTESIAN_POINT('Ctrl Pts',(-201.933696109946,-65.6267537266412,
6.25912914231741));
#16096=CARTESIAN_POINT('Ctrl Pts',(-201.93041282103,-64.9982329274285,6.29157655282255));
#16097=CARTESIAN_POINT('Ctrl Pts',(-201.926100533607,-64.9971929803835,
5.20842344717745));
#16098=CARTESIAN_POINT('Ctrl Pts',(-201.923984660047,-64.7684605820622,
5.22027380496568));
#16099=CARTESIAN_POINT('Ctrl Pts',(-202.051779336195,-63.5196687889702,
5.28509360235533));
#16100=CARTESIAN_POINT('Ctrl Pts',(-203.757442108639,-61.5851023665706,
5.40288283934643));
#16101=CARTESIAN_POINT('Ctrl Pts',(-207.197698422129,-62.1059375256302,
5.56179115815073));
#16102=CARTESIAN_POINT('Ctrl Pts',(-208.623129385432,-65.2800168148538,
5.72069947695504));
#16103=CARTESIAN_POINT('Ctrl Pts',(-206.726915823139,-68.1973798179096,
5.87960779575935));
#16104=CARTESIAN_POINT('Ctrl Pts',(-203.247485135573,-68.183420740359,6.03851611456365));
#16105=CARTESIAN_POINT('Ctrl Pts',(-201.955780678157,-66.1607732940332,
6.14812133170302));
#16106=CARTESIAN_POINT('Ctrl Pts',(-201.921593304462,-65.0717861066736,
6.20475710924096));
#16107=CARTESIAN_POINT('Ctrl Pts',(-201.92196047901,-65.0012666663909,6.20842344717746));
#16108=CARTESIAN_POINT('Origin',(-205.,-65.,-2.20842344717744));
#16109=CARTESIAN_POINT('',(-201.931423553656,-65.0002813807169,4.20842344717746));
#16110=CARTESIAN_POINT('',(-201.921426613004,-65.0005065231376,4.29157655282254));
#16111=CARTESIAN_POINT('',(-201.9265,-64.9999999999997,-2.20842344717744));
#16112=CARTESIAN_POINT('Ctrl Pts',(-201.921426613004,-65.0005065231376,
4.29157655282254));
#16113=CARTESIAN_POINT('Ctrl Pts',(-201.923689481612,-64.0093326254348,
4.34313197336828));
#16114=CARTESIAN_POINT('Ctrl Pts',(-202.981935532719,-61.9956495212633,
4.44765683351546));
#16115=CARTESIAN_POINT('Ctrl Pts',(-206.413282356468,-61.652148567679,4.60515113326408));
#16116=CARTESIAN_POINT('Ctrl Pts',(-208.579755111172,-64.3748363606043,
4.76405945206838));
#16117=CARTESIAN_POINT('Ctrl Pts',(-207.464348390136,-67.6706671908,4.92296777087269));
#16118=CARTESIAN_POINT('Ctrl Pts',(-204.089654608536,-68.5180601899667,
5.08187608967699));
#16119=CARTESIAN_POINT('Ctrl Pts',(-202.125622944275,-66.6794232091735,
5.20474568366028));
#16120=CARTESIAN_POINT('Ctrl Pts',(-201.926409346397,-65.3300529587612,
5.27464583804213));
#16121=CARTESIAN_POINT('Ctrl Pts',(-201.928910873452,-65.0025004618091,
5.29157655282255));
#16122=CARTESIAN_POINT('Ctrl Pts',(-201.931423553656,-65.0002813807169,
4.20842344717746));
#16123=CARTESIAN_POINT('Ctrl Pts',(-201.931856208338,-64.4697328931174,
4.2357905006904));
#16124=CARTESIAN_POINT('Ctrl Pts',(-202.315183154355,-62.9117123239822,
4.31612699380478));
#16125=CARTESIAN_POINT('Ctrl Pts',(-204.794831471885,-61.3718624839552,
4.44943292652058));
#16126=CARTESIAN_POINT('Ctrl Pts',(-207.93881072326,-62.8625090659739,4.6083412453249));
#16127=CARTESIAN_POINT('Ctrl Pts',(-208.388521150012,-66.3127834459959,
4.7672495641292));
#16128=CARTESIAN_POINT('Ctrl Pts',(-205.731673259242,-68.5595126354467,
4.92615788293351));
#16129=CARTESIAN_POINT('Ctrl Pts',(-202.652189269735,-67.6187313168277,
5.07321584394959));
#16130=CARTESIAN_POINT('Ctrl Pts',(-201.93344231852,-65.7908623672484,5.16730436536424));
#16131=CARTESIAN_POINT('Ctrl Pts',(-201.926100533607,-64.9971929803835,
5.20842344717745));
#16132=CARTESIAN_POINT('Origin',(-205.,-65.,-2.20842344717744));
#16133=CARTESIAN_POINT('',(-201.925065525565,-65.0026812057629,3.20842344717745));
#16134=CARTESIAN_POINT('',(-201.927406805321,-64.9972100888671,3.29157655282254));
#16135=CARTESIAN_POINT('',(-201.9265,-64.9999999999997,-2.20842344717744));
#16136=CARTESIAN_POINT('Ctrl Pts',(-201.927406805321,-64.9972100888671,
3.29157655282254));
#16137=CARTESIAN_POINT('Ctrl Pts',(-201.924995747753,-64.724708687099,3.30567922949157));
#16138=CARTESIAN_POINT('Ctrl Pts',(-202.083109157865,-63.4314473629371,
3.37275134576203));
#16139=CARTESIAN_POINT('Ctrl Pts',(-203.90349839961,-61.5354422402711,3.49279290163393));
#16140=CARTESIAN_POINT('Ctrl Pts',(-207.318549253241,-62.2018210220118,
3.65170122043824));
#16141=CARTESIAN_POINT('Ctrl Pts',(-208.607980065528,-65.4335390165435,
3.81060953924254));
#16142=CARTESIAN_POINT('Ctrl Pts',(-206.589655079347,-68.2677932860708,
3.96951785804685));
#16143=CARTESIAN_POINT('Ctrl Pts',(-203.113952083686,-68.1061711944818,
4.12842617685116));
#16144=CARTESIAN_POINT('Ctrl Pts',(-201.934013400269,-66.0731764684801,
4.23577907510972));
#16145=CARTESIAN_POINT('Ctrl Pts',(-201.921364548932,-65.0276916137454,
4.29016253376685));
#16146=CARTESIAN_POINT('Ctrl Pts',(-201.921426613004,-65.0005065231376,
4.29157655282254));
#16147=CARTESIAN_POINT('Ctrl Pts',(-201.925065525565,-65.0026812057629,
3.20842344717745));
#16148=CARTESIAN_POINT('Ctrl Pts',(-201.932639942483,-64.1756663036064,
3.25130719641512));
#16149=CARTESIAN_POINT('Ctrl Pts',(-202.703271098363,-62.3146899905717,
3.34716038525422));
#16150=CARTESIAN_POINT('Ctrl Pts',(-205.849647457805,-61.4667896805192,
3.49598301369474));
#16151=CARTESIAN_POINT('Ctrl Pts',(-208.430306047719,-63.8006350093353,
3.65489133249905));
#16152=CARTESIAN_POINT('Ctrl Pts',(-207.86609839156,-67.2340447552034,3.81379965130336));
#16153=CARTESIAN_POINT('Ctrl Pts',(-204.674283764462,-68.6193072396057,
3.97270797010767));
#16154=CARTESIAN_POINT('Ctrl Pts',(-202.27934682778,-67.0193078694193,4.10424923539903));
#16155=CARTESIAN_POINT('Ctrl Pts',(-201.931018797178,-65.4966193299875,
4.18282106108896));
#16156=CARTESIAN_POINT('Ctrl Pts',(-201.931423553656,-65.0002813807169,
4.20842344717746));
#16157=CARTESIAN_POINT('Origin',(-205.,-65.,-2.20842344717744));
#16158=CARTESIAN_POINT('',(-201.922632855754,-64.9982129720012,2.20842344717745));
#16159=CARTESIAN_POINT('',(-201.931155097516,-65.0009810679335,2.29157655282254));
#16160=CARTESIAN_POINT('',(-201.9265,-64.9999999999997,-2.20842344717744));
#16161=CARTESIAN_POINT('Ctrl Pts',(-201.931155097516,-65.0009810679335,
2.29157655282254));
#16162=CARTESIAN_POINT('Ctrl Pts',(-201.932795742513,-64.4268935344444,
2.32119592521629));
#16163=CARTESIAN_POINT('Ctrl Pts',(-202.363272159361,-62.8238592626871,
2.40378473721147));
#16164=CARTESIAN_POINT('Ctrl Pts',(-204.949003423762,-61.3664238768246,
2.53934298880808));
#16165=CARTESIAN_POINT('Ctrl Pts',(-208.026882997387,-62.9891654522027,
2.69825130761239));
#16166=CARTESIAN_POINT('Ctrl Pts',(-208.329750076191,-66.455417699762,2.8571596264167));
#16167=CARTESIAN_POINT('Ctrl Pts',(-205.579939497992,-68.5873592508376,
3.01606794522101));
#16168=CARTESIAN_POINT('Ctrl Pts',(-202.589670325603,-67.5331224660227,
3.16087358735629));
#16169=CARTESIAN_POINT('Ctrl Pts',(-201.9340516434,-65.7482198177174,3.25270978989013));
#16170=CARTESIAN_POINT('Ctrl Pts',(-201.927406805321,-64.9972100888671,
3.29157655282254));
#16171=CARTESIAN_POINT('Ctrl Pts',(-201.922632855754,-64.9982129720012,
2.20842344717745));
#16172=CARTESIAN_POINT('Ctrl Pts',(-201.921910441958,-64.8936910841268,
2.2138544525384));
#16173=CARTESIAN_POINT('Ctrl Pts',(-201.974200188913,-63.7704822827847,
2.27225489750078));
#16174=CARTESIAN_POINT('Ctrl Pts',(-203.354325918685,-61.7600568500266,
2.3836247820646));
#16175=CARTESIAN_POINT('Ctrl Pts',(-206.832295952684,-61.8618209657714,
2.54253310086891));
#16176=CARTESIAN_POINT('Ctrl Pts',(-208.630437747347,-64.8406327545204,
2.70144141967322));
#16177=CARTESIAN_POINT('Ctrl Pts',(-207.100234689454,-67.965550551091,2.86034973847752));
#16178=CARTESIAN_POINT('Ctrl Pts',(-203.644559991919,-68.3716847971282,
3.01925805728183));
#16179=CARTESIAN_POINT('Ctrl Pts',(-202.028754213716,-66.4112798143637,
3.13528262684847));
#16180=CARTESIAN_POINT('Ctrl Pts',(-201.923284122934,-65.1971841673195,
3.19833775681368));
#16181=CARTESIAN_POINT('Ctrl Pts',(-201.925065525565,-65.0026812057629,
3.20842344717745));
#16182=CARTESIAN_POINT('Origin',(-205.,-65.,-2.20842344717744));
#16183=CARTESIAN_POINT('',(-201.930556952874,-64.9983469618497,1.20842344717745));
#16184=CARTESIAN_POINT('',(-201.92380386931,-65.0023470817023,1.29157655282254));
#16185=CARTESIAN_POINT('',(-201.9265,-64.9999999999997,-2.20842344717744));
#16186=CARTESIAN_POINT('Ctrl Pts',(-201.92380386931,-65.0023470817023,1.29157655282254));
#16187=CARTESIAN_POINT('Ctrl Pts',(-201.931157820393,-64.1328208103926,
1.33671262094101));
#16188=CARTESIAN_POINT('Ctrl Pts',(-202.771191487033,-62.2304278274959,
1.43481812866091));
#16189=CARTESIAN_POINT('Ctrl Pts',(-205.998840266797,-61.5060359469962,
1.58589307598225));
#16190=CARTESIAN_POINT('Ctrl Pts',(-208.478118943853,-63.9473056488985,
1.74480139478655));
#16191=CARTESIAN_POINT('Ctrl Pts',(-207.768697529891,-67.3536763121769,
1.90370971359086));
#16192=CARTESIAN_POINT('Ctrl Pts',(-204.52096493132,-68.6022216022895,2.06261803239517));
#16193=CARTESIAN_POINT('Ctrl Pts',(-202.235901628419,-66.931128943739,2.19190697880573));
#16194=CARTESIAN_POINT('Ctrl Pts',(-201.929861715252,-65.453555900103,2.26822648561485));
#16195=CARTESIAN_POINT('Ctrl Pts',(-201.931155097516,-65.0009810679335,
2.29157655282254));
#16196=CARTESIAN_POINT('Ctrl Pts',(-201.930556952874,-64.9983469618497,
1.20842344717745));
#16197=CARTESIAN_POINT('Ctrl Pts',(-201.928569491267,-64.5925310316569,
1.22937114826312));
#16198=CARTESIAN_POINT('Ctrl Pts',(-202.192314055039,-63.1630216590503,
1.30328828895022));
#16199=CARTESIAN_POINT('Ctrl Pts',(-204.358399560164,-61.4231650176065,
1.43017486923876));
#16200=CARTESIAN_POINT('Ctrl Pts',(-207.659308409489,-62.5233989116837,
1.58908318804307));
#16201=CARTESIAN_POINT('Ctrl Pts',(-208.522209085787,-65.8941689287448,
1.74799150684737));
#16202=CARTESIAN_POINT('Ctrl Pts',(-206.155980040914,-68.445167130006,1.90689982565168));
#16203=CARTESIAN_POINT('Ctrl Pts',(-202.847056020182,-67.8584404971801,
2.06037713909504));
#16204=CARTESIAN_POINT('Ctrl Pts',(-201.928956256023,-65.9131093057697,
2.16088501293696));
#16205=CARTESIAN_POINT('Ctrl Pts',(-201.922632855754,-64.9982129720012,
2.20842344717745));
#16206=CARTESIAN_POINT('Origin',(-205.,-65.,-2.20842344717744));
#16207=CARTESIAN_POINT('',(-201.92961158086,-65.0031570762977,0.208423447177454));
#16208=CARTESIAN_POINT('',(-201.923731533573,-64.9977249101301,0.291576552822544));
#16209=CARTESIAN_POINT('',(-201.9265,-64.9999999999997,-2.20842344717744));
#16210=CARTESIAN_POINT('',(-204.206200717467,-67.9692229537457,0.));
#16211=CARTESIAN_POINT('Ctrl Pts',(-204.206200717467,-67.9692229537457,
-8.32667268468867E-16));
#16212=CARTESIAN_POINT('Ctrl Pts',(-203.217993421758,-67.705033213013,0.0529694396014348));
#16213=CARTESIAN_POINT('Ctrl Pts',(-202.119878302883,-66.6624875897336,
0.12244392199392));
#16214=CARTESIAN_POINT('Ctrl Pts',(-201.92719206015,-65.3223930798511,0.191918404386405));
#16215=CARTESIAN_POINT('Ctrl Pts',(-201.92961158086,-65.0031570762977,0.208423447177454));
#16216=CARTESIAN_POINT('',(-205.795567289133,-67.9745804941197,-1.17835206387761E-15));
#16217=CARTESIAN_POINT('Origin',(-205.,-65.,0.));
#16218=CARTESIAN_POINT('Ctrl Pts',(-205.795568749511,-67.9745849194644,
-1.60597446799415E-16));
#16219=CARTESIAN_POINT('Ctrl Pts',(-204.83119279379,-68.2310729434654,0.0519060689144953));
#16220=CARTESIAN_POINT('Ctrl Pts',(-202.766529390716,-67.7537239905742,
0.149098253188677));
#16221=CARTESIAN_POINT('Ctrl Pts',(-201.931014089346,-65.8699107350031,
0.246290437462858));
#16222=CARTESIAN_POINT('Ctrl Pts',(-201.923731533573,-64.9977249101301,
0.291576552822544));
#16223=CARTESIAN_POINT('Origin',(-205.,-65.,17.));
#16224=CARTESIAN_POINT('Ctrl Pts',(-203.086534003335,-63.3640127966251,
17.));
#16225=CARTESIAN_POINT('Ctrl Pts',(-203.02440597855,-63.4223978842397,17.));
#16226=CARTESIAN_POINT('Ctrl Pts',(-202.965656533056,-63.484037682377,17.));
#16227=CARTESIAN_POINT('Ctrl Pts',(-202.910296296302,-63.5485554899634,
17.));
#16228=CARTESIAN_POINT('Ctrl Pts',(-202.853579007623,-63.6146548300752,
17.));
#16229=CARTESIAN_POINT('Ctrl Pts',(-202.800418658262,-63.6837754979915,
17.));
#16230=CARTESIAN_POINT('Ctrl Pts',(-202.750855616275,-63.7555586853473,
17.));
#16231=CARTESIAN_POINT('Ctrl Pts',(-202.737942375479,-63.7742612013012,
17.));
#16232=CARTESIAN_POINT('Ctrl Pts',(-202.725273497568,-63.7931446704172,
17.));
#16233=CARTESIAN_POINT('Ctrl Pts',(-202.712850070252,-63.8122031777925,
17.));
#16234=CARTESIAN_POINT('Ctrl Pts',(-202.702648305927,-63.8278534807001,
17.));
#16235=CARTESIAN_POINT('Ctrl Pts',(-202.692611588147,-63.8436227659743,
17.));
#16236=CARTESIAN_POINT('Ctrl Pts',(-202.682749443169,-63.859493035454,17.));
#16237=CARTESIAN_POINT('Ctrl Pts',(-202.63531796322,-63.9358202817403,17.));
#16238=CARTESIAN_POINT('Ctrl Pts',(-202.59187124907,-64.0145559081911,17.));
#16239=CARTESIAN_POINT('Ctrl Pts',(-202.552442526139,-64.0953069128711,
17.));
#16240=CARTESIAN_POINT('Ctrl Pts',(-202.520315679276,-64.1611034938538,
17.));
#16241=CARTESIAN_POINT('Ctrl Pts',(-202.490856911205,-64.2282391982212,
17.));
#16242=CARTESIAN_POINT('Ctrl Pts',(-202.464101958719,-64.2965198329108,
17.));
#16243=CARTESIAN_POINT('Ctrl Pts',(-202.455216196125,-64.3191969619356,
17.));
#16244=CARTESIAN_POINT('Ctrl Pts',(-202.446628808742,-64.3420004925349,
17.));
#16245=CARTESIAN_POINT('Ctrl Pts',(-202.43834153865,-64.3649236233451,17.));
#16246=CARTESIAN_POINT('Ctrl Pts',(-202.431659599736,-64.3834063031797,
17.));
#16247=CARTESIAN_POINT('Ctrl Pts',(-202.425171976069,-64.4019694556671,
17.));
#16248=CARTESIAN_POINT('Ctrl Pts',(-202.418887257457,-64.4205860790577,
17.));
#16249=CARTESIAN_POINT('Ctrl Pts',(-202.389370048133,-64.5080220970403,
17.));
#16250=CARTESIAN_POINT('Ctrl Pts',(-202.364286527296,-64.5967387245119,
17.));
#16251=CARTESIAN_POINT('Ctrl Pts',(-202.343667851554,-64.6863376891691,
17.));
#16252=CARTESIAN_POINT('Ctrl Pts',(-202.322591412091,-64.7779258773834,
17.));
#16253=CARTESIAN_POINT('Ctrl Pts',(-202.306179715118,-64.8704368052643,
17.));
#16254=CARTESIAN_POINT('Ctrl Pts',(-202.294508870619,-64.9634790031726,
17.));
#16255=CARTESIAN_POINT('Ctrl Pts',(-202.283005247673,-65.0551880789642,
17.));
#16256=CARTESIAN_POINT('Ctrl Pts',(-202.276107302816,-65.1474142708408,
17.));
#16257=CARTESIAN_POINT('Ctrl Pts',(-202.273935013967,-65.2398018803324,
17.));
#16258=CARTESIAN_POINT('Ctrl Pts',(-202.272809982513,-65.2876495533737,
17.));
#16259=CARTESIAN_POINT('Ctrl Pts',(-202.272953276915,-65.3355407504061,
17.));
#16260=CARTESIAN_POINT('Ctrl Pts',(-202.27438704446,-65.383426836211,17.));
#16261=CARTESIAN_POINT('Ctrl Pts',(-202.275036744558,-65.4051260264126,
17.));
#16262=CARTESIAN_POINT('Ctrl Pts',(-202.275952004537,-65.4268312379048,
17.));
#16263=CARTESIAN_POINT('Ctrl Pts',(-202.277132662655,-65.4484998374491,
17.));
#16264=CARTESIAN_POINT('Ctrl Pts',(-202.282342582934,-65.5441174209293,
17.));
#16265=CARTESIAN_POINT('Ctrl Pts',(-202.292716438461,-65.6391274226978,
17.));
#16266=CARTESIAN_POINT('Ctrl Pts',(-202.308321259936,-65.7331327397659,
17.));
#16267=CARTESIAN_POINT('Ctrl Pts',(-202.312170275657,-65.7563196723322,
17.));
#16268=CARTESIAN_POINT('Ctrl Pts',(-202.316337767864,-65.7794455742674,
17.));
#16269=CARTESIAN_POINT('Ctrl Pts',(-202.320825205417,-65.8025046417956,
17.));
#16270=CARTESIAN_POINT('Ctrl Pts',(-202.338330039074,-65.8924546715381,
17.));
#16271=CARTESIAN_POINT('Ctrl Pts',(-202.360699143547,-65.981387621661,17.));
#16272=CARTESIAN_POINT('Ctrl Pts',(-202.387629324862,-66.0690734250235,
17.));
#16273=CARTESIAN_POINT('Ctrl Pts',(-202.415161796534,-66.1587203111241,
17.));
#16274=CARTESIAN_POINT('Ctrl Pts',(-202.447461860745,-66.2470643438459,
17.));
#16275=CARTESIAN_POINT('Ctrl Pts',(-202.484259699373,-66.3338552345522,
17.));
#16276=CARTESIAN_POINT('Ctrl Pts',(-202.498888789869,-66.3683592120058,
17.));
#16277=CARTESIAN_POINT('Ctrl Pts',(-202.514229318749,-66.4026176104445,
17.));
#16278=CARTESIAN_POINT('Ctrl Pts',(-202.53026650595,-66.4366141224841,17.));
#16279=CARTESIAN_POINT('Ctrl Pts',(-202.538263030882,-66.4535655961273,
17.));
#16280=CARTESIAN_POINT('Ctrl Pts',(-202.546434613239,-66.4704554166591,
17.));
#16281=CARTESIAN_POINT('Ctrl Pts',(-202.554767107621,-66.4872571600793,
17.));
#16282=CARTESIAN_POINT('Ctrl Pts',(-202.597562057197,-66.5735494189751,
17.));
#16283=CARTESIAN_POINT('Ctrl Pts',(-202.644652245067,-66.6576403398475,
17.));
#16284=CARTESIAN_POINT('Ctrl Pts',(-202.695692225863,-66.7392833372882,
17.));
#16285=CARTESIAN_POINT('Ctrl Pts',(-202.747749531408,-66.8225536363186,
17.));
#16286=CARTESIAN_POINT('Ctrl Pts',(-202.803915970958,-66.9032782223774,
17.));
#16287=CARTESIAN_POINT('Ctrl Pts',(-202.863880125944,-66.9811882726074,
17.));
#16288=CARTESIAN_POINT('Ctrl Pts',(-202.924342162766,-67.0597452092798,
17.));
#16289=CARTESIAN_POINT('Ctrl Pts',(-202.988665705321,-67.1354415100437,
17.));
#16290=CARTESIAN_POINT('Ctrl Pts',(-203.056580879016,-67.2079822210047,
17.));
#16291=CARTESIAN_POINT('Ctrl Pts',(-203.094627114409,-67.2486196929359,
17.));
#16292=CARTESIAN_POINT('Ctrl Pts',(-203.13380134389,-67.2882664402971,17.));
#16293=CARTESIAN_POINT('Ctrl Pts',(-203.17406195576,-67.326866466561,17.));
#16294=CARTESIAN_POINT('Ctrl Pts',(-203.185603488747,-67.3379319585079,
17.));
#16295=CARTESIAN_POINT('Ctrl Pts',(-203.197234324745,-67.3489114087184,
17.));
#16296=CARTESIAN_POINT('Ctrl Pts',(-203.208953539895,-67.3598034420083,
17.));
#16297=CARTESIAN_POINT('Ctrl Pts',(-203.219358840357,-67.3694743011535,
17.));
#16298=CARTESIAN_POINT('Ctrl Pts',(-203.229830604016,-67.3790732118472,
17.));
#16299=CARTESIAN_POINT('Ctrl Pts',(-203.240361997973,-67.3885939838815,
17.));
#16300=CARTESIAN_POINT('Ctrl Pts',(-203.316072549381,-67.457039139711,17.));
#16301=CARTESIAN_POINT('Ctrl Pts',(-203.394952319029,-67.5215327177357,
17.));
#16302=CARTESIAN_POINT('Ctrl Pts',(-203.476670785051,-67.5817955879554,
17.));
#16303=CARTESIAN_POINT('Ctrl Pts',(-203.558482237366,-67.6421270304475,
17.));
#16304=CARTESIAN_POINT('Ctrl Pts',(-203.643139431469,-67.6982189644735,
17.));
#16305=CARTESIAN_POINT('Ctrl Pts',(-203.730355930017,-67.7497653639998,
17.));
#16306=CARTESIAN_POINT('Ctrl Pts',(-203.815753640172,-67.8002368293722,
17.));
#16307=CARTESIAN_POINT('Ctrl Pts',(-203.903605699369,-67.8463510305609,
17.));
#16308=CARTESIAN_POINT('Ctrl Pts',(-203.993677035266,-67.8877849551271,
17.));
#16309=CARTESIAN_POINT('Ctrl Pts',(-204.044060944389,-67.9109621742627,
17.));
#16310=CARTESIAN_POINT('Ctrl Pts',(-204.095139826534,-67.9326742194188,
17.));
#16311=CARTESIAN_POINT('Ctrl Pts',(-204.146876136319,-67.9528583341107,
17.));
#16312=CARTESIAN_POINT('Ctrl Pts',(-204.165972573965,-67.9603085115445,
17.));
#16313=CARTESIAN_POINT('Ctrl Pts',(-204.185158603728,-67.9675504698475,
17.));
#16314=CARTESIAN_POINT('Ctrl Pts',(-204.204431258832,-67.9745848956374,
17.));
#16315=CARTESIAN_POINT('Ctrl Pts',(-205.793799282533,-67.9692229537457,
17.));
#16316=CARTESIAN_POINT('Ctrl Pts',(-205.888627148018,-67.9345344969579,
17.));
#16317=CARTESIAN_POINT('Ctrl Pts',(-205.981409263194,-67.8948513145698,
17.));
#16318=CARTESIAN_POINT('Ctrl Pts',(-206.071905763361,-67.8504949414992,
17.));
#16319=CARTESIAN_POINT('Ctrl Pts',(-206.16368767609,-67.8055085303715,17.));
#16320=CARTESIAN_POINT('Ctrl Pts',(-206.253119250409,-67.7557145264303,
17.));
#16321=CARTESIAN_POINT('Ctrl Pts',(-206.339916218874,-67.701407654434,17.));
#16322=CARTESIAN_POINT('Ctrl Pts',(-206.364296575079,-67.6861534248557,
17.));
#16323=CARTESIAN_POINT('Ctrl Pts',(-206.388468826147,-67.6705429272934,
17.));
#16324=CARTESIAN_POINT('Ctrl Pts',(-206.412426086333,-67.6545822455055,
17.));
#16325=CARTESIAN_POINT('Ctrl Pts',(-206.431863526899,-67.6416327345333,
17.));
#16326=CARTESIAN_POINT('Ctrl Pts',(-206.451161651935,-67.6284510097797,
17.));
#16327=CARTESIAN_POINT('Ctrl Pts',(-206.470297235862,-67.6150542711723,
17.));
#16328=CARTESIAN_POINT('Ctrl Pts',(-206.553008824826,-67.5571482495228,
17.));
#16329=CARTESIAN_POINT('Ctrl Pts',(-206.632764547703,-67.495177621976,17.));
#16330=CARTESIAN_POINT('Ctrl Pts',(-206.709298974822,-67.4294411381943,
17.));
#16331=CARTESIAN_POINT('Ctrl Pts',(-206.768827144667,-67.378311565284,17.));
#16332=CARTESIAN_POINT('Ctrl Pts',(-206.826405917082,-67.3249028587324,
17.));
#16333=CARTESIAN_POINT('Ctrl Pts',(-206.881892272758,-67.2693434657245,
17.));
#16334=CARTESIAN_POINT('Ctrl Pts',(-206.912069662648,-67.2391263529871,
17.));
#16335=CARTESIAN_POINT('Ctrl Pts',(-206.941627832692,-67.2082729188649,
17.));
#16336=CARTESIAN_POINT('Ctrl Pts',(-206.970541519969,-67.1768029072482,
17.));
#16337=CARTESIAN_POINT('Ctrl Pts',(-206.982346348857,-67.1639543867987,
17.));
#16338=CARTESIAN_POINT('Ctrl Pts',(-206.994038644047,-67.1510085536672,
17.));
#16339=CARTESIAN_POINT('Ctrl Pts',(-207.005612030979,-67.1379726476749,
17.));
#16340=CARTESIAN_POINT('Ctrl Pts',(-207.071011723905,-67.0643084511959,
17.));
#16341=CARTESIAN_POINT('Ctrl Pts',(-207.132669244518,-66.9877146035452,
17.));
#16342=CARTESIAN_POINT('Ctrl Pts',(-207.190339462795,-66.9084693768327,
17.));
#16343=CARTESIAN_POINT('Ctrl Pts',(-207.247552243663,-66.8298527194637,
17.));
#16344=CARTESIAN_POINT('Ctrl Pts',(-207.300841167328,-66.7486257942039,
17.));
#16345=CARTESIAN_POINT('Ctrl Pts',(-207.349920589594,-66.6650384656478,
17.));
#16346=CARTESIAN_POINT('Ctrl Pts',(-207.397481339409,-66.5840375932332,
17.));
#16347=CARTESIAN_POINT('Ctrl Pts',(-207.44108925285,-66.500819434757,17.));
#16348=CARTESIAN_POINT('Ctrl Pts',(-207.480436480452,-66.4156016691333,
17.));
#16349=CARTESIAN_POINT('Ctrl Pts',(-207.501052397794,-66.3709519563276,
17.));
#16350=CARTESIAN_POINT('Ctrl Pts',(-207.520497841185,-66.3257532073699,
17.));
#16351=CARTESIAN_POINT('Ctrl Pts',(-207.538722766342,-66.280036559567,17.));
#16352=CARTESIAN_POINT('Ctrl Pts',(-207.545019324992,-66.2642418415239,
17.));
#16353=CARTESIAN_POINT('Ctrl Pts',(-207.551170160701,-66.2483853062549,
17.));
#16354=CARTESIAN_POINT('Ctrl Pts',(-207.557173092316,-66.2324682453042,
17.));
#16355=CARTESIAN_POINT('Ctrl Pts',(-207.562735046531,-66.2177204570677,
17.));
#16356=CARTESIAN_POINT('Ctrl Pts',(-207.568167259183,-66.2029279237178,
17.));
#16357=CARTESIAN_POINT('Ctrl Pts',(-207.573465901499,-66.1880990080578,
17.));
#16358=CARTESIAN_POINT('Ctrl Pts',(-207.604700042699,-66.1006863430889,
17.));
#16359=CARTESIAN_POINT('Ctrl Pts',(-207.631326666905,-66.0119317997892,
17.));
#16360=CARTESIAN_POINT('Ctrl Pts',(-207.653093540636,-65.9220590100927,
17.));
#16361=CARTESIAN_POINT('Ctrl Pts',(-207.65825467588,-65.9007493067314,17.));
#16362=CARTESIAN_POINT('Ctrl Pts',(-207.663142365404,-65.8793766928838,
17.));
#16363=CARTESIAN_POINT('Ctrl Pts',(-207.667752815749,-65.8579440884434,
17.));
#16364=CARTESIAN_POINT('Ctrl Pts',(-207.687563008922,-65.7658524265826,
17.));
#16365=CARTESIAN_POINT('Ctrl Pts',(-207.702258795435,-65.6726527986311,
17.));
#16366=CARTESIAN_POINT('Ctrl Pts',(-207.711951637232,-65.5787373627011,
17.));
#16367=CARTESIAN_POINT('Ctrl Pts',(-207.722120050741,-65.480214039264,17.));
#16368=CARTESIAN_POINT('Ctrl Pts',(-207.726782566171,-65.3809016624173,
17.));
#16369=CARTESIAN_POINT('Ctrl Pts',(-207.726009593431,-65.2812689631459,
17.));
#16370=CARTESIAN_POINT('Ctrl Pts',(-207.725769513995,-65.2503238068458,
17.));
#16371=CARTESIAN_POINT('Ctrl Pts',(-207.725004679199,-65.2193479400861,
17.));
#16372=CARTESIAN_POINT('Ctrl Pts',(-207.723716132524,-65.188356011546,17.));
#16373=CARTESIAN_POINT('Ctrl Pts',(-207.723127462139,-65.1741974010323,
17.));
#16374=CARTESIAN_POINT('Ctrl Pts',(-207.722429402964,-65.1600353565386,
17.));
#16375=CARTESIAN_POINT('Ctrl Pts',(-207.721623066916,-65.1458857972683,
17.));
#16376=CARTESIAN_POINT('Ctrl Pts',(-207.716331511517,-65.0530297517173,
17.));
#16377=CARTESIAN_POINT('Ctrl Pts',(-207.706375521326,-64.9605544163374,
17.));
#16378=CARTESIAN_POINT('Ctrl Pts',(-207.69188291931,-64.8688309918216,17.));
#16379=CARTESIAN_POINT('Ctrl Pts',(-207.677420951151,-64.7773014484522,
17.));
#16380=CARTESIAN_POINT('Ctrl Pts',(-207.658441112453,-64.6865196943256,
17.));
#16381=CARTESIAN_POINT('Ctrl Pts',(-207.635021694811,-64.5968715427646,
17.));
#16382=CARTESIAN_POINT('Ctrl Pts',(-207.611997353704,-64.508735720912,17.));
#16383=CARTESIAN_POINT('Ctrl Pts',(-207.58468148308,-64.4216947907291,17.));
#16384=CARTESIAN_POINT('Ctrl Pts',(-207.553108101053,-64.3361444936322,
17.));
#16385=CARTESIAN_POINT('Ctrl Pts',(-207.536805168121,-64.2919705513309,
17.));
#16386=CARTESIAN_POINT('Ctrl Pts',(-207.519366487178,-64.2481945888456,
17.));
#16387=CARTESIAN_POINT('Ctrl Pts',(-207.500793029987,-64.2048752352537,
17.));
#16388=CARTESIAN_POINT('Ctrl Pts',(-207.494982654184,-64.191323545803,17.));
#16389=CARTESIAN_POINT('Ctrl Pts',(-207.489060435718,-64.1778148479559,
17.));
#16390=CARTESIAN_POINT('Ctrl Pts',(-207.483028790468,-64.1643564201991,
17.));
#16391=CARTESIAN_POINT('Ctrl Pts',(-207.44648471981,-64.0828155280312,17.));
#16392=CARTESIAN_POINT('Ctrl Pts',(-207.406050937059,-64.003390750436,17.));
#16393=CARTESIAN_POINT('Ctrl Pts',(-207.36180715762,-63.9264273776788,17.));
#16394=CARTESIAN_POINT('Ctrl Pts',(-207.318274262746,-63.8507006098065,
17.));
#16395=CARTESIAN_POINT('Ctrl Pts',(-207.271052355616,-63.7773560957185,
17.));
#16396=CARTESIAN_POINT('Ctrl Pts',(-207.22018022953,-63.7067557020002,17.));
#16397=CARTESIAN_POINT('Ctrl Pts',(-207.170937081922,-63.6384160064454,
17.));
#16398=CARTESIAN_POINT('Ctrl Pts',(-207.118273277825,-63.5726470624006,
17.));
#16399=CARTESIAN_POINT('Ctrl Pts',(-207.062195778224,-63.5098162258635,
17.));
#16400=CARTESIAN_POINT('Ctrl Pts',(-207.027350701924,-63.470774804462,17.));
#16401=CARTESIAN_POINT('Ctrl Pts',(-206.99118704962,-63.4328686004809,17.));
#16402=CARTESIAN_POINT('Ctrl Pts',(-206.953701849393,-63.3961948658342,
17.));
#16403=CARTESIAN_POINT('Ctrl Pts',(-206.941653045689,-63.3844068901223,
17.));
#16404=CARTESIAN_POINT('Ctrl Pts',(-206.929467677439,-63.372746308816,17.));
#16405=CARTESIAN_POINT('Ctrl Pts',(-206.917148223239,-63.3612143401441,
17.));
#16406=CARTESIAN_POINT('Origin',(-205.,-65.,-2.20842344717744));
#16407=CARTESIAN_POINT('Ctrl Pts',(-201.923731533573,-64.9977249101301,
0.291576552822544));
#16408=CARTESIAN_POINT('Ctrl Pts',(-201.922495961988,-64.8497482855437,
0.299259877064294));
#16409=CARTESIAN_POINT('Ctrl Pts',(-201.999549636482,-63.6828739087284,
0.359912640907479));
#16410=CARTESIAN_POINT('Ctrl Pts',(-203.493276918295,-61.6929032503864,
0.473534844352099));
#16411=CARTESIAN_POINT('Ctrl Pts',(-206.963857847912,-61.9425259124891,
0.632443163156407));
#16412=CARTESIAN_POINT('Ctrl Pts',(-208.633920228955,-64.9948075983619,
0.791351481960713));
#16413=CARTESIAN_POINT('Ctrl Pts',(-206.972481892344,-68.0520434541846,
0.950259800765019));
#16414=CARTESIAN_POINT('Ctrl Pts',(-203.502676360176,-68.3111058299649,
1.10916811956933));
#16415=CARTESIAN_POINT('Ctrl Pts',(-202.001256755867,-66.3232551853252,
1.22294037025517));
#16416=CARTESIAN_POINT('Ctrl Pts',(-201.922527589981,-65.1532534982625,
1.28374318133957));
#16417=CARTESIAN_POINT('Ctrl Pts',(-201.92380386931,-65.0023470817023,1.29157655282254));
#16418=CARTESIAN_POINT('Ctrl Pts',(-201.92961158086,-65.0031570762977,0.208423447177454));
#16419=CARTESIAN_POINT('Ctrl Pts',(-201.934956999492,-64.2978727303493,
0.24488784398784));
#16420=CARTESIAN_POINT('Ctrl Pts',(-202.525030743872,-62.5576537690219,
0.334321680399662));
#16421=CARTESIAN_POINT('Ctrl Pts',(-205.417645988708,-61.3907533400893,
0.47672495641292));
#16422=CARTESIAN_POINT('Ctrl Pts',(-208.260115801475,-63.3950087136501,
0.635633275217226));
#16423=CARTESIAN_POINT('Ctrl Pts',(-208.114970263096,-66.8719143799143,
0.794541594021533));
#16424=CARTESIAN_POINT('Ctrl Pts',(-205.113461147179,-68.6320808995075,
0.95344991282584));
#16425=CARTESIAN_POINT('Ctrl Pts',(-202.417561254516,-67.269564439631,1.09141053054448));
#16426=CARTESIAN_POINT('Ctrl Pts',(-201.933595089404,-65.6186981664531,
1.17640170866168));
#16427=CARTESIAN_POINT('Ctrl Pts',(-201.930556952874,-64.9983469618497,
1.20842344717745));
#16428=CARTESIAN_POINT('Ctrl Pts',(-206.913465996665,-63.364012796625,-1.94289029309402E-15));
#16429=CARTESIAN_POINT('Ctrl Pts',(-207.457950030113,-64.0008464354095,
0.0529694396014337));
#16430=CARTESIAN_POINT('Ctrl Pts',(-207.85066103992,-65.8508593102597,0.158908318804304));
#16431=CARTESIAN_POINT('Ctrl Pts',(-205.826538448717,-67.8612078721254,
0.317816637608612));
#16432=CARTESIAN_POINT('Ctrl Pts',(-203.043492499314,-67.2425410520485,
0.476724956412918));
#16433=CARTESIAN_POINT('Ctrl Pts',(-202.054683509666,-64.5708016763166,
0.635633275217225));
#16434=CARTESIAN_POINT('Ctrl Pts',(-203.765845011162,-62.291161195005,0.794541594021531));
#16435=CARTESIAN_POINT('Ctrl Pts',(-206.608593503211,-62.495626804845,0.953449912825838));
#16436=CARTESIAN_POINT('Ctrl Pts',(-207.97653950753,-64.9957469103226,1.11235823163015));
#16437=CARTESIAN_POINT('Ctrl Pts',(-206.615657447202,-67.4999249701999,
1.27126655043445));
#16438=CARTESIAN_POINT('Ctrl Pts',(-203.773544082233,-67.7121226376889,
1.43017486923876));
#16439=CARTESIAN_POINT('Ctrl Pts',(-202.055838893905,-65.4379140446217,
1.58908318804307));
#16440=CARTESIAN_POINT('Ctrl Pts',(-203.037304253044,-62.7622125536136,
1.74799150684737));
#16441=CARTESIAN_POINT('Ctrl Pts',(-205.818148811342,-62.1380984208763,
1.90689982565168));
#16442=CARTESIAN_POINT('Ctrl Pts',(-207.848922870067,-64.1377393756635,
2.06580814445599));
#16443=CARTESIAN_POINT('Ctrl Pts',(-207.267836678543,-66.9278933189866,
2.22471646326029));
#16444=CARTESIAN_POINT('Ctrl Pts',(-204.607622975304,-67.9505752021356,
2.3836247820646));
#16445=CARTESIAN_POINT('Ctrl Pts',(-202.307136236037,-66.2682032099886,
2.5425331008689));
#16446=CARTESIAN_POINT('Ctrl Pts',(-202.475436852696,-63.4231564503584,
2.70144141967321));
#16447=CARTESIAN_POINT('Ctrl Pts',(-204.958228768284,-62.0237423490828,
2.86034973847752));
#16448=CARTESIAN_POINT('Ctrl Pts',(-207.479316071554,-63.3529279407582,
3.01925805728183));
#16449=CARTESIAN_POINT('Ctrl Pts',(-207.727394116418,-66.1921308147553,
3.17816637608613));
#16450=CARTESIAN_POINT('Ctrl Pts',(-205.475027716348,-67.9384014686786,
3.33707469489044));
#16451=CARTESIAN_POINT('Ctrl Pts',(-202.787161216442,-66.9907785044862,
3.49598301369474));
#16452=CARTESIAN_POINT('Ctrl Pts',(-202.128000580265,-64.2180320547611,
3.65489133249906));
#16453=CARTESIAN_POINT('Ctrl Pts',(-204.101856912646,-62.162185078862,3.81379965130335));
#16454=CARTESIAN_POINT('Ctrl Pts',(-206.899120789014,-62.7080151042509,
3.97270797010767));
#16455=CARTESIAN_POINT('Ctrl Pts',(-207.955291952161,-65.3551112653809,
4.13161628891197));
#16456=CARTESIAN_POINT('Ctrl Pts',(-206.302084484222,-67.6766453872404,
4.29052460771628));
#16457=CARTESIAN_POINT('Ctrl Pts',(-203.455140514293,-67.5442609344747,
4.44943292652058));
#16458=CARTESIAN_POINT('Ctrl Pts',(-202.024506454277,-65.07932649362,4.60834124532489));
#16459=CARTESIAN_POINT('Ctrl Pts',(-203.321771620508,-62.5416664100502,
4.7672495641292));
#16460=CARTESIAN_POINT('Ctrl Pts',(-206.157617807844,-62.2577790854505,
4.92615788293351));
#16461=CARTESIAN_POINT('Ctrl Pts',(-207.932172927404,-64.4879292460782,
5.08506620173781));
#16462=CARTESIAN_POINT('Ctrl Pts',(-207.018544679411,-67.1875401505902,
5.24397452054212));
#16463=CARTESIAN_POINT('Ctrl Pts',(-204.25433723019,-67.8816386947262,5.40288283934643));
#16464=CARTESIAN_POINT('Ctrl Pts',(-202.173745074213,-65.9338830910165,
5.56179115815073));
#16465=CARTESIAN_POINT('Ctrl Pts',(-202.68423184573,-63.1299539072815,5.72069947695504));
#16466=CARTESIAN_POINT('Ctrl Pts',(-205.31778897822,-62.040462080232,5.87960779575935));
#16467=CARTESIAN_POINT('Ctrl Pts',(-207.66000072734,-63.6642415398826,6.03851611456366));
#16468=CARTESIAN_POINT('Ctrl Pts',(-207.563553539912,-66.5126294262725,
6.19742443336796));
#16469=CARTESIAN_POINT('Ctrl Pts',(-205.116869119401,-67.9742555610023,
6.35633275217227));
#16470=CARTESIAN_POINT('Ctrl Pts',(-202.563040396445,-66.7091174400446,
6.51524107097658));
#16471=CARTESIAN_POINT('Ctrl Pts',(-202.243389000634,-63.8770795525063,
6.67414938978088));
#16472=CARTESIAN_POINT('Ctrl Pts',(-204.450967758971,-62.0745225805805,
6.83305770858518));
#16473=CARTESIAN_POINT('Ctrl Pts',(-207.161893139463,-62.9540106093222,
6.99196602738949));
#16474=CARTESIAN_POINT('Ctrl Pts',(-207.890819052728,-65.709238843837,7.15087434619381));
#16475=CARTESIAN_POINT('Ctrl Pts',(-205.969474368539,-67.8142448333378,
7.3097826649981));
#16476=CARTESIAN_POINT('Ctrl Pts',(-203.159326418888,-67.3391826138673,
7.46869098380242));
#16477=CARTESIAN_POINT('Ctrl Pts',(-202.036687435572,-64.7195839185636,
7.62759930260671));
#16478=CARTESIAN_POINT('Ctrl Pts',(-203.630780290992,-62.3570675525683,
7.78650762141104));
#16479=CARTESIAN_POINT('Ctrl Pts',(-206.480158472145,-62.4175621148688,
7.94541594021532));
#16480=CARTESIAN_POINT('Ctrl Pts',(-207.97254390946,-64.8456068668834,8.10432425901965));
#16481=CARTESIAN_POINT('Ctrl Pts',(-206.739734314091,-67.415197517719,8.26323257782394));
#16482=CARTESIAN_POINT('Ctrl Pts',(-203.911955744214,-67.7705620784733,
8.42214089662826));
#16483=CARTESIAN_POINT('Ctrl Pts',(-202.081683987196,-65.5859062916828,
8.58104921543255));
#16484=CARTESIAN_POINT('Ctrl Pts',(-202.926891733301,-62.8640981652309,
8.73995753423687));
#16485=CARTESIAN_POINT('Ctrl Pts',(-205.672701967614,-62.1004609683623,
8.89886585304117));
#16486=CARTESIAN_POINT('Ctrl Pts',(-207.801786556669,-63.9950887481507,
9.05777417184549));
#16487=CARTESIAN_POINT('Ctrl Pts',(-207.362224545558,-66.8110079319493,
9.21668249064978));
#16488=CARTESIAN_POINT('Ctrl Pts',(-204.757001473176,-67.966615284998,9.37559080945409));
#16489=CARTESIAN_POINT('Ctrl Pts',(-202.374556734241,-66.4024629020062,
9.53449912825839));
#16490=CARTESIAN_POINT('Ctrl Pts',(-202.399089037318,-63.5525482054929,
9.69340744706271));
#16491=CARTESIAN_POINT('Ctrl Pts',(-204.808107441137,-62.0296411363144,
9.85231576586701));
#16492=CARTESIAN_POINT('Ctrl Pts',(-207.393050798179,-63.2299258742758,
10.0112240846713));
#16493=CARTESIAN_POINT('Ctrl Pts',(-207.784071930084,-66.0529947869487,
10.1701324034756));
#16494=CARTESIAN_POINT('Ctrl Pts',(-205.622687033484,-67.910689848052,10.3290407222799));
#16495=CARTESIAN_POINT('Ctrl Pts',(-202.890429624231,-67.0998969886399,
10.4879490410842));
#16496=CARTESIAN_POINT('Ctrl Pts',(-202.09220275725,-64.3639420401572,10.6468573598885));
#16497=CARTESIAN_POINT('Ctrl Pts',(-203.959811902574,-62.2111179201701,
10.8057656786929));
#16498=CARTESIAN_POINT('Ctrl Pts',(-206.781053869651,-62.6151097202126,
10.9646739974972));
#16499=CARTESIAN_POINT('Ctrl Pts',(-207.969445555503,-65.2055422733386,
11.1235823163015));
#16500=CARTESIAN_POINT('Ctrl Pts',(-206.435482744948,-67.6075359675713,
11.2824906351058));
#16501=CARTESIAN_POINT('Ctrl Pts',(-203.58548539792,-67.618969830625,11.4413989539101));
#16502=CARTESIAN_POINT('Ctrl Pts',(-202.032299228341,-65.229361424646,11.6003072727144));
#16503=CARTESIAN_POINT('Ctrl Pts',(-203.199867956841,-62.6294770280768,
11.7592155915187));
#16504=CARTESIAN_POINT('Ctrl Pts',(-206.017777622806,-62.2028615973215,
11.918123910323));
#16505=CARTESIAN_POINT('Ctrl Pts',(-207.902600139672,-64.3406313911045,
12.0770322291273));
#16506=CARTESIAN_POINT('Ctrl Pts',(-207.126351290249,-67.0829029558956,
12.2359405479316));
#16507=CARTESIAN_POINT('Ctrl Pts',(-204.400687343713,-67.9155923708988,
12.3948488667359));
#16508=CARTESIAN_POINT('Ctrl Pts',(-202.22446654207,-66.0752992872318,12.5537571855402));
#16509=CARTESIAN_POINT('Ctrl Pts',(-202.592823793087,-63.2491838354354,
12.7126655043445));
#16510=CARTESIAN_POINT('Ctrl Pts',(-205.168053286105,-62.0281970747873,
12.8715738231488));
#16511=CARTESIAN_POINT('Ctrl Pts',(-207.589213404689,-63.5317260207767,
13.0304821419532));
#16512=CARTESIAN_POINT('Ctrl Pts',(-207.636611613018,-66.3813521402626,
13.1893904607575));
#16513=CARTESIAN_POINT('Ctrl Pts',(-205.266793763269,-67.9645700567683,
13.3482987795618));
#16514=CARTESIAN_POINT('Ctrl Pts',(-202.652382373513,-66.8299032793574,
13.5072070983661));
#16515=CARTESIAN_POINT('Ctrl Pts',(-202.190240584349,-64.0176016284133,
13.6661154171704));
#16516=CARTESIAN_POINT('Ctrl Pts',(-204.304054824455,-62.1059518233833,
13.8250237359747));
#16517=CARTESIAN_POINT('Ctrl Pts',(-207.055903820797,-62.8475330427476,
13.983932054779));
#16518=CARTESIAN_POINT('Ctrl Pts',(-207.922923177315,-65.5624719062102,
14.1428403735833));
#16519=CARTESIAN_POINT('Ctrl Pts',(-206.110239224163,-67.7617428222285,
14.3017486923876));
#16520=CARTESIAN_POINT('Ctrl Pts',(-203.279700379008,-67.4290787666223,
14.4606570111919));
#16521=CARTESIAN_POINT('Ctrl Pts',(-202.026312958194,-64.8694624875084,
14.6195653299962));
#16522=CARTESIAN_POINT('Ctrl Pts',(-203.499168664916,-62.4295214576422,
14.7784736488005));
#16523=CARTESIAN_POINT('Ctrl Pts',(-206.34796959245,-62.3461665970152,14.9373819676048));
#16524=CARTESIAN_POINT('Ctrl Pts',(-207.960967419167,-64.6958161862147,
15.0962902864091));
#16525=CARTESIAN_POINT('Ctrl Pts',(-206.85938267811,-67.3243388221629,15.2551986052134));
#16526=CARTESIAN_POINT('Ctrl Pts',(-204.053138186676,-67.8219321098425,
15.4141069240177));
#16527=CARTESIAN_POINT('Ctrl Pts',(-202.114962920394,-65.7324126566496,
15.5730152428221));
#16528=CARTESIAN_POINT('Ctrl Pts',(-202.821763790211,-62.9714191306523,
15.7319235616264));
#16529=CARTESIAN_POINT('Ctrl Pts',(-205.525534122556,-62.0702189149839,
15.8908318804307));
#16530=CARTESIAN_POINT('Ctrl Pts',(-207.747527714867,-63.8549824021587,
16.049740199235));
#16531=CARTESIAN_POINT('Ctrl Pts',(-207.450562878104,-66.6895405023604,
16.2086485180393));
#16532=CARTESIAN_POINT('Ctrl Pts',(-204.907064112986,-67.975032954454,16.3675568368436));
#16533=CARTESIAN_POINT('Ctrl Pts',(-202.448531736689,-66.5332827231908,
16.5264651556479));
#16534=CARTESIAN_POINT('Ctrl Pts',(-202.329643199581,-63.6853536643865,
16.6853734744522));
#16535=CARTESIAN_POINT('Ctrl Pts',(-204.657906690574,-62.0436704956976,
16.8442817932565));
#16536=CARTESIAN_POINT('Ctrl Pts',(-207.301858842744,-63.1102587047955,
17.0031901120608));
#16537=CARTESIAN_POINT('Ctrl Pts',(-207.831197343881,-65.9135379195059,
17.1620984308651));
#16538=CARTESIAN_POINT('Ctrl Pts',(-206.459639356019,-67.2156893163364,
17.268037310068));
#16539=CARTESIAN_POINT('Ctrl Pts',(-205.650199997975,-67.4320868020351,
17.3210067496694));
#16540=CARTESIAN_POINT('Ctrl Pts',(-207.054331550342,-63.2435746787731,
-0.107002249889813));
#16541=CARTESIAN_POINT('Ctrl Pts',(-207.63889941333,-63.9272907410153,-0.054032810288377));
#16542=CARTESIAN_POINT('Ctrl Pts',(-208.060521025117,-65.9134978771587,
0.051906068914494));
#16543=CARTESIAN_POINT('Ctrl Pts',(-205.887386562254,-68.0718442940919,
0.210814387718801));
#16544=CARTESIAN_POINT('Ctrl Pts',(-202.899458315881,-67.4076324555492,
0.369722706523107));
#16545=CARTESIAN_POINT('Ctrl Pts',(-201.837855178832,-64.5392049509981,
0.528631025327414));
#16546=CARTESIAN_POINT('Ctrl Pts',(-203.674988980207,-62.0917418801321,
0.687539344131721));
#16547=CARTESIAN_POINT('Ctrl Pts',(-206.727014951444,-62.3112598407265,
0.846447662936028));
#16548=CARTESIAN_POINT('Ctrl Pts',(-208.195666414672,-64.9954338063356,
1.00535598174033));
#16549=CARTESIAN_POINT('Ctrl Pts',(-206.734598928916,-67.6839644648615,
1.16426430054464));
#16550=CARTESIAN_POINT('Ctrl Pts',(-203.683254841548,-67.9117837017809,
1.32317261934895));
#16551=CARTESIAN_POINT('Ctrl Pts',(-201.839095620156,-65.4701524039476,
1.48208093815325));
#16552=CARTESIAN_POINT('Ctrl Pts',(-202.892814503252,-62.5974711010892,
1.64098925695756));
#16553=CARTESIAN_POINT('Ctrl Pts',(-205.878379296494,-61.9274109295829,
1.79989757576187));
#16554=CARTESIAN_POINT('Ctrl Pts',(-208.058654894662,-64.0742614667419,
1.95880589456618));
#16555=CARTESIAN_POINT('Ctrl Pts',(-207.434790295659,-67.0698209833833,
2.11771421337048));
#16556=CARTESIAN_POINT('Ctrl Pts',(-204.578736960642,-68.1677906688536,
2.27662253217479));
#16557=CARTESIAN_POINT('Ctrl Pts',(-202.108892971851,-66.3615658031371,
2.4355308509791));
#16558=CARTESIAN_POINT('Ctrl Pts',(-202.289583544533,-63.3070723704377,
2.5944391697834));
#16559=CARTESIAN_POINT('Ctrl Pts',(-204.955153653443,-61.8046361916634,
2.75334748858771));
#16560=CARTESIAN_POINT('Ctrl Pts',(-207.661838380165,-63.2316737779064,
2.91225580739202));
#16561=CARTESIAN_POINT('Ctrl Pts',(-207.928179436342,-66.2798931097576,
3.07116412619632));
#16562=CARTESIAN_POINT('Ctrl Pts',(-205.50999831023,-68.1547207293982,3.23007244500063));
#16563=CARTESIAN_POINT('Ctrl Pts',(-202.624256434759,-67.1373356509271,
3.38898076380493));
#16564=CARTESIAN_POINT('Ctrl Pts',(-201.916569706068,-64.160465132874,3.54788908260924));
#16565=CARTESIAN_POINT('Ctrl Pts',(-204.035737408301,-61.9532707993317,
3.70679740141355));
#16566=CARTESIAN_POINT('Ctrl Pts',(-207.038930277089,-62.5392837435045,
3.86570572021786));
#16567=CARTESIAN_POINT('Ctrl Pts',(-208.172854656617,-65.3812538491018,
4.02461403902216));
#16568=CARTESIAN_POINT('Ctrl Pts',(-206.397941349264,-67.8736946868505,
4.18352235782647));
#16569=CARTESIAN_POINT('Ctrl Pts',(-203.341411037424,-67.7315643544771,
4.34243067663077));
#16570=CARTESIAN_POINT('Ctrl Pts',(-201.80545654876,-65.085166352005,4.50133899543508));
#16571=CARTESIAN_POINT('Ctrl Pts',(-203.198223791445,-62.3606887899229,
4.66024731423939));
#16572=CARTESIAN_POINT('Ctrl Pts',(-206.242839324052,-62.0559022461933,
4.8191556330437));
#16573=CARTESIAN_POINT('Ctrl Pts',(-208.148033655327,-64.450231617587,4.978063951848));
#16574=CARTESIAN_POINT('Ctrl Pts',(-207.167145916319,-67.3485824973268,
5.13697227065231));
#16575=CARTESIAN_POINT('Ctrl Pts',(-204.199443022972,-68.0937791931397,
5.29588058945662));
#16576=CARTESIAN_POINT('Ctrl Pts',(-201.965681818504,-66.0026337032119,
5.45478890826092));
#16577=CARTESIAN_POINT('Ctrl Pts',(-202.513749608885,-62.9922848404093,
5.61369722706523));
#16578=CARTESIAN_POINT('Ctrl Pts',(-205.341183969533,-61.8225867961021,
5.77260554586953));
#16579=CARTESIAN_POINT('Ctrl Pts',(-207.855824680256,-63.5659056638381,
5.93151386467385));
#16580=CARTESIAN_POINT('Ctrl Pts',(-207.752277243082,-66.6239861903914,
6.09042218347815));
#16581=CARTESIAN_POINT('Ctrl Pts',(-205.125472791084,-68.1932143285518,
6.24933050228246));
#16582=CARTESIAN_POINT('Ctrl Pts',(-202.383636286604,-66.8349392601922,
6.40823882108676));
#16583=CARTESIAN_POINT('Ctrl Pts',(-202.040452792008,-63.7944123868251,
6.56714713989107));
#16584=CARTESIAN_POINT('Ctrl Pts',(-204.410549099453,-61.8591547626134,
6.72605545869538));
#16585=CARTESIAN_POINT('Ctrl Pts',(-207.321047404347,-62.8033889474597,
6.88496377749968));
#16586=CARTESIAN_POINT('Ctrl Pts',(-208.103635390804,-65.7614515942076,
7.04387209630399));
#16587=CARTESIAN_POINT('Ctrl Pts',(-206.040845139662,-68.0214239299728,
7.2027804151083));
#16588=CARTESIAN_POINT('Ctrl Pts',(-203.023819697789,-67.5113885765698,
7.36168873391261));
#16589=CARTESIAN_POINT('Ctrl Pts',(-201.818534269624,-64.6989402454383,
7.52059705271691));
#16590=CARTESIAN_POINT('Ctrl Pts',(-203.529981064483,-62.1625001324065,
7.67950537152122));
#16591=CARTESIAN_POINT('Ctrl Pts',(-206.589124789326,-62.227448183835,7.83841369032552));
#16592=CARTESIAN_POINT('Ctrl Pts',(-208.191376668634,-64.8342407520852,
7.99732200912984));
#16593=CARTESIAN_POINT('Ctrl Pts',(-206.867810087495,-67.5929995461668,
8.15623032793414));
#16594=CARTESIAN_POINT('Ctrl Pts',(-203.831856094268,-67.9745253377426,
8.31513864673845));
#16595=CARTESIAN_POINT('Ctrl Pts',(-201.866843377713,-65.6290395453307,
8.47404696554276));
#16596=CARTESIAN_POINT('Ctrl Pts',(-202.774273633827,-62.7068573284045,
8.63295528434705));
#16597=CARTESIAN_POINT('Ctrl Pts',(-205.722224945965,-61.8870026828157,
8.79186360315137));
#16598=CARTESIAN_POINT('Ctrl Pts',(-208.008048499801,-63.921109184294,8.95077192195566));
#16599=CARTESIAN_POINT('Ctrl Pts',(-207.536126809356,-66.944330727072,9.10968024075998));
#16600=CARTESIAN_POINT('Ctrl Pts',(-204.739112405858,-68.185011590653,9.26858855956428));
#16601=CARTESIAN_POINT('Ctrl Pts',(-202.181276832783,-66.5057094261393,
9.42749687836859));
#16602=CARTESIAN_POINT('Ctrl Pts',(-202.207615155126,-63.4459896887441,
9.5864051971729));
#16603=CARTESIAN_POINT('Ctrl Pts',(-204.793980693342,-61.8109692358563,
9.7453135159772));
#16604=CARTESIAN_POINT('Ctrl Pts',(-207.569222429266,-63.099616544398,9.90422183478152));
#16605=CARTESIAN_POINT('Ctrl Pts',(-207.989029757708,-66.1305141648425,
10.0631301535858));
#16606=CARTESIAN_POINT('Ctrl Pts',(-205.66852801205,-68.1249690344826,10.2220384723901));
#16607=CARTESIAN_POINT('Ctrl Pts',(-202.735127256945,-67.2544872204418,
10.3809467911944));
#16608=CARTESIAN_POINT('Ctrl Pts',(-201.878136518658,-64.3171167206374,
10.5398551099987));
#16609=CARTESIAN_POINT('Ctrl Pts',(-203.883235327643,-62.0058059789076,
10.698763428803));
#16610=CARTESIAN_POINT('Ctrl Pts',(-206.912171506397,-62.4395388502276,
10.8576717476073));
#16611=CARTESIAN_POINT('Ctrl Pts',(-208.188050220032,-65.2206738859141,
11.0165800664116));
#16612=CARTESIAN_POINT('Ctrl Pts',(-206.54116012412,-67.799497569421,11.175488385216));
#16613=CARTESIAN_POINT('Ctrl Pts',(-203.481351651642,-67.8117731706882,
11.3343967040203));
#16614=CARTESIAN_POINT('Ctrl Pts',(-201.813823011321,-65.2462465556759,
11.4933050228246));
#16615=CARTESIAN_POINT('Ctrl Pts',(-203.067345822979,-62.4549638506668,
11.6522133416289));
#16616=CARTESIAN_POINT('Ctrl Pts',(-206.092704383254,-61.9969418420234,
11.8111216604332));
#16617=CARTESIAN_POINT('Ctrl Pts',(-208.116283777892,-64.2920899880532,
11.9700299792375));
#16618=CARTESIAN_POINT('Ctrl Pts',(-207.28288903502,-67.2362421208711,12.1289382980418));
#16619=CARTESIAN_POINT('Ctrl Pts',(-204.356567140218,-68.130232471292,12.2878466168461));
#16620=CARTESIAN_POINT('Ctrl Pts',(-202.020137299752,-66.1544606779899,
12.4467549356504));
#16621=CARTESIAN_POINT('Ctrl Pts',(-202.415612277557,-63.1202922382824,
12.6056632544547));
#16622=CARTESIAN_POINT('Ctrl Pts',(-205.180425034146,-61.8094188653972,
12.764571573259));
#16623=CARTESIAN_POINT('Ctrl Pts',(-207.779826135971,-63.4236346162818,
12.9234798920633));
#16624=CARTESIAN_POINT('Ctrl Pts',(-207.830713705946,-66.483044532184,13.0823882108676));
#16625=CARTESIAN_POINT('Ctrl Pts',(-205.286434588476,-68.1828157967964,
13.241296529672));
#16626=CARTESIAN_POINT('Ctrl Pts',(-202.47955544199,-66.9646171123032,13.4002048484763));
#16627=CARTESIAN_POINT('Ctrl Pts',(-201.983391695226,-63.9452794179396,
13.5591131672806));
#16628=CARTESIAN_POINT('Ctrl Pts',(-204.252820727453,-61.8928977636416,
13.7180214860849));
#16629=CARTESIAN_POINT('Ctrl Pts',(-207.207255363249,-62.6890727146135,
13.8769298048892));
#16630=CARTESIAN_POINT('Ctrl Pts',(-208.138102957068,-65.6038799670978,
14.0358381236935));
#16631=CARTESIAN_POINT('Ctrl Pts',(-206.191972823453,-67.9650568254273,
14.1947464424978));
#16632=CARTESIAN_POINT('Ctrl Pts',(-203.153055348982,-67.607902704953,14.3536547613021));
#16633=CARTESIAN_POINT('Ctrl Pts',(-201.807396043895,-64.8598525759631,
14.5125630801064));
#16634=CARTESIAN_POINT('Ctrl Pts',(-203.388680452761,-62.2402879495917,
14.6714713989107));
#16635=CARTESIAN_POINT('Ctrl Pts',(-206.447204427723,-62.150796670228,14.830379717715));
#16636=CARTESIAN_POINT('Ctrl Pts',(-208.178947940194,-64.6734227799964,
14.9892880365193));
#16637=CARTESIAN_POINT('Ctrl Pts',(-206.996266725648,-67.4954520144994,
15.1481963553236));
#16638=CARTESIAN_POINT('Ctrl Pts',(-203.983432106807,-68.0296771284552,
15.3071046741279));
#16639=CARTESIAN_POINT('Ctrl Pts',(-201.902572239658,-65.7863314169405,
15.4660129929322));
#16640=CARTESIAN_POINT('Ctrl Pts',(-202.661406381056,-62.8220790494398,
15.6249213117365));
#16641=CARTESIAN_POINT('Ctrl Pts',(-205.564222897418,-61.8545342697314,
15.7838296305408));
#16642=CARTESIAN_POINT('Ctrl Pts',(-207.949795230189,-63.7706884883024,
15.9427379493452));
#16643=CARTESIAN_POINT('Ctrl Pts',(-207.63096843391,-66.8139211073671,16.1016462681495));
#16644=CARTESIAN_POINT('Ctrl Pts',(-204.900222358179,-68.1940489521602,
16.2605545869538));
#16645=CARTESIAN_POINT('Ctrl Pts',(-202.2606977275,-66.6461599418726,16.4194629057581));
#16646=CARTESIAN_POINT('Ctrl Pts',(-202.133056853201,-63.5885720208776,
16.5783712245624));
#16647=CARTESIAN_POINT('Ctrl Pts',(-204.632722462829,-61.8260314087208,
16.7372795433667));
#16648=CARTESIAN_POINT('Ctrl Pts',(-207.471317103792,-62.9711397163634,
16.896187862171));
#16649=CARTESIAN_POINT('Ctrl Pts',(-208.039624450561,-65.9807907607168,
17.0550961809753));
#16650=CARTESIAN_POINT('Ctrl Pts',(-206.56709509676,-67.3788039485619,17.1610350601782));
#16651=CARTESIAN_POINT('Ctrl Pts',(-205.698066426161,-67.6111321859386,
17.2140044997796));
#16652=CARTESIAN_POINT('Ctrl Pts',(-207.195197104019,-63.1231365609212,
-0.214004499779623));
#16653=CARTESIAN_POINT('Ctrl Pts',(-207.819848796546,-63.8537350466211,
-0.161035060178188));
#16654=CARTESIAN_POINT('Ctrl Pts',(-208.270381010313,-65.9761364440577,
-0.0550961809753165));
#16655=CARTESIAN_POINT('Ctrl Pts',(-205.948234675791,-68.2824807160583,
0.10381213782899));
#16656=CARTESIAN_POINT('Ctrl Pts',(-202.755424132447,-67.5727238590499,
0.262720456633297));
#16657=CARTESIAN_POINT('Ctrl Pts',(-201.621026847998,-64.5076082256796,
0.421628775437604));
#16658=CARTESIAN_POINT('Ctrl Pts',(-203.584132949251,-61.8923225652592,
0.58053709424191));
#16659=CARTESIAN_POINT('Ctrl Pts',(-206.845436399678,-62.1268928766078,
0.739445413046217));
#16660=CARTESIAN_POINT('Ctrl Pts',(-208.414793321813,-64.9951207023487,
0.898353731850525));
#16661=CARTESIAN_POINT('Ctrl Pts',(-206.85354041063,-67.8680039595231,1.05726205065483));
#16662=CARTESIAN_POINT('Ctrl Pts',(-203.592965600862,-68.1114447658729,
1.21617036945914));
#16663=CARTESIAN_POINT('Ctrl Pts',(-201.622352346407,-65.5023907632737,
1.37507868826344));
#16664=CARTESIAN_POINT('Ctrl Pts',(-202.74832475346,-62.4327296485647,1.53398700706775));
#16665=CARTESIAN_POINT('Ctrl Pts',(-205.938609781645,-61.7167234382895,
1.69289532587206));
#16666=CARTESIAN_POINT('Ctrl Pts',(-208.268386919257,-64.0107835578202,
1.85180364467636));
#16667=CARTESIAN_POINT('Ctrl Pts',(-207.601743912775,-67.2117486477801,
2.01071196348067));
#16668=CARTESIAN_POINT('Ctrl Pts',(-204.549850945981,-68.3850061355715,
2.16962028228498));
#16669=CARTESIAN_POINT('Ctrl Pts',(-201.910649707665,-66.4549283962856,
2.32852860108928));
#16670=CARTESIAN_POINT('Ctrl Pts',(-202.10373023637,-63.190988290517,2.48743691989359));
#16671=CARTESIAN_POINT('Ctrl Pts',(-204.952078538602,-61.585530034244,2.6463452386979));
#16672=CARTESIAN_POINT('Ctrl Pts',(-207.844360688776,-63.1104196150545,
2.8052535575022));
#16673=CARTESIAN_POINT('Ctrl Pts',(-208.128964756266,-66.3676554047598,
2.96416187630651));
#16674=CARTESIAN_POINT('Ctrl Pts',(-205.544968904111,-68.3710399901179,
3.12307019511081));
#16675=CARTESIAN_POINT('Ctrl Pts',(-202.461351653077,-67.2838927973679,
3.28197851391513));
#16676=CARTESIAN_POINT('Ctrl Pts',(-201.705138831871,-64.1028982109869,
3.44088683271943));
#16677=CARTESIAN_POINT('Ctrl Pts',(-203.969617903956,-61.7443565198013,
3.59979515152374));
#16678=CARTESIAN_POINT('Ctrl Pts',(-207.178739765165,-62.3705523827582,
3.75870347032805));
#16679=CARTESIAN_POINT('Ctrl Pts',(-208.390417361073,-65.4073964328226,
3.91761178913235));
#16680=CARTESIAN_POINT('Ctrl Pts',(-206.493798214305,-68.0707439864606,
4.07652010793666));
#16681=CARTESIAN_POINT('Ctrl Pts',(-203.227681560555,-67.9188677744795,
4.23542842674097));
#16682=CARTESIAN_POINT('Ctrl Pts',(-201.586406643242,-65.0910062103899,
4.39433674554527));
#16683=CARTESIAN_POINT('Ctrl Pts',(-203.074675962382,-62.1797111697955,
4.55324506434958));
#16684=CARTESIAN_POINT('Ctrl Pts',(-206.32806084026,-61.8540254069362,4.71215338315389));
#16685=CARTESIAN_POINT('Ctrl Pts',(-208.363894383249,-64.4125339890956,
4.87106170195819));
#16686=CARTESIAN_POINT('Ctrl Pts',(-207.315747153228,-67.5096248440634,
5.0299700207625));
#16687=CARTESIAN_POINT('Ctrl Pts',(-204.144548815754,-68.3059196915532,
5.1888783395668));
#16688=CARTESIAN_POINT('Ctrl Pts',(-201.757618562796,-66.0713843154072,
5.34778665837111));
#16689=CARTESIAN_POINT('Ctrl Pts',(-202.34326737204,-62.8546157735372,5.50669497717542));
#16690=CARTESIAN_POINT('Ctrl Pts',(-205.364578960846,-61.6047115119722,
5.66560329597973));
#16691=CARTESIAN_POINT('Ctrl Pts',(-208.051648633173,-63.4675697877938,
5.82451161478403));
#16692=CARTESIAN_POINT('Ctrl Pts',(-207.941000946252,-66.7353429545102,
5.98341993358834));
#16693=CARTESIAN_POINT('Ctrl Pts',(-205.134076462768,-68.4121730961013,
6.14232825239265));
#16694=CARTESIAN_POINT('Ctrl Pts',(-202.204232176763,-66.9607610803398,
6.30123657119695));
#16695=CARTESIAN_POINT('Ctrl Pts',(-201.837516583383,-63.7117452211441,
6.46014489000126));
#16696=CARTESIAN_POINT('Ctrl Pts',(-204.370130439934,-61.6437869446461,
6.61905320880556));
#16697=CARTESIAN_POINT('Ctrl Pts',(-207.480201669232,-62.6527672855972,
6.77796152760987));
#16698=CARTESIAN_POINT('Ctrl Pts',(-208.31645172888,-65.813664344578,6.93686984641418));
#16699=CARTESIAN_POINT('Ctrl Pts',(-206.112215910785,-68.2286030266078,
7.09577816521849));
#16700=CARTESIAN_POINT('Ctrl Pts',(-202.888312976691,-67.6835945392722,
7.25468648402279));
#16701=CARTESIAN_POINT('Ctrl Pts',(-201.600381103676,-64.678296572313,7.4135948028271));
#16702=CARTESIAN_POINT('Ctrl Pts',(-203.429181837975,-61.9679327122447,
7.5725031216314));
#16703=CARTESIAN_POINT('Ctrl Pts',(-206.698091106507,-62.0373342528012,
7.73141144043571));
#16704=CARTESIAN_POINT('Ctrl Pts',(-208.410209427808,-64.8228746372871,
7.89031975924003));
#16705=CARTESIAN_POINT('Ctrl Pts',(-206.995885860899,-67.7708015746146,
8.04922807804432));
#16706=CARTESIAN_POINT('Ctrl Pts',(-203.751756444322,-68.1784885970118,
8.20813639684863));
#16707=CARTESIAN_POINT('Ctrl Pts',(-201.65200276823,-65.6721727989785,8.36704471565294));
#16708=CARTESIAN_POINT('Ctrl Pts',(-202.621655534352,-62.5496164915781,
8.52595303445724));
#16709=CARTESIAN_POINT('Ctrl Pts',(-205.771747924315,-61.6735443972691,
8.68486135326156));
#16710=CARTESIAN_POINT('Ctrl Pts',(-208.214310442934,-63.8471296204372,
8.84376967206585));
#16711=CARTESIAN_POINT('Ctrl Pts',(-207.710029073154,-67.0776535221947,
9.00267799087017));
#16712=CARTESIAN_POINT('Ctrl Pts',(-204.721223338541,-68.4034078963079,
9.16158630967447));
#16713=CARTESIAN_POINT('Ctrl Pts',(-201.987996931325,-66.6089559502724,
9.32049462847878));
#16714=CARTESIAN_POINT('Ctrl Pts',(-202.016141272935,-63.3394311719952,
9.47940294728309));
#16715=CARTESIAN_POINT('Ctrl Pts',(-204.779853945546,-61.5922973353983,
9.63831126608739));
#16716=CARTESIAN_POINT('Ctrl Pts',(-207.745394060354,-62.9693072145201,
9.7972195848917));
#16717=CARTESIAN_POINT('Ctrl Pts',(-208.193987585331,-66.2080335427364,
9.95612790369601));
#16718=CARTESIAN_POINT('Ctrl Pts',(-205.714368990616,-68.3392482209132,
10.1150362225003));
#16719=CARTESIAN_POINT('Ctrl Pts',(-202.579824889659,-67.4090774522437,
10.2739445413046));
#16720=CARTESIAN_POINT('Ctrl Pts',(-201.664070280065,-64.2702914011178,
10.4328528601089));
#16721=CARTESIAN_POINT('Ctrl Pts',(-203.806658752712,-61.800494037645,10.5917611789132));
#16722=CARTESIAN_POINT('Ctrl Pts',(-207.043289143143,-62.2639679802425,
10.7506694977175));
#16723=CARTESIAN_POINT('Ctrl Pts',(-208.406654884562,-65.2358054984896,
10.9095778165218));
#16724=CARTESIAN_POINT('Ctrl Pts',(-206.646837503291,-67.9914591712706,
11.0684861353262));
#16725=CARTESIAN_POINT('Ctrl Pts',(-203.377217905366,-68.0045765107515,
11.2273944541305));
#16726=CARTESIAN_POINT('Ctrl Pts',(-201.595346794301,-65.2631316867057,
11.3863027729348));
#16727=CARTESIAN_POINT('Ctrl Pts',(-202.934823689116,-62.2804506732568,
11.5452110917391));
#16728=CARTESIAN_POINT('Ctrl Pts',(-206.167631143701,-61.7910220867251,
11.7041194105434));
#16729=CARTESIAN_POINT('Ctrl Pts',(-208.329967416112,-64.2435485850018,
11.8630277293477));
#16730=CARTESIAN_POINT('Ctrl Pts',(-207.43942677979,-67.3895812858467,12.021936048152));
#16731=CARTESIAN_POINT('Ctrl Pts',(-204.312446936723,-68.3448725716852,
12.1808443669563));
#16732=CARTESIAN_POINT('Ctrl Pts',(-201.815808057434,-66.233622068748,12.3397526857606));
#16733=CARTESIAN_POINT('Ctrl Pts',(-202.238400762026,-62.9914006411294,
12.4986610045649));
#16734=CARTESIAN_POINT('Ctrl Pts',(-205.192796782186,-61.5906406560071,
12.6575693233692));
#16735=CARTESIAN_POINT('Ctrl Pts',(-207.970438867253,-63.3155432117869,
12.8164776421735));
#16736=CARTESIAN_POINT('Ctrl Pts',(-208.024815798874,-66.5847369241054,
12.9753859609778));
#16737=CARTESIAN_POINT('Ctrl Pts',(-205.306075413683,-68.4010615368247,
13.1342942797821));
#16738=CARTESIAN_POINT('Ctrl Pts',(-202.306728510468,-67.099330945249,13.2932025985865));
#16739=CARTESIAN_POINT('Ctrl Pts',(-201.776542806102,-63.8729572074659,
13.4521109173907));
#16740=CARTESIAN_POINT('Ctrl Pts',(-204.201586630452,-61.6798437039,13.6110192361951));
#16741=CARTESIAN_POINT('Ctrl Pts',(-207.3586069057,-62.5306123864796,13.7699275549994));
#16742=CARTESIAN_POINT('Ctrl Pts',(-208.353282736821,-65.6452880279853,
13.9288358738037));
#16743=CARTESIAN_POINT('Ctrl Pts',(-206.273706422742,-68.1683708286262,
14.087744192608));
#16744=CARTESIAN_POINT('Ctrl Pts',(-203.026410318955,-67.7867266432836,
14.2466525114123));
#16745=CARTESIAN_POINT('Ctrl Pts',(-201.588479129595,-64.8502426644178,
14.4055608302166));
#16746=CARTESIAN_POINT('Ctrl Pts',(-203.278192240605,-62.0510544415413,
14.5644691490209));
#16747=CARTESIAN_POINT('Ctrl Pts',(-206.546439262996,-61.9554267434409,
14.7233774678252));
#16748=CARTESIAN_POINT('Ctrl Pts',(-208.396928461221,-64.6510293737779,
14.8822857866295));
#16749=CARTESIAN_POINT('Ctrl Pts',(-207.133150773185,-67.6665652068362,
15.0411941054338));
#16750=CARTESIAN_POINT('Ctrl Pts',(-203.913726026938,-68.2374221470678,
15.2001024242381));
#16751=CARTESIAN_POINT('Ctrl Pts',(-201.690181558921,-65.8402501772315,
15.3590107430424));
#16752=CARTESIAN_POINT('Ctrl Pts',(-202.501048971901,-62.6727389682273,
15.5179190618468));
#16753=CARTESIAN_POINT('Ctrl Pts',(-205.602911672279,-61.638849624479,15.676827380651));
#16754=CARTESIAN_POINT('Ctrl Pts',(-208.15206274551,-63.6863945744461,15.8357356994554));
#16755=CARTESIAN_POINT('Ctrl Pts',(-207.811373989716,-66.9383017123736,
15.9946440182597));
#16756=CARTESIAN_POINT('Ctrl Pts',(-204.893380603372,-68.4130649498665,
16.153552337064));
#16757=CARTESIAN_POINT('Ctrl Pts',(-202.07286371831,-66.7590371605543,16.3124606558683));
#16758=CARTESIAN_POINT('Ctrl Pts',(-201.936470506822,-63.4917903773687,
16.4713689746726));
#16759=CARTESIAN_POINT('Ctrl Pts',(-204.607538235084,-61.608392321744,16.6302772934769));
#16760=CARTESIAN_POINT('Ctrl Pts',(-207.64077536484,-62.8320207279313,16.7891856122812));
#16761=CARTESIAN_POINT('Ctrl Pts',(-208.24805155724,-66.0480436019276,16.9480939310855));
#16762=CARTESIAN_POINT('Ctrl Pts',(-206.674550837501,-67.5419185807874,
17.0540328102884));
#16763=CARTESIAN_POINT('Ctrl Pts',(-205.745932854347,-67.7901775698422,
17.1070022498898));
#16764=CARTESIAN_POINT('Ctrl Pts',(-207.336062657696,-63.0026984430693,
-0.321006749669434));
#16765=CARTESIAN_POINT('Ctrl Pts',(-208.000798179763,-63.7801793522269,
-0.268037310067998));
#16766=CARTESIAN_POINT('Ctrl Pts',(-208.480240995509,-66.0387750109567,
-0.162098430865127));
#16767=CARTESIAN_POINT('Ctrl Pts',(-206.009082789328,-68.4931171380248,
-0.00319011206082034));
#16768=CARTESIAN_POINT('Ctrl Pts',(-202.611389949013,-67.7378152625506,
0.155718206743486));
#16769=CARTESIAN_POINT('Ctrl Pts',(-201.404198517164,-64.4760115003611,
0.314626525547793));
#16770=CARTESIAN_POINT('Ctrl Pts',(-203.493276918295,-61.6929032503864,
0.473534844352099));
#16771=CARTESIAN_POINT('Ctrl Pts',(-206.963857847912,-61.9425259124891,
0.632443163156407));
#16772=CARTESIAN_POINT('Ctrl Pts',(-208.633920228955,-64.9948075983619,
0.791351481960713));
#16773=CARTESIAN_POINT('Ctrl Pts',(-206.972481892344,-68.0520434541846,
0.950259800765019));
#16774=CARTESIAN_POINT('Ctrl Pts',(-203.502676360176,-68.3111058299649,
1.10916811956933));
#16775=CARTESIAN_POINT('Ctrl Pts',(-201.405609072658,-65.5346291225997,
1.26807643837363));
#16776=CARTESIAN_POINT('Ctrl Pts',(-202.603835003667,-62.2679881960402,
1.42698475717794));
#16777=CARTESIAN_POINT('Ctrl Pts',(-205.998840266797,-61.5060359469962,
1.58589307598225));
#16778=CARTESIAN_POINT('Ctrl Pts',(-208.478118943853,-63.9473056488985,
1.74480139478655));
#16779=CARTESIAN_POINT('Ctrl Pts',(-207.768697529891,-67.3536763121769,
1.90370971359086));
#16780=CARTESIAN_POINT('Ctrl Pts',(-204.52096493132,-68.6022216022895,2.06261803239517));
#16781=CARTESIAN_POINT('Ctrl Pts',(-201.712406443479,-66.548290989434,2.22152635119947));
#16782=CARTESIAN_POINT('Ctrl Pts',(-201.917876928207,-63.0749042105964,
2.38043467000378));
#16783=CARTESIAN_POINT('Ctrl Pts',(-204.949003423762,-61.3664238768246,
2.53934298880808));
#16784=CARTESIAN_POINT('Ctrl Pts',(-208.026882997387,-62.9891654522027,
2.69825130761239));
#16785=CARTESIAN_POINT('Ctrl Pts',(-208.329750076191,-66.455417699762,2.8571596264167));
#16786=CARTESIAN_POINT('Ctrl Pts',(-205.579939497992,-68.5873592508376,
3.01606794522101));
#16787=CARTESIAN_POINT('Ctrl Pts',(-202.298446871394,-67.4304499438088,
3.17497626402531));
#16788=CARTESIAN_POINT('Ctrl Pts',(-201.493707957674,-64.0453312890996,
3.33388458282962));
#16789=CARTESIAN_POINT('Ctrl Pts',(-203.90349839961,-61.5354422402711,3.49279290163393));
#16790=CARTESIAN_POINT('Ctrl Pts',(-207.318549253241,-62.2018210220118,
3.65170122043824));
#16791=CARTESIAN_POINT('Ctrl Pts',(-208.607980065528,-65.4335390165435,
3.81060953924254));
#16792=CARTESIAN_POINT('Ctrl Pts',(-206.589655079347,-68.2677932860708,
3.96951785804685));
#16793=CARTESIAN_POINT('Ctrl Pts',(-203.113952083686,-68.1061711944818,
4.12842617685116));
#16794=CARTESIAN_POINT('Ctrl Pts',(-201.367356737724,-65.096846068775,4.28733449565546));
#16795=CARTESIAN_POINT('Ctrl Pts',(-202.951128133319,-61.9987335496681,
4.44624281445977));
#16796=CARTESIAN_POINT('Ctrl Pts',(-206.413282356468,-61.652148567679,4.60515113326408));
#16797=CARTESIAN_POINT('Ctrl Pts',(-208.579755111172,-64.3748363606043,
4.76405945206838));
#16798=CARTESIAN_POINT('Ctrl Pts',(-207.464348390136,-67.6706671908,4.92296777087269));
#16799=CARTESIAN_POINT('Ctrl Pts',(-204.089654608536,-68.5180601899667,
5.08187608967699));
#16800=CARTESIAN_POINT('Ctrl Pts',(-201.549555307088,-66.1401349276025,
5.2407844084813));
#16801=CARTESIAN_POINT('Ctrl Pts',(-202.172785135194,-62.7169467066651,
5.39969272728561));
#16802=CARTESIAN_POINT('Ctrl Pts',(-205.387973952159,-61.3868362278423,
5.55860104608991));
#16803=CARTESIAN_POINT('Ctrl Pts',(-208.247472586089,-63.3692339117493,
5.71750936489423));
#16804=CARTESIAN_POINT('Ctrl Pts',(-208.129724649422,-66.8466997186291,
5.87641768369853));
#16805=CARTESIAN_POINT('Ctrl Pts',(-205.142680134451,-68.6311318636507,
6.03532600250283));
#16806=CARTESIAN_POINT('Ctrl Pts',(-202.024828066921,-67.0865829004874,
6.19423432130715));
#16807=CARTESIAN_POINT('Ctrl Pts',(-201.634580374757,-63.629078055463,6.35314264011145));
#16808=CARTESIAN_POINT('Ctrl Pts',(-204.329711780416,-61.428419126679,6.51205095891576));
#16809=CARTESIAN_POINT('Ctrl Pts',(-207.639355934117,-62.5021456237346,
6.67095927772006));
#16810=CARTESIAN_POINT('Ctrl Pts',(-208.529268066955,-65.8658770949486,
6.82986759652438));
#16811=CARTESIAN_POINT('Ctrl Pts',(-206.183586681908,-68.4357821232429,
6.98877591532867));
#16812=CARTESIAN_POINT('Ctrl Pts',(-202.752806255592,-67.8558005019746,
7.14768423413299));
#16813=CARTESIAN_POINT('Ctrl Pts',(-201.382227937729,-64.6576528991878,
7.30659255293729));
#16814=CARTESIAN_POINT('Ctrl Pts',(-203.328382611466,-61.7733652920829,
7.4655008717416));
#16815=CARTESIAN_POINT('Ctrl Pts',(-206.807057423689,-61.8472203217673,
7.6244091905459));
#16816=CARTESIAN_POINT('Ctrl Pts',(-208.629042186982,-64.811508522489,7.78331750935021));
#16817=CARTESIAN_POINT('Ctrl Pts',(-207.123961634304,-67.9486036030623,
7.94222582815452));
#16818=CARTESIAN_POINT('Ctrl Pts',(-203.671656794376,-68.3824518562811,
8.10113414695882));
#16819=CARTESIAN_POINT('Ctrl Pts',(-201.437162158747,-65.7153060526264,
8.26004246576313));
#16820=CARTESIAN_POINT('Ctrl Pts',(-202.469037434877,-62.3923756547517,
8.41895078456743));
#16821=CARTESIAN_POINT('Ctrl Pts',(-205.821270902666,-61.4600861117225,
8.57785910337174));
#16822=CARTESIAN_POINT('Ctrl Pts',(-208.420572386066,-63.7731500565804,
8.73676742217605));
#16823=CARTESIAN_POINT('Ctrl Pts',(-207.883931336951,-67.2109763173173,
8.89567574098036));
#16824=CARTESIAN_POINT('Ctrl Pts',(-204.703334271224,-68.6218042019629,
9.05458405978466));
#16825=CARTESIAN_POINT('Ctrl Pts',(-201.794717029867,-66.7122024744056,
9.21349237858897));
#16826=CARTESIAN_POINT('Ctrl Pts',(-201.824667390743,-63.2328726552463,
9.37240069739327));
#16827=CARTESIAN_POINT('Ctrl Pts',(-204.76572719775,-61.3736254349403,9.53130901619758));
#16828=CARTESIAN_POINT('Ctrl Pts',(-207.921565691441,-62.8389978846421,
9.69021733500189));
#16829=CARTESIAN_POINT('Ctrl Pts',(-208.398945412955,-66.2855529206304,
9.8491256538062));
#16830=CARTESIAN_POINT('Ctrl Pts',(-205.760209969182,-68.5535274073437,
10.0080339726105));
#16831=CARTESIAN_POINT('Ctrl Pts',(-202.424522522372,-67.5636676840456,
10.1669422914148));
#16832=CARTESIAN_POINT('Ctrl Pts',(-201.450004041473,-64.2234660815981,
10.3258506102191));
#16833=CARTESIAN_POINT('Ctrl Pts',(-203.73008217778,-61.5951820963824,10.4847589290234));
#16834=CARTESIAN_POINT('Ctrl Pts',(-207.17440677989,-62.0883971102576,10.6436672478277));
#16835=CARTESIAN_POINT('Ctrl Pts',(-208.625259549091,-65.2509371110651,
10.802575566632));
#16836=CARTESIAN_POINT('Ctrl Pts',(-206.752514882462,-68.1834207731203,
10.9614838854363));
#16837=CARTESIAN_POINT('Ctrl Pts',(-203.273084159089,-68.1973798508147,
11.1203922042406));
#16838=CARTESIAN_POINT('Ctrl Pts',(-201.376870577281,-65.2800168177356,
11.279300523045));
#16839=CARTESIAN_POINT('Ctrl Pts',(-202.802301555254,-62.1059374958468,
11.4382088418493));
#16840=CARTESIAN_POINT('Ctrl Pts',(-206.242557904149,-61.585102331427,11.5971171606536));
#16841=CARTESIAN_POINT('Ctrl Pts',(-208.543651054332,-64.1950071819504,
11.7560254794579));
#16842=CARTESIAN_POINT('Ctrl Pts',(-207.59596452456,-67.5429204508222,11.9149337982622));
#16843=CARTESIAN_POINT('Ctrl Pts',(-204.268326733228,-68.5595126720785,
12.0738421170665));
#16844=CARTESIAN_POINT('Ctrl Pts',(-201.611478815115,-66.3127834595062,
12.2327504358708));
#16845=CARTESIAN_POINT('Ctrl Pts',(-202.061189246496,-62.8625090439764,
12.3916587546751));
#16846=CARTESIAN_POINT('Ctrl Pts',(-205.205168530226,-61.3718624466171,
12.5505670734794));
#16847=CARTESIAN_POINT('Ctrl Pts',(-208.161051598535,-63.2074518072919,
12.7094753922837));
#16848=CARTESIAN_POINT('Ctrl Pts',(-208.218917891802,-66.6864293160267,
12.868383711088));
#16849=CARTESIAN_POINT('Ctrl Pts',(-205.32571623889,-68.6193072768529,13.0272920298923));
#16850=CARTESIAN_POINT('Ctrl Pts',(-202.133901578945,-67.2340447781946,
13.1862003486966));
#16851=CARTESIAN_POINT('Ctrl Pts',(-201.569693916979,-63.8006349969923,
13.3451086675009));
#16852=CARTESIAN_POINT('Ctrl Pts',(-204.150352533451,-61.4667896441583,
13.5040169863052));
#16853=CARTESIAN_POINT('Ctrl Pts',(-207.509958448151,-62.3721520583455,
13.6629253051096));
#16854=CARTESIAN_POINT('Ctrl Pts',(-208.568462516575,-65.6866960888727,
13.8218336239139));
#16855=CARTESIAN_POINT('Ctrl Pts',(-206.355440022032,-68.371684831825,13.9807419427182));
#16856=CARTESIAN_POINT('Ctrl Pts',(-202.89976528893,-67.9655505816142,14.1396502615225));
#16857=CARTESIAN_POINT('Ctrl Pts',(-201.369562215296,-64.8406327528726,
14.2985585803268));
#16858=CARTESIAN_POINT('Ctrl Pts',(-203.167704028449,-61.8618209334909,
14.4574668991311));
#16859=CARTESIAN_POINT('Ctrl Pts',(-206.64567409827,-61.7600568166538,14.6163752179354));
#16860=CARTESIAN_POINT('Ctrl Pts',(-208.614908982248,-64.6286359675596,
14.7752835367397));
#16861=CARTESIAN_POINT('Ctrl Pts',(-207.270034820723,-67.8376783991727,
14.934191855544));
#16862=CARTESIAN_POINT('Ctrl Pts',(-203.844019947069,-68.4451671656806,
15.0931001743483));
#16863=CARTESIAN_POINT('Ctrl Pts',(-201.477790878185,-65.8941689375223,
15.2520084931526));
#16864=CARTESIAN_POINT('Ctrl Pts',(-202.340691562746,-62.5233988870148,
15.4109168119569));
#16865=CARTESIAN_POINT('Ctrl Pts',(-205.641600447141,-61.4231649792265,
15.5698251307612));
#16866=CARTESIAN_POINT('Ctrl Pts',(-208.354330260832,-63.6021006605898,
15.7287334495655));
#16867=CARTESIAN_POINT('Ctrl Pts',(-207.991779545523,-67.0626823173804,
15.8876417683699));
#16868=CARTESIAN_POINT('Ctrl Pts',(-204.886538848565,-68.6320809475727,
16.0465500871742));
#16869=CARTESIAN_POINT('Ctrl Pts',(-201.885029709121,-66.8719143792362,
16.2054584059785));
#16870=CARTESIAN_POINT('Ctrl Pts',(-201.739884160442,-63.3950087338597,
16.3643667247828));
#16871=CARTESIAN_POINT('Ctrl Pts',(-204.58235400734,-61.3907532347673,16.5232750435871));
#16872=CARTESIAN_POINT('Ctrl Pts',(-207.810233625888,-62.6929017394991,
16.6821833623914));
#16873=CARTESIAN_POINT('Ctrl Pts',(-208.45647866392,-66.1152964431386,16.8410916811957));
#16874=CARTESIAN_POINT('Ctrl Pts',(-206.782006578242,-67.7050332130129,
16.9470305603986));
#16875=CARTESIAN_POINT('Ctrl Pts',(-205.793799282533,-67.9692229537457,
17.));
#16876=CARTESIAN_POINT('Ctrl Pts',(-206.913465996665,-63.364012796625,-1.94289029309402E-15));
#16877=CARTESIAN_POINT('Ctrl Pts',(-206.975064335153,-63.4219001091858,
-1.97292133004108E-15));
#16878=CARTESIAN_POINT('Ctrl Pts',(-207.033290434855,-63.482938938711,-2.21623739315488E-15));
#16879=CARTESIAN_POINT('Ctrl Pts',(-207.088148006259,-63.5467442557774,
-2.20309881449055E-15));
#16880=CARTESIAN_POINT('Ctrl Pts',(-207.14445943011,-63.6122405612339,-2.1896120331214E-15));
#16881=CARTESIAN_POINT('Ctrl Pts',(-207.197221846936,-63.6806523656421,
-1.80211485911159E-15));
#16882=CARTESIAN_POINT('Ctrl Pts',(-207.246413701517,-63.7516117614939,
-1.6306400674182E-15));
#16883=CARTESIAN_POINT('Ctrl Pts',(-207.29736402947,-63.8251077603907,-1.45303552400534E-15));
#16884=CARTESIAN_POINT('Ctrl Pts',(-207.344484547899,-63.9013372602885,
-2.27663609778748E-15));
#16885=CARTESIAN_POINT('Ctrl Pts',(-207.387716218901,-63.9799356548756,
-2.32452945780892E-15));
#16886=CARTESIAN_POINT('Ctrl Pts',(-207.406630074965,-64.0143224525075,
-2.3454828028183E-15));
#16887=CARTESIAN_POINT('Ctrl Pts',(-207.424799084886,-64.0491631801201,
-2.03082216487457E-15));
#16888=CARTESIAN_POINT('Ctrl Pts',(-207.442215847947,-64.084429403981,-2.04697370165263E-15));
#16889=CARTESIAN_POINT('Ctrl Pts',(-207.4516722521,-64.1035771448449,-2.05574315318221E-15));
#16890=CARTESIAN_POINT('Ctrl Pts',(-207.460906871958,-64.1228503386334,
-2.04057437215808E-15));
#16891=CARTESIAN_POINT('Ctrl Pts',(-207.469918322462,-64.1422445609559,
-2.04697370165263E-15));
#16892=CARTESIAN_POINT('Ctrl Pts',(-207.478568225495,-64.1608606696942,
-2.05311628431163E-15));
#16893=CARTESIAN_POINT('Ctrl Pts',(-207.487014999459,-64.1795942961117,
-2.37355651913976E-15));
#16894=CARTESIAN_POINT('Ctrl Pts',(-207.495243316265,-64.1984087222124,
-2.34534613952064E-15));
#16895=CARTESIAN_POINT('Ctrl Pts',(-207.531786155502,-64.281965610518,-2.22006081185391E-15));
#16896=CARTESIAN_POINT('Ctrl Pts',(-207.564069529394,-64.3672061702463,
-2.19854429085911E-15));
#16897=CARTESIAN_POINT('Ctrl Pts',(-207.592069829017,-64.4537311766029,
-2.15105711021124E-15));
#16898=CARTESIAN_POINT('Ctrl Pts',(-207.620534398179,-64.5416908434951,
-2.10278255043571E-15));
#16899=CARTESIAN_POINT('Ctrl Pts',(-207.644573172372,-64.6309786604899,
-2.09454222238891E-15));
#16900=CARTESIAN_POINT('Ctrl Pts',(-207.664122231294,-64.7212123541091,
-2.12330153459561E-15));
#16901=CARTESIAN_POINT('Ctrl Pts',(-207.68337365362,-64.8100722297138,-2.15162298307744E-15));
#16902=CARTESIAN_POINT('Ctrl Pts',(-207.698271307414,-64.8998503076178,
-2.67974986921836E-15));
#16903=CARTESIAN_POINT('Ctrl Pts',(-207.708711137774,-64.9902045182676,
-2.76167977375508E-15));
#16904=CARTESIAN_POINT('Ctrl Pts',(-207.712805437947,-65.0256396975281,
-2.79381110259042E-15));
#16905=CARTESIAN_POINT('Ctrl Pts',(-207.716213605543,-65.0611636688123,
-2.0404376105344E-15));
#16906=CARTESIAN_POINT('Ctrl Pts',(-207.718927373463,-65.0967563226444,
-2.02615701994091E-15));
#16907=CARTESIAN_POINT('Ctrl Pts',(-207.720523200181,-65.1176865236056,
-2.01775934236463E-15));
#16908=CARTESIAN_POINT('Ctrl Pts',(-207.721878881011,-65.1386404789908,
-1.74090680682343E-15));
#16909=CARTESIAN_POINT('Ctrl Pts',(-207.72299254181,-65.1596141213673,-1.72084568816899E-15));
#16910=CARTESIAN_POINT('Ctrl Pts',(-207.723754218348,-65.1739588224918,
-1.70712509800373E-15));
#16911=CARTESIAN_POINT('Ctrl Pts',(-207.724402620351,-65.1883131146187,
-1.95724670614016E-15));
#16912=CARTESIAN_POINT('Ctrl Pts',(-207.724936762549,-65.2026603377787,
-1.95676808090184E-15));
#16913=CARTESIAN_POINT('Ctrl Pts',(-207.728480618606,-65.2978493977624,
-1.95359256142936E-15));
#16914=CARTESIAN_POINT('Ctrl Pts',(-207.727008196039,-65.3928884344764,
-1.81199077416004E-15));
#16915=CARTESIAN_POINT('Ctrl Pts',(-207.720461583985,-65.4873781558944,
-1.85962356624714E-15));
#16916=CARTESIAN_POINT('Ctrl Pts',(-207.713936993971,-65.5815500248844,
-1.9070961271642E-15));
#16917=CARTESIAN_POINT('Ctrl Pts',(-207.702372653513,-65.6751772225213,
-2.05958830061839E-15));
#16918=CARTESIAN_POINT('Ctrl Pts',(-207.685663242701,-65.767882393997,-1.99840144432528E-15));
#16919=CARTESIAN_POINT('Ctrl Pts',(-207.683580478217,-65.7794377409136,
-1.99077473548103E-15));
#16920=CARTESIAN_POINT('Ctrl Pts',(-207.681417710998,-65.7909787747085,
-2.33792174055657E-15));
#16921=CARTESIAN_POINT('Ctrl Pts',(-207.679174680234,-65.8025047726911,
-2.35922392732846E-15));
#16922=CARTESIAN_POINT('Ctrl Pts',(-207.661554445533,-65.8930477972969,
-2.52759723237176E-15));
#16923=CARTESIAN_POINT('Ctrl Pts',(-207.638985550185,-65.9826632848584,
-1.79135627445481E-15));
#16924=CARTESIAN_POINT('Ctrl Pts',(-207.611743048214,-66.0711138579085,
-1.66533453693773E-15));
#16925=CARTESIAN_POINT('Ctrl Pts',(-207.60081644828,-66.1065901892194,-1.61478891853904E-15));
#16926=CARTESIAN_POINT('Ctrl Pts',(-207.589137410261,-66.1418790674857,
-1.79168624825887E-15));
#16927=CARTESIAN_POINT('Ctrl Pts',(-207.576721387245,-66.1769648121992,
-1.77635683940025E-15));
#16928=CARTESIAN_POINT('Ctrl Pts',(-207.570942246212,-66.1932957634797,
-1.76922163872903E-15));
#16929=CARTESIAN_POINT('Ctrl Pts',(-207.565003418531,-66.2095827012965,
-1.91957011249023E-15));
#16930=CARTESIAN_POINT('Ctrl Pts',(-207.558906371455,-66.2258240187521,
-1.9151347174784E-15));
#16931=CARTESIAN_POINT('Ctrl Pts',(-207.553840425172,-66.2393186893321,
-1.91144941333107E-15));
#16932=CARTESIAN_POINT('Ctrl Pts',(-207.548668567227,-66.2527729916654,
-2.42723306653759E-15));
#16933=CARTESIAN_POINT('Ctrl Pts',(-207.543392857624,-66.2661841275907,
-2.41473507855972E-15));
#16934=CARTESIAN_POINT('Ctrl Pts',(-207.509159374317,-66.3532074727684,
-2.33363704720111E-15));
#16935=CARTESIAN_POINT('Ctrl Pts',(-207.470547395912,-66.4384398905487,
-2.12854475574276E-15));
#16936=CARTESIAN_POINT('Ctrl Pts',(-207.427889442439,-66.5216501935512,
-2.16493489801906E-15));
#16937=CARTESIAN_POINT('Ctrl Pts',(-207.38365247829,-66.6079405776665,-2.20267204404216E-15));
#16938=CARTESIAN_POINT('Ctrl Pts',(-207.335064336909,-66.692057101939,-2.12399586674231E-15));
#16939=CARTESIAN_POINT('Ctrl Pts',(-207.282439886309,-66.773738360666,-2.05391259555654E-15));
#16940=CARTESIAN_POINT('Ctrl Pts',(-207.229239181682,-66.8563140544646,
-1.98306189085347E-15));
#16941=CARTESIAN_POINT('Ctrl Pts',(-207.171912867569,-66.9364016733955,
-1.93693493431011E-15));
#16942=CARTESIAN_POINT('Ctrl Pts',(-207.110734661138,-67.0137157330808,
-1.9151347174784E-15));
#16943=CARTESIAN_POINT('Ctrl Pts',(-207.086644405525,-67.0441598335049,
-1.90655040573494E-15));
#16944=CARTESIAN_POINT('Ctrl Pts',(-207.061956365489,-67.0741736421049,
-2.23389407293862E-15));
#16945=CARTESIAN_POINT('Ctrl Pts',(-207.036685317581,-67.1037386472167,
-2.27595720048157E-15));
#16946=CARTESIAN_POINT('Ctrl Pts',(-207.022376522802,-67.1204787362049,
-2.29977388833693E-15));
#16947=CARTESIAN_POINT('Ctrl Pts',(-207.007880798569,-67.1370749273764,
-2.22822292691737E-15));
#16948=CARTESIAN_POINT('Ctrl Pts',(-206.993200685982,-67.1535237511539,
-2.22044604925031E-15));
#16949=CARTESIAN_POINT('Ctrl Pts',(-206.979145852523,-67.1692719599935,
-2.21300041694992E-15));
#16950=CARTESIAN_POINT('Ctrl Pts',(-206.964919138242,-67.1848880123012,
-1.95342784401499E-15));
#16951=CARTESIAN_POINT('Ctrl Pts',(-206.950541882912,-67.2003486168303,
-1.97064586870965E-15));
#16952=CARTESIAN_POINT('Ctrl Pts',(-206.881822930974,-67.2742456517767,
-2.05294284294357E-15));
#16953=CARTESIAN_POINT('Ctrl Pts',(-206.809592725806,-67.3446809429097,
-2.39171272535874E-15));
#16954=CARTESIAN_POINT('Ctrl Pts',(-206.734164841959,-67.4113677334851,
-2.22044604925031E-15));
#16955=CARTESIAN_POINT('Ctrl Pts',(-206.66904943858,-67.4689371235679,-2.07259490811688E-15));
#16956=CARTESIAN_POINT('Ctrl Pts',(-206.6015499159,-67.5237130159225,-1.84853531005696E-15));
#16957=CARTESIAN_POINT('Ctrl Pts',(-206.531841458199,-67.5754953714549,
-1.72084568816899E-15));
#16958=CARTESIAN_POINT('Ctrl Pts',(-206.504681281771,-67.595671085543,-1.67109458517742E-15));
#16959=CARTESIAN_POINT('Ctrl Pts',(-206.477185531439,-67.6153921679212,
-1.55730478202358E-15));
#16960=CARTESIAN_POINT('Ctrl Pts',(-206.449363702133,-67.6346459831098,
-1.55431223447522E-15));
#16961=CARTESIAN_POINT('Ctrl Pts',(-206.43409331051,-67.6452137029715,-1.55266973381473E-15));
#16962=CARTESIAN_POINT('Ctrl Pts',(-206.418725944916,-67.6556396822825,
-1.84911424756666E-15));
#16963=CARTESIAN_POINT('Ctrl Pts',(-206.403273354045,-67.6659153349133,
-1.83186799063151E-15));
#16964=CARTESIAN_POINT('Ctrl Pts',(-206.316688603458,-67.7234923993424,
-1.73523287825519E-15));
#16965=CARTESIAN_POINT('Ctrl Pts',(-206.227347132085,-67.7764114036352,
-1.8361507155124E-15));
#16966=CARTESIAN_POINT('Ctrl Pts',(-206.135558921451,-67.8243493290082,
-1.33226762955019E-15));
#16967=CARTESIAN_POINT('Ctrl Pts',(-206.043770710818,-67.8722872543811,
-8.28384543587972E-16));
#16968=CARTESIAN_POINT('Ctrl Pts',(-205.949535108699,-67.915245019694,-3.68147691493984E-16));
#16969=CARTESIAN_POINT('Ctrl Pts',(-205.853123870327,-67.9528583595717,
-2.22044604925031E-16));
#16970=CARTESIAN_POINT('Ctrl Pts',(-205.834023285542,-67.9603101546064,
-1.93099282372341E-16));
#16971=CARTESIAN_POINT('Ctrl Pts',(-205.814837205121,-67.9675520267903,
-1.66533453693773E-16));
#16972=CARTESIAN_POINT('Ctrl Pts',(-205.795568749511,-67.9745849194645,
-1.66533453693773E-16));
#16973=CARTESIAN_POINT('Ctrl Pts',(-202.480291602729,-65.0019224916823,
1.61258330249198));
#16974=CARTESIAN_POINT('Ctrl Pts',(-202.47924620393,-65.1255297484548,1.60474993100901));
#16975=CARTESIAN_POINT('Ctrl Pts',(-202.487554213272,-65.248995872321,1.59691655952604));
#16976=CARTESIAN_POINT('Ctrl Pts',(-202.505700651816,-65.3709985616315,
1.58908318804307));
#16977=CARTESIAN_POINT('Ctrl Pts',(-202.628407290015,-66.1959835756441,
1.53611374844163));
#16978=CARTESIAN_POINT('Ctrl Pts',(-203.200975686124,-66.9540531066665,
1.48314430884019));
#16979=CARTESIAN_POINT('Ctrl Pts',(-203.960945445007,-67.2977215942629,
1.43017486923876));
#16980=CARTESIAN_POINT('Ctrl Pts',(-204.72091520389,-67.6413900818592,1.37720542963732));
#16981=CARTESIAN_POINT('Ctrl Pts',(-205.668286325546,-67.5706575260295,
1.32423599003589));
#16982=CARTESIAN_POINT('Ctrl Pts',(-206.368785563095,-67.1179282381352,
1.27126655043445));
#16983=CARTESIAN_POINT('Ctrl Pts',(-207.069284800645,-66.6651989502408,
1.21829711083302));
#16984=CARTESIAN_POINT('Ctrl Pts',(-207.522912154087,-65.8304729302817,
1.16532767123158));
#16985=CARTESIAN_POINT('Ctrl Pts',(-207.521734830089,-64.9964232360559,
1.11235823163015));
#16986=CARTESIAN_POINT('Ctrl Pts',(-207.52055750609,-64.1623735418301,1.05938879202871));
#16987=CARTESIAN_POINT('Ctrl Pts',(-207.064575504651,-63.3290001733376,
1.00641935242727));
#16988=CARTESIAN_POINT('Ctrl Pts',(-206.362793088589,-62.8782358874513,
0.953449912825839));
#16989=CARTESIAN_POINT('Ctrl Pts',(-205.661010672528,-62.427471601565,0.900480473224403));
#16990=CARTESIAN_POINT('Ctrl Pts',(-204.713427841845,-62.359316398285,0.847511033622967));
#16991=CARTESIAN_POINT('Ctrl Pts',(-203.954442842921,-62.7051788768636,
0.794541594021531));
#16992=CARTESIAN_POINT('Ctrl Pts',(-203.195457843997,-63.0510413554422,
0.741572154420096));
#16993=CARTESIAN_POINT('Ctrl Pts',(-202.625070676832,-63.8109215158794,
0.68860271481866));
#16994=CARTESIAN_POINT('Ctrl Pts',(-202.504678591524,-64.6361514920533,
0.635633275217225));
#16995=CARTESIAN_POINT('Ctrl Pts',(-202.487215476291,-64.7558527675182,
0.627949950975476));
#16996=CARTESIAN_POINT('Ctrl Pts',(-202.47922029748,-64.8769290089006,0.620266626733727));
#16997=CARTESIAN_POINT('Ctrl Pts',(-202.480232352617,-64.9981364767374,
0.612583302491977));
#16998=CARTESIAN_POINT('Ctrl Pts',(-204.206200717467,-67.9692229537457,
-8.32667268468867E-16));
#16999=CARTESIAN_POINT('Ctrl Pts',(-203.217993421758,-67.705033213013,0.0529694396014348));
#17000=CARTESIAN_POINT('Ctrl Pts',(-201.543521285756,-66.115296794048,0.158908318804306));
#17001=CARTESIAN_POINT('Ctrl Pts',(-202.189766417583,-62.6929016513152,
0.317816637608613));
#17002=CARTESIAN_POINT('Ctrl Pts',(-205.417645988708,-61.3907533400893,
0.47672495641292));
#17003=CARTESIAN_POINT('Ctrl Pts',(-208.260115801475,-63.3950087136501,
0.635633275217226));
#17004=CARTESIAN_POINT('Ctrl Pts',(-208.114970263096,-66.8719143799143,
0.794541594021533));
#17005=CARTESIAN_POINT('Ctrl Pts',(-205.113461147179,-68.6320808995075,
0.95344991282584));
#17006=CARTESIAN_POINT('Ctrl Pts',(-202.008220487258,-67.0626823018313,
1.11235823163015));
#17007=CARTESIAN_POINT('Ctrl Pts',(-201.645669772482,-63.602100671981,1.27126655043445));
#17008=CARTESIAN_POINT('Ctrl Pts',(-204.358399560164,-61.4231650176065,
1.43017486923876));
#17009=CARTESIAN_POINT('Ctrl Pts',(-207.659308409489,-62.5233989116837,
1.58908318804307));
#17010=CARTESIAN_POINT('Ctrl Pts',(-208.522209085787,-65.8941689287448,
1.74799150684737));
#17011=CARTESIAN_POINT('Ctrl Pts',(-206.155980040914,-68.445167130006,1.90689982565168));
#17012=CARTESIAN_POINT('Ctrl Pts',(-202.729965202703,-67.8376783700826,
2.06580814445599));
#17013=CARTESIAN_POINT('Ctrl Pts',(-201.385091054919,-64.6286359713235,
2.22471646326029));
#17014=CARTESIAN_POINT('Ctrl Pts',(-203.354325918685,-61.7600568500266,
2.3836247820646));
#17015=CARTESIAN_POINT('Ctrl Pts',(-206.832295952684,-61.8618209657714,
2.54253310086891));
#17016=CARTESIAN_POINT('Ctrl Pts',(-208.630437747347,-64.8406327545204,
2.70144141967322));
#17017=CARTESIAN_POINT('Ctrl Pts',(-207.100234689454,-67.965550551091,2.86034973847752));
#17018=CARTESIAN_POINT('Ctrl Pts',(-203.644559991919,-68.3716847971282,
3.01925805728183));
#17019=CARTESIAN_POINT('Ctrl Pts',(-201.431537520148,-65.6866960818049,
3.17816637608613));
#17020=CARTESIAN_POINT('Ctrl Pts',(-202.49004157768,-62.3721520853899,3.33707469489044));
#17021=CARTESIAN_POINT('Ctrl Pts',(-205.849647457805,-61.4667896805192,
3.49598301369474));
#17022=CARTESIAN_POINT('Ctrl Pts',(-208.430306047719,-63.8006350093353,
3.65489133249905));
#17023=CARTESIAN_POINT('Ctrl Pts',(-207.86609839156,-67.2340447552034,3.81379965130336));
#17024=CARTESIAN_POINT('Ctrl Pts',(-204.674283764462,-68.6193072396057,
3.97270797010767));
#17025=CARTESIAN_POINT('Ctrl Pts',(-201.781082141325,-66.6864292986713,
4.13161628891197));
#17026=CARTESIAN_POINT('Ctrl Pts',(-201.838948433996,-63.2074518257396,
4.29052460771628));
#17027=CARTESIAN_POINT('Ctrl Pts',(-204.794831471885,-61.3718624839552,
4.44943292652058));
#17028=CARTESIAN_POINT('Ctrl Pts',(-207.93881072326,-62.8625090659739,4.6083412453249));
#17029=CARTESIAN_POINT('Ctrl Pts',(-208.388521150012,-66.3127834459959,
4.7672495641292));
#17030=CARTESIAN_POINT('Ctrl Pts',(-205.731673259242,-68.5595126354467,
4.92615788293351));
#17031=CARTESIAN_POINT('Ctrl Pts',(-202.404035502155,-67.5429204246525,
5.08506620173781));
#17032=CARTESIAN_POINT('Ctrl Pts',(-201.456348982136,-64.1950071902349,
5.24397452054212));
#17033=CARTESIAN_POINT('Ctrl Pts',(-203.757442108639,-61.5851023665706,
5.40288283934643));
#17034=CARTESIAN_POINT('Ctrl Pts',(-207.197698422129,-62.1059375256302,
5.56179115815073));
#17035=CARTESIAN_POINT('Ctrl Pts',(-208.623129385432,-65.2800168148538,
5.72069947695504));
#17036=CARTESIAN_POINT('Ctrl Pts',(-206.726915823139,-68.1973798179096,
5.87960779575935));
#17037=CARTESIAN_POINT('Ctrl Pts',(-203.247485135573,-68.183420740359,6.03851611456365));
#17038=CARTESIAN_POINT('Ctrl Pts',(-201.374740488217,-65.2509371084826,
6.19742443336796));
#17039=CARTESIAN_POINT('Ctrl Pts',(-202.825593242488,-62.0883971402218,
6.35633275217227));
#17040=CARTESIAN_POINT('Ctrl Pts',(-206.26991780915,-61.5951821314221,6.51524107097657));
#17041=CARTESIAN_POINT('Ctrl Pts',(-208.549995921993,-64.2234660895895,
6.67414938978088));
#17042=CARTESIAN_POINT('Ctrl Pts',(-207.575477451123,-67.5636676576622,
6.83305770858519));
#17043=CARTESIAN_POINT('Ctrl Pts',(-204.239790038642,-68.5535273707736,
6.9919660273895));
#17044=CARTESIAN_POINT('Ctrl Pts',(-201.601054622025,-66.2855529074004,
7.15087434619379));
#17045=CARTESIAN_POINT('Ctrl Pts',(-202.078434338626,-62.8389979068817,
7.30978266499812));
#17046=CARTESIAN_POINT('Ctrl Pts',(-205.234272799839,-61.3736254722602,
7.46869098380241));
#17047=CARTESIAN_POINT('Ctrl Pts',(-208.175332576579,-63.2328726734323,
7.62759930260673));
#17048=CARTESIAN_POINT('Ctrl Pts',(-208.205282937147,-66.7122024567848,
7.78650762141103));
#17049=CARTESIAN_POINT('Ctrl Pts',(-205.296665725724,-68.62180416469,7.94541594021533));
#17050=CARTESIAN_POINT('Ctrl Pts',(-202.116068692728,-67.2109762945637,
8.10432425901964));
#17051=CARTESIAN_POINT('Ctrl Pts',(-201.579427649136,-63.7731500692063,
8.26323257782395));
#17052=CARTESIAN_POINT('Ctrl Pts',(-204.178729105786,-61.4600861481526,
8.42214089662826));
#17053=CARTESIAN_POINT('Ctrl Pts',(-207.530962539076,-62.3923756815873,
8.58104921543256));
#17054=CARTESIAN_POINT('Ctrl Pts',(-208.562837804587,-65.7153060452649,
8.73995753423686));
#17055=CARTESIAN_POINT('Ctrl Pts',(-206.328343191953,-68.3824518214713,
8.89886585304117));
#17056=CARTESIAN_POINT('Ctrl Pts',(-202.876038387555,-67.9486035727176,
9.05777417184548));
#17057=CARTESIAN_POINT('Ctrl Pts',(-201.370957850366,-64.8115085244288,
9.21668249064979));
#17058=CARTESIAN_POINT('Ctrl Pts',(-203.192942594908,-61.8472203542135,
9.3755908094541));
#17059=CARTESIAN_POINT('Ctrl Pts',(-206.671617371331,-61.7733653252889,
9.5344991282584));
#17060=CARTESIAN_POINT('Ctrl Pts',(-208.61777202504,-64.6576529027109,9.69340744706271));
#17061=CARTESIAN_POINT('Ctrl Pts',(-207.247193721282,-67.8558004725847,
9.85231576586701));
#17062=CARTESIAN_POINT('Ctrl Pts',(-203.816413330272,-68.4357820878843,
10.0112240846713));
#17063=CARTESIAN_POINT('Ctrl Pts',(-201.470731969365,-65.8658770860377,
10.1701324034756));
#17064=CARTESIAN_POINT('Ctrl Pts',(-202.360644093045,-62.5021456494408,
10.3290407222799));
#17065=CARTESIAN_POINT('Ctrl Pts',(-205.670288212686,-61.4284191634349,
10.4879490410842));
#17066=CARTESIAN_POINT('Ctrl Pts',(-208.365419590609,-63.6290780695714,
10.6468573598886));
#17067=CARTESIAN_POINT('Ctrl Pts',(-207.975171902461,-67.0865828790137,
10.8057656786928));
#17068=CARTESIAN_POINT('Ctrl Pts',(-204.857319867018,-68.6311318262819,
10.9646739974972));
#17069=CARTESIAN_POINT('Ctrl Pts',(-201.870275382787,-66.8466996996243,
11.1235823163015));
#17070=CARTESIAN_POINT('Ctrl Pts',(-201.752527447332,-63.3692339285321,
11.2824906351058));
#17071=CARTESIAN_POINT('Ctrl Pts',(-204.612026051834,-61.3868362650263,
11.4413989539101));
#17072=CARTESIAN_POINT('Ctrl Pts',(-207.82721483571,-62.7169467301605,11.6003072727144));
#17073=CARTESIAN_POINT('Ctrl Pts',(-208.450444657403,-66.140134915869,11.7592155915187));
#17074=CARTESIAN_POINT('Ctrl Pts',(-205.910345382095,-68.5180601537614,
11.918123910323));
#17075=CARTESIAN_POINT('Ctrl Pts',(-202.535651635225,-67.6706671633156,
12.0770322291273));
#17076=CARTESIAN_POINT('Ctrl Pts',(-201.420244925668,-64.3748363670382,
12.2359405479316));
#17077=CARTESIAN_POINT('Ctrl Pts',(-203.586717658077,-61.6521486021326,
12.3948488667359));
#17078=CARTESIAN_POINT('Ctrl Pts',(-207.048871845595,-61.9987335805548,
12.5537571855402));
#17079=CARTESIAN_POINT('Ctrl Pts',(-208.632643224891,-65.0968460677781,
12.7126655043445));
#17080=CARTESIAN_POINT('Ctrl Pts',(-206.886047896905,-68.1061711625154,
12.8715738231488));
#17081=CARTESIAN_POINT('Ctrl Pts',(-203.410344937013,-68.2677932524411,
13.0304821419532));
#17082=CARTESIAN_POINT('Ctrl Pts',(-201.392019971602,-65.433539012082,13.1893904607574));
#17083=CARTESIAN_POINT('Ctrl Pts',(-202.68145077062,-62.2018210508086,13.3482987795618));
#17084=CARTESIAN_POINT('Ctrl Pts',(-206.096501589105,-61.5354422759257,
13.5072070983661));
#17085=CARTESIAN_POINT('Ctrl Pts',(-208.506292006242,-64.0453312989241,
13.6661154171704));
#17086=CARTESIAN_POINT('Ctrl Pts',(-207.701553100804,-67.4304499187966,
13.8250237359747));
#17087=CARTESIAN_POINT('Ctrl Pts',(-204.420060507976,-68.5873592139186,
13.983932054779));
#17088=CARTESIAN_POINT('Ctrl Pts',(-201.670249958077,-66.4554176847852,
14.1428403735833));
#17089=CARTESIAN_POINT('Ctrl Pts',(-201.973117033763,-62.9891654728944,
14.3017486923876));
#17090=CARTESIAN_POINT('Ctrl Pts',(-205.050996575713,-61.3664239142234,
14.4606570111919));
#17091=CARTESIAN_POINT('Ctrl Pts',(-208.082123040074,-63.0749042303987,
14.6195653299962));
#17092=CARTESIAN_POINT('Ctrl Pts',(-208.287593522688,-66.548290973518,14.7784736488005));
#17093=CARTESIAN_POINT('Ctrl Pts',(-205.479035063749,-68.6022215651833,
14.9373819676048));
#17094=CARTESIAN_POINT('Ctrl Pts',(-202.231302498607,-67.3536762880221,
15.0962902864091));
#17095=CARTESIAN_POINT('Ctrl Pts',(-201.521881091931,-63.9473056596023,
15.2551986052134));
#17096=CARTESIAN_POINT('Ctrl Pts',(-204.001159743508,-61.5060359832025,
15.4141069240177));
#17097=CARTESIAN_POINT('Ctrl Pts',(-207.396164971614,-62.2679882236812,
15.5730152428221));
#17098=CARTESIAN_POINT('Ctrl Pts',(-208.594390890487,-65.5346291179969,
15.7319235616264));
#17099=CARTESIAN_POINT('Ctrl Pts',(-206.497323624104,-68.3111057941983,
15.8908318804307));
#17100=CARTESIAN_POINT('Ctrl Pts',(-203.027518128658,-68.0520434259267,
16.049740199235));
#17101=CARTESIAN_POINT('Ctrl Pts',(-201.366079806868,-64.9948075926078,
16.2086485180393));
#17102=CARTESIAN_POINT('Ctrl Pts',(-203.036142175806,-61.9425259545107,
16.3675568368436));
#17103=CARTESIAN_POINT('Ctrl Pts',(-206.506723058425,-61.6929032655643,
16.5264651556479));
#17104=CARTESIAN_POINT('Ctrl Pts',(-208.5958014629,-64.4760115385876,16.6853734744522));
#17105=CARTESIAN_POINT('Ctrl Pts',(-207.388609988071,-67.7378151779928,
16.8442817932565));
#17106=CARTESIAN_POINT('Ctrl Pts',(-203.990917296448,-68.4931171860738,
17.0031901120608));
#17107=CARTESIAN_POINT('Ctrl Pts',(-201.519758764249,-66.038774750277,17.1620984308651));
#17108=CARTESIAN_POINT('Ctrl Pts',(-201.999201820237,-63.780179352227,17.268037310068));
#17109=CARTESIAN_POINT('Ctrl Pts',(-202.663937342304,-63.0026984430694,
17.3210067496694));
#17110=CARTESIAN_POINT('Ctrl Pts',(-204.254067145653,-67.7901775698422,
-0.107002249889811));
#17111=CARTESIAN_POINT('Ctrl Pts',(-203.325449162499,-67.5419185807875,
-0.0540328102883759));
#17112=CARTESIAN_POINT('Ctrl Pts',(-201.751948395471,-66.0480439316771,
0.0519060689144955));
#17113=CARTESIAN_POINT('Ctrl Pts',(-202.359224676009,-62.8320206450648,
0.210814387718802));
#17114=CARTESIAN_POINT('Ctrl Pts',(-205.392461761202,-61.6083924207151,
0.369722706523109));
#17115=CARTESIAN_POINT('Ctrl Pts',(-208.063529457392,-63.4917903583777,
0.528631025327416));
#17116=CARTESIAN_POINT('Ctrl Pts',(-207.927136255583,-66.7590371611916,
0.687539344131722));
#17117=CARTESIAN_POINT('Ctrl Pts',(-205.106619392628,-68.4130649046996,
0.846447662936029));
#17118=CARTESIAN_POINT('Ctrl Pts',(-202.188626041087,-66.9383016977623,
1.00535598174034));
#17119=CARTESIAN_POINT('Ctrl Pts',(-201.847937285795,-63.6863945851504,
1.16426430054464));
#17120=CARTESIAN_POINT('Ctrl Pts',(-204.397088334585,-61.6388496605446,
1.32317261934895));
#17121=CARTESIAN_POINT('Ctrl Pts',(-207.498951002008,-62.6727389914087,
1.48208093815326));
#17122=CARTESIAN_POINT('Ctrl Pts',(-208.309818407223,-65.8402501689831,
1.64098925695756));
#17123=CARTESIAN_POINT('Ctrl Pts',(-206.08627396177,-68.2374221135446,1.79989757576187));
#17124=CARTESIAN_POINT('Ctrl Pts',(-202.866849248828,-67.6665651795,1.95880589456618));
#17125=CARTESIAN_POINT('Ctrl Pts',(-201.603071573705,-64.651029377315,2.11771421337048));
#17126=CARTESIAN_POINT('Ctrl Pts',(-203.453560752936,-61.9554267748013,
2.27662253217479));
#17127=CARTESIAN_POINT('Ctrl Pts',(-206.721807741666,-62.0510544718753,
2.43553085097909));
#17128=CARTESIAN_POINT('Ctrl Pts',(-208.4115208353,-64.8502426659663,2.59443916978341));
#17129=CARTESIAN_POINT('Ctrl Pts',(-206.973589660732,-67.7867266146009,
2.75334748858771));
#17130=CARTESIAN_POINT('Ctrl Pts',(-203.726293590367,-68.1683707960215,
2.91225580739202));
#17131=CARTESIAN_POINT('Ctrl Pts',(-201.646717297687,-65.6452880213436,
3.07116412619632));
#17132=CARTESIAN_POINT('Ctrl Pts',(-202.641393118574,-62.5306124118932,
3.23007244500063));
#17133=CARTESIAN_POINT('Ctrl Pts',(-205.798413361331,-61.6798437380682,
3.38898076380494));
#17134=CARTESIAN_POINT('Ctrl Pts',(-208.223457160724,-63.8729572190647,
3.54788908260924));
#17135=CARTESIAN_POINT('Ctrl Pts',(-207.693271461815,-67.0993309236441,
3.70679740141355));
#17136=CARTESIAN_POINT('Ctrl Pts',(-204.693924589467,-68.4010615018235,
3.86570572021786));
#17137=CARTESIAN_POINT('Ctrl Pts',(-201.975184232255,-66.5847369077965,
4.02461403902216));
#17138=CARTESIAN_POINT('Ctrl Pts',(-202.029561163317,-63.3155432291222,
4.18352235782647));
#17139=CARTESIAN_POINT('Ctrl Pts',(-204.807203219798,-61.5906406910937,
4.34243067663077));
#17140=CARTESIAN_POINT('Ctrl Pts',(-207.761599209553,-62.9914006618004,
4.50133899543508));
#17141=CARTESIAN_POINT('Ctrl Pts',(-208.184191909797,-66.2336220560524,
4.66024731423939));
#17142=CARTESIAN_POINT('Ctrl Pts',(-205.687553056201,-68.3448725372624,
4.8191556330437));
#17143=CARTESIAN_POINT('Ctrl Pts',(-202.560573245315,-67.3895812612549,
4.978063951848));
#17144=CARTESIAN_POINT('Ctrl Pts',(-201.670032618157,-64.2435485927867,
5.13697227065231));
#17145=CARTESIAN_POINT('Ctrl Pts',(-203.832368868315,-61.7910221197497,
5.29588058945662));
#17146=CARTESIAN_POINT('Ctrl Pts',(-207.06517628963,-62.2804507012443,5.45478890826092));
#17147=CARTESIAN_POINT('Ctrl Pts',(-208.404653170661,-65.2631316839978,
5.61369722706523));
#17148=CARTESIAN_POINT('Ctrl Pts',(-206.622782077934,-68.0045764798305,
5.77260554586953));
#17149=CARTESIAN_POINT('Ctrl Pts',(-203.353162513657,-67.9914591404848,
5.93151386467385));
#17150=CARTESIAN_POINT('Ctrl Pts',(-201.593345150497,-65.235805496063,6.09042218347814));
#17151=CARTESIAN_POINT('Ctrl Pts',(-202.956710877885,-62.2639680083999,
6.24933050228247));
#17152=CARTESIAN_POINT('Ctrl Pts',(-206.193341235007,-61.8004940705718,
6.40823882108676));
#17153=CARTESIAN_POINT('Ctrl Pts',(-208.335929685604,-64.2702914086274,
6.56714713989107));
#17154=CARTESIAN_POINT('Ctrl Pts',(-207.420175085435,-67.4090774274512,
6.72605545869537));
#17155=CARTESIAN_POINT('Ctrl Pts',(-204.285631016736,-68.3392481865482,
6.88496377749969));
#17156=CARTESIAN_POINT('Ctrl Pts',(-201.806012447539,-66.2080335303043,
7.04387209630399));
#17157=CARTESIAN_POINT('Ctrl Pts',(-202.2546059679,-62.9693072354186,7.20278041510831));
#17158=CARTESIAN_POINT('Ctrl Pts',(-205.220146052188,-61.5922973704678,
7.3616887339126));
#17159=CARTESIAN_POINT('Ctrl Pts',(-207.983858696358,-63.3394311890845,
7.52059705271692));
#17160=CARTESIAN_POINT('Ctrl Pts',(-208.012003037678,-66.6089559337142,
7.67950537152122));
#17161=CARTESIAN_POINT('Ctrl Pts',(-205.27877665859,-68.4034078612826,7.83841369032552));
#17162=CARTESIAN_POINT('Ctrl Pts',(-202.289970954736,-67.0776535008131,
7.99732200912983));
#17163=CARTESIAN_POINT('Ctrl Pts',(-201.785689590146,-63.8471296323018,
8.15623032793414));
#17164=CARTESIAN_POINT('Ctrl Pts',(-204.228252083627,-61.6735444315025,
8.31513864673845));
#17165=CARTESIAN_POINT('Ctrl Pts',(-207.378344441172,-62.5496165167955,
8.47404696554275));
#17166=CARTESIAN_POINT('Ctrl Pts',(-208.347997197315,-65.6721727920609,
8.63295528434706));
#17167=CARTESIAN_POINT('Ctrl Pts',(-206.248243542832,-68.1784885643011,
8.79186360315136));
#17168=CARTESIAN_POINT('Ctrl Pts',(-203.00411415964,-67.7708015460996,8.95077192195566));
#17169=CARTESIAN_POINT('Ctrl Pts',(-201.589790607288,-64.82287463911,9.10968024075999));
#17170=CARTESIAN_POINT('Ctrl Pts',(-203.301908910968,-62.0373342832907,
9.26858855956428));
#17171=CARTESIAN_POINT('Ctrl Pts',(-206.57081814586,-61.9679327434484,9.4274968783686));
#17172=CARTESIAN_POINT('Ctrl Pts',(-208.399618861337,-64.6782965756237,
9.58640519717289));
#17173=CARTESIAN_POINT('Ctrl Pts',(-207.111687001578,-67.6835945116545,
9.7453135159772));
#17174=CARTESIAN_POINT('Ctrl Pts',(-203.887784100661,-68.2286029933815,
9.90422183478151));
#17175=CARTESIAN_POINT('Ctrl Pts',(-201.683548305251,-65.8136643362045,
10.0631301535858));
#17176=CARTESIAN_POINT('Ctrl Pts',(-202.519798356292,-62.6527673097532,
10.2220384723901));
#17177=CARTESIAN_POINT('Ctrl Pts',(-205.629869553584,-61.6437869791857,
10.3809467911944));
#17178=CARTESIAN_POINT('Ctrl Pts',(-208.162483384071,-63.7117452344017,
10.5398551099987));
#17179=CARTESIAN_POINT('Ctrl Pts',(-207.795767794466,-66.960761060161,10.698763428803));
#17180=CARTESIAN_POINT('Ctrl Pts',(-204.865923538612,-68.4121730609857,
10.8576717476073));
#17181=CARTESIAN_POINT('Ctrl Pts',(-202.058999084014,-66.7353429366515,
11.0165800664117));
#17182=CARTESIAN_POINT('Ctrl Pts',(-201.948351398233,-63.4675698035645,
11.175488385216));
#17183=CARTESIAN_POINT('Ctrl Pts',(-204.635421042906,-61.604711546914,11.3343967040203));
#17184=CARTESIAN_POINT('Ctrl Pts',(-207.656732600619,-62.8546157956158,
11.4933050228246));
#17185=CARTESIAN_POINT('Ctrl Pts',(-208.242381403836,-66.0713843043812,
11.6522133416289));
#17186=CARTESIAN_POINT('Ctrl Pts',(-205.855451175442,-68.3059196575311,
11.8111216604332));
#17187=CARTESIAN_POINT('Ctrl Pts',(-202.684252870604,-67.5096248182363,
11.9700299792375));
#17188=CARTESIAN_POINT('Ctrl Pts',(-201.636105651369,-64.4125339951416,
12.1289382980418));
#17189=CARTESIAN_POINT('Ctrl Pts',(-203.671939173408,-61.8540254393122,
12.2878466168461));
#17190=CARTESIAN_POINT('Ctrl Pts',(-206.925324017804,-62.1797111988197,
12.4467549356504));
#17191=CARTESIAN_POINT('Ctrl Pts',(-208.413593321628,-65.0910062094532,
12.6056632544547));
#17192=CARTESIAN_POINT('Ctrl Pts',(-206.772318421206,-67.9188677444407,
12.764571573259));
#17193=CARTESIAN_POINT('Ctrl Pts',(-203.506201801068,-68.0707439548588,
12.9234798920633));
#17194=CARTESIAN_POINT('Ctrl Pts',(-201.609582673819,-65.4073964286302,
13.0823882108676));
#17195=CARTESIAN_POINT('Ctrl Pts',(-202.821260257257,-62.3705524098184,
13.2412965296719));
#17196=CARTESIAN_POINT('Ctrl Pts',(-206.03038208544,-61.744356553306,13.4002048484763));
#17197=CARTESIAN_POINT('Ctrl Pts',(-208.29486113422,-64.1028982202188,13.5591131672806));
#17198=CARTESIAN_POINT('Ctrl Pts',(-207.538648320798,-67.283892773864,13.7180214860849));
#17199=CARTESIAN_POINT('Ctrl Pts',(-204.455031101497,-68.3710399554251,
13.8769298048892));
#17200=CARTESIAN_POINT('Ctrl Pts',(-201.871035275935,-66.3676553906861,
14.0358381236935));
#17201=CARTESIAN_POINT('Ctrl Pts',(-202.155639340496,-63.1104196344985,
14.1947464424978));
#17202=CARTESIAN_POINT('Ctrl Pts',(-205.047921460904,-61.5855300693876,
14.3536547613021));
#17203=CARTESIAN_POINT('Ctrl Pts',(-207.896269733824,-63.1909883091252,
14.5125630801064));
#17204=CARTESIAN_POINT('Ctrl Pts',(-208.089350260542,-66.4549283813293,
14.6714713989107));
#17205=CARTESIAN_POINT('Ctrl Pts',(-205.450149049385,-68.3850061007028,
14.830379717715));
#17206=CARTESIAN_POINT('Ctrl Pts',(-202.398256114005,-67.2117486250819,
14.9892880365193));
#17207=CARTESIAN_POINT('Ctrl Pts',(-201.731613114368,-64.0107835678785,
15.1481963553236));
#17208=CARTESIAN_POINT('Ctrl Pts',(-204.061390228038,-61.7167234723125,
15.3071046741279));
#17209=CARTESIAN_POINT('Ctrl Pts',(-207.251675223312,-62.4327296745389,
15.4660129929322));
#17210=CARTESIAN_POINT('Ctrl Pts',(-208.377647618961,-65.5023907589485,
15.6249213117365));
#17211=CARTESIAN_POINT('Ctrl Pts',(-206.407034384366,-68.111444732263,15.7838296305409));
#17212=CARTESIAN_POINT('Ctrl Pts',(-203.146459609106,-67.8680039329691,
15.9427379493452));
#17213=CARTESIAN_POINT('Ctrl Pts',(-201.585206711849,-64.9951206969416,
16.1016462681495));
#17214=CARTESIAN_POINT('Ctrl Pts',(-203.15456362261,-62.1268929160954,16.2605545869538));
#17215=CARTESIAN_POINT('Ctrl Pts',(-206.415867028873,-61.8923225795219,
16.4194629057581));
#17216=CARTESIAN_POINT('Ctrl Pts',(-208.378973133268,-64.507608261601,16.5783712245624));
#17217=CARTESIAN_POINT('Ctrl Pts',(-207.244575808431,-67.572723779591,16.7372795433667));
#17218=CARTESIAN_POINT('Ctrl Pts',(-204.051765404813,-68.2824807612099,
16.896187862171));
#17219=CARTESIAN_POINT('Ctrl Pts',(-201.729618763932,-65.9761361990972,
17.0550961809753));
#17220=CARTESIAN_POINT('Ctrl Pts',(-202.180151203454,-63.8537350466212,
17.1610350601782));
#17221=CARTESIAN_POINT('Ctrl Pts',(-202.804802895981,-63.1231365609213,
17.2140044997796));
#17222=CARTESIAN_POINT('Ctrl Pts',(-204.301933573839,-67.6111321859386,
-0.214004499779622));
#17223=CARTESIAN_POINT('Ctrl Pts',(-203.43290490324,-67.378803948562,-0.161035060178186));
#17224=CARTESIAN_POINT('Ctrl Pts',(-201.960375505185,-65.9807910693062,
-0.0550961809753148));
#17225=CARTESIAN_POINT('Ctrl Pts',(-202.528682934436,-62.9711396388145,
0.103812137828991));
#17226=CARTESIAN_POINT('Ctrl Pts',(-205.367277533696,-61.8260315013409,
0.262720456633298));
#17227=CARTESIAN_POINT('Ctrl Pts',(-207.866943113308,-63.5885720031053,
0.421628775437605));
#17228=CARTESIAN_POINT('Ctrl Pts',(-207.739302248069,-66.646159942469,0.580537094241911));
#17229=CARTESIAN_POINT('Ctrl Pts',(-205.099777638078,-68.1940489098917,
0.739445413046219));
#17230=CARTESIAN_POINT('Ctrl Pts',(-202.369031594917,-66.8139210936934,
0.898353731850524));
#17231=CARTESIAN_POINT('Ctrl Pts',(-202.050204799108,-63.7706884983198,
1.05726205065483));
#17232=CARTESIAN_POINT('Ctrl Pts',(-204.435777109006,-61.8545343034827,
1.21617036945914));
#17233=CARTESIAN_POINT('Ctrl Pts',(-207.338593594527,-62.8220790711336,
1.37507868826345));
#17234=CARTESIAN_POINT('Ctrl Pts',(-208.097427728659,-65.7863314092215,
1.53398700706775));
#17235=CARTESIAN_POINT('Ctrl Pts',(-206.016567882626,-68.029677097083,1.69289532587206));
#17236=CARTESIAN_POINT('Ctrl Pts',(-203.003733294953,-67.4954519889176,
1.85180364467637));
#17237=CARTESIAN_POINT('Ctrl Pts',(-201.821052092491,-64.6734227833063,
2.01071196348067));
#17238=CARTESIAN_POINT('Ctrl Pts',(-203.552795587186,-62.1507966995761,
2.16962028228498));
#17239=CARTESIAN_POINT('Ctrl Pts',(-206.611319530648,-62.2402879779792,
2.32852860108929));
#17240=CARTESIAN_POINT('Ctrl Pts',(-208.192603923254,-64.8598525774122,
2.48743691989359));
#17241=CARTESIAN_POINT('Ctrl Pts',(-206.846944632009,-67.6079026781108,
2.6463452386979));
#17242=CARTESIAN_POINT('Ctrl Pts',(-203.808027188815,-67.965056794915,2.80525355750221));
#17243=CARTESIAN_POINT('Ctrl Pts',(-201.861897075226,-65.6038799608823,
2.96416187630651));
#17244=CARTESIAN_POINT('Ctrl Pts',(-202.792744659467,-62.6890727383964,
3.12307019511082));
#17245=CARTESIAN_POINT('Ctrl Pts',(-205.747179264856,-61.8928977956174,
3.28197851391512));
#17246=CARTESIAN_POINT('Ctrl Pts',(-208.01660827373,-63.9452794287941,3.44088683271943));
#17247=CARTESIAN_POINT('Ctrl Pts',(-207.520444532071,-66.9646170920847,
3.59979515152374));
#17248=CARTESIAN_POINT('Ctrl Pts',(-204.713565414472,-68.1828157640413,
3.75870347032805));
#17249=CARTESIAN_POINT('Ctrl Pts',(-202.169286323185,-66.4830445169217,
3.91761178913235));
#17250=CARTESIAN_POINT('Ctrl Pts',(-202.220173892637,-63.4236346325047,
4.07652010793666));
#17251=CARTESIAN_POINT('Ctrl Pts',(-204.819574967711,-61.8094188982323,
4.23542842674097));
#17252=CARTESIAN_POINT('Ctrl Pts',(-207.584387695847,-63.120292257627,4.39433674554527));
#17253=CARTESIAN_POINT('Ctrl Pts',(-207.979862669581,-66.154460666109,4.55324506434958));
#17254=CARTESIAN_POINT('Ctrl Pts',(-205.643432853161,-68.130232439078,4.71215338315389));
#17255=CARTESIAN_POINT('Ctrl Pts',(-202.717110988474,-67.2362420978575,
4.87106170195819));
#17256=CARTESIAN_POINT('Ctrl Pts',(-201.883716254178,-64.2920899953385,
5.0299700207625));
#17257=CARTESIAN_POINT('Ctrl Pts',(-203.907295627992,-61.9969418729286,
5.1888783395668));
#17258=CARTESIAN_POINT('Ctrl Pts',(-206.932654157132,-62.4549638768584,
5.34778665837112));
#17259=CARTESIAN_POINT('Ctrl Pts',(-208.18617695589,-65.2462465531416,5.50669497717542));
#17260=CARTESIAN_POINT('Ctrl Pts',(-206.518648332729,-67.8117731417515,
5.66560329597973));
#17261=CARTESIAN_POINT('Ctrl Pts',(-203.458839891741,-67.7994975406107,
5.82451161478403));
#17262=CARTESIAN_POINT('Ctrl Pts',(-201.811949812777,-65.2206738836432,
5.98341993358834));
#17263=CARTESIAN_POINT('Ctrl Pts',(-203.087828513282,-62.439538876578,6.14232825239265));
#17264=CARTESIAN_POINT('Ctrl Pts',(-206.116764660864,-62.0058060097215,
6.30123657119696));
#17265=CARTESIAN_POINT('Ctrl Pts',(-208.121863449215,-64.3171167276652,
6.46014489000126));
#17266=CARTESIAN_POINT('Ctrl Pts',(-207.264872719747,-67.2544871972402,
6.61905320880557));
#17267=CARTESIAN_POINT('Ctrl Pts',(-204.33147199483,-68.1249690023228,6.77796152760988));
#17268=CARTESIAN_POINT('Ctrl Pts',(-202.010970273053,-66.1305141532081,
6.93686984641418));
#17269=CARTESIAN_POINT('Ctrl Pts',(-202.430777597174,-63.0996165639554,
7.09577816521849));
#17270=CARTESIAN_POINT('Ctrl Pts',(-205.206019304538,-61.8109692686754,
7.25468648402279));
#17271=CARTESIAN_POINT('Ctrl Pts',(-207.792384816137,-63.4459897047368,
7.4135948028271));
#17272=CARTESIAN_POINT('Ctrl Pts',(-207.818723138209,-66.5057094106436,
7.5725031216314));
#17273=CARTESIAN_POINT('Ctrl Pts',(-205.260887591457,-68.1850115578752,
7.73141144043572));
#17274=CARTESIAN_POINT('Ctrl Pts',(-202.463873216744,-66.9443307070625,
7.89031975924001));
#17275=CARTESIAN_POINT('Ctrl Pts',(-201.991951531155,-63.9211091953971,
8.04922807804433));
#17276=CARTESIAN_POINT('Ctrl Pts',(-204.277775061468,-61.8870027148524,
8.20813639684863));
#17277=CARTESIAN_POINT('Ctrl Pts',(-207.225726343268,-62.7068573520037,
8.36704471565294));
#17278=CARTESIAN_POINT('Ctrl Pts',(-208.133156590043,-65.629039538857,8.52595303445725));
#17279=CARTESIAN_POINT('Ctrl Pts',(-206.16814389371,-67.9745253071309,8.68486135326155));
#17280=CARTESIAN_POINT('Ctrl Pts',(-203.132189931727,-67.5929995194816,
8.84376967206586));
#17281=CARTESIAN_POINT('Ctrl Pts',(-201.808623364209,-64.8342407537912,
9.00267799087017));
#17282=CARTESIAN_POINT('Ctrl Pts',(-203.410875227028,-62.227448212368,9.16158630967447));
#17283=CARTESIAN_POINT('Ctrl Pts',(-206.470018920388,-62.162500161608,9.32049462847879));
#17284=CARTESIAN_POINT('Ctrl Pts',(-208.181465697634,-64.6989402485364,
9.47940294728307));
#17285=CARTESIAN_POINT('Ctrl Pts',(-206.976180281873,-67.5113885507243,
9.63831126608739));
#17286=CARTESIAN_POINT('Ctrl Pts',(-203.95915487105,-68.0214238988787,9.7972195848917));
#17287=CARTESIAN_POINT('Ctrl Pts',(-201.896364641136,-65.7614515863713,
9.956127903696));
#17288=CARTESIAN_POINT('Ctrl Pts',(-202.678952619539,-62.8033889700657,
10.1150362225003));
#17289=CARTESIAN_POINT('Ctrl Pts',(-205.589450894481,-61.8591547949365,
10.2739445413046));
#17290=CARTESIAN_POINT('Ctrl Pts',(-207.959547177534,-63.7944123992321,
10.4328528601089));
#17291=CARTESIAN_POINT('Ctrl Pts',(-207.616363686471,-66.8349392413083,
10.5917611789132));
#17292=CARTESIAN_POINT('Ctrl Pts',(-204.874527210207,-68.1932142956896,
10.7506694977175));
#17293=CARTESIAN_POINT('Ctrl Pts',(-202.247722785242,-66.6239861736786,
10.9095778165219));
#17294=CARTESIAN_POINT('Ctrl Pts',(-202.144175349134,-63.5659056785969,
11.0684861353262));
#17295=CARTESIAN_POINT('Ctrl Pts',(-204.658816033978,-61.8225868288017,
11.2273944541305));
#17296=CARTESIAN_POINT('Ctrl Pts',(-207.486250365528,-62.9922848610711,
11.3863027729348));
#17297=CARTESIAN_POINT('Ctrl Pts',(-208.034318150269,-66.0026336928935,
11.5452110917391));
#17298=CARTESIAN_POINT('Ctrl Pts',(-205.800556968789,-68.0937791613008,
11.7041194105434));
#17299=CARTESIAN_POINT('Ctrl Pts',(-202.832854105983,-67.3485824731571,
11.8630277293477));
#17300=CARTESIAN_POINT('Ctrl Pts',(-201.851966377071,-64.4502316232448,
12.021936048152));
#17301=CARTESIAN_POINT('Ctrl Pts',(-203.757160688739,-62.0559022764919,
12.1808443669563));
#17302=CARTESIAN_POINT('Ctrl Pts',(-206.801776190012,-62.3606888170845,
12.3397526857606));
#17303=CARTESIAN_POINT('Ctrl Pts',(-208.194543418365,-65.0851663511284,
12.4986610045649));
#17304=CARTESIAN_POINT('Ctrl Pts',(-206.658588945508,-67.7315643263658,
12.6575693233692));
#17305=CARTESIAN_POINT('Ctrl Pts',(-203.602058665123,-67.8736946572765,
12.8164776421735));
#17306=CARTESIAN_POINT('Ctrl Pts',(-201.827145376036,-65.3812538451784,
12.9753859609778));
#17307=CARTESIAN_POINT('Ctrl Pts',(-202.961069743894,-62.5392837688283,
13.1342942797821));
#17308=CARTESIAN_POINT('Ctrl Pts',(-205.964262581775,-61.9532708306864,
13.2932025985864));
#17309=CARTESIAN_POINT('Ctrl Pts',(-208.083430262199,-64.1604651415136,
13.4521109173907));
#17310=CARTESIAN_POINT('Ctrl Pts',(-207.375743540791,-67.1373356289315,
13.6110192361951));
#17311=CARTESIAN_POINT('Ctrl Pts',(-204.490001695019,-68.1547206969317,
13.7699275549994));
#17312=CARTESIAN_POINT('Ctrl Pts',(-202.071820593793,-66.279893096587,13.9288358738037));
#17313=CARTESIAN_POINT('Ctrl Pts',(-202.338161647229,-63.2316737961026,
14.087744192608));
#17314=CARTESIAN_POINT('Ctrl Pts',(-205.044846346095,-61.8046362245518,
14.2466525114123));
#17315=CARTESIAN_POINT('Ctrl Pts',(-207.710416427574,-63.3070723878518,
14.4055608302166));
#17316=CARTESIAN_POINT('Ctrl Pts',(-207.891106998396,-66.3615657891406,
14.5644691490209));
#17317=CARTESIAN_POINT('Ctrl Pts',(-205.421263035021,-68.1677906362224,
14.7233774678252));
#17318=CARTESIAN_POINT('Ctrl Pts',(-202.565209729402,-67.0698209621416,
14.8822857866295));
#17319=CARTESIAN_POINT('Ctrl Pts',(-201.941345136806,-64.0742614761548,
15.0411941054338));
#17320=CARTESIAN_POINT('Ctrl Pts',(-204.121620712568,-61.9274109614226,
15.2001024242381));
#17321=CARTESIAN_POINT('Ctrl Pts',(-207.10718547501,-62.5974711253967,15.3590107430424));
#17322=CARTESIAN_POINT('Ctrl Pts',(-208.160904347434,-65.4701523999,15.5179190618468));
#17323=CARTESIAN_POINT('Ctrl Pts',(-206.316745144628,-67.9117836703277,
15.6768273806511));
#17324=CARTESIAN_POINT('Ctrl Pts',(-203.265401089553,-67.6839644400115,
15.8357356994554));
#17325=CARTESIAN_POINT('Ctrl Pts',(-201.80433361683,-64.9954338012754,15.9946440182597));
#17326=CARTESIAN_POINT('Ctrl Pts',(-203.272985069414,-62.3112598776802,
16.153552337064));
#17327=CARTESIAN_POINT('Ctrl Pts',(-206.325010999321,-62.0917418934795,
16.3124606558683));
#17328=CARTESIAN_POINT('Ctrl Pts',(-208.162144803636,-64.5392049846145,
16.4713689746726));
#17329=CARTESIAN_POINT('Ctrl Pts',(-207.100541628792,-67.4076323811892,
16.6302772934769));
#17330=CARTESIAN_POINT('Ctrl Pts',(-204.112613513177,-68.0718443363461,
16.7891856122812));
#17331=CARTESIAN_POINT('Ctrl Pts',(-201.939478763615,-65.9134976479173,
16.9480939310855));
#17332=CARTESIAN_POINT('Ctrl Pts',(-202.36110058667,-63.9272907410154,17.0540328102884));
#17333=CARTESIAN_POINT('Ctrl Pts',(-202.945668449658,-63.2435746787732,
17.1070022498898));
#17334=CARTESIAN_POINT('Ctrl Pts',(-204.349800002025,-67.4320868020351,
-0.321006749669433));
#17335=CARTESIAN_POINT('Ctrl Pts',(-203.540360643981,-67.2156893163365,
-0.268037310067997));
#17336=CARTESIAN_POINT('Ctrl Pts',(-202.168802614899,-65.9135382069353,
-0.162098430865125));
#17337=CARTESIAN_POINT('Ctrl Pts',(-202.698141192863,-63.1102586325642,
-0.00319011206081941));
#17338=CARTESIAN_POINT('Ctrl Pts',(-205.34209330619,-62.0436705819667,0.155718206743488));
#17339=CARTESIAN_POINT('Ctrl Pts',(-207.670356769225,-63.6853536478328,
0.314626525547794));
#17340=CARTESIAN_POINT('Ctrl Pts',(-207.551468240555,-66.5332827237463,
0.473534844352101));
#17341=CARTESIAN_POINT('Ctrl Pts',(-205.092935883528,-67.9750329150838,
0.632443163156408));
#17342=CARTESIAN_POINT('Ctrl Pts',(-202.549437148746,-66.6895404896243,
0.791351481960714));
#17343=CARTESIAN_POINT('Ctrl Pts',(-202.25247231242,-63.8549824114892,0.95025980076502));
#17344=CARTESIAN_POINT('Ctrl Pts',(-204.474465883427,-62.0702189464208,
1.10916811956933));
#17345=CARTESIAN_POINT('Ctrl Pts',(-207.178236187047,-62.9714191508586,
1.26807643837363));
#17346=CARTESIAN_POINT('Ctrl Pts',(-207.885037050096,-65.7324126494599,
1.42698475717794));
#17347=CARTESIAN_POINT('Ctrl Pts',(-205.946861803482,-67.8219320806215,
1.58589307598225));
#17348=CARTESIAN_POINT('Ctrl Pts',(-203.140617341079,-67.324338798335,1.74480139478656));
#17349=CARTESIAN_POINT('Ctrl Pts',(-202.039032611277,-64.6958161892978,
1.90370971359086));
#17350=CARTESIAN_POINT('Ctrl Pts',(-203.652030421438,-62.3461666243507,
2.06261803239517));
#17351=CARTESIAN_POINT('Ctrl Pts',(-206.50083131963,-62.4295214840832,2.22152635119947));
#17352=CARTESIAN_POINT('Ctrl Pts',(-207.973687011208,-64.869462488858,2.38043467000378));
#17353=CARTESIAN_POINT('Ctrl Pts',(-206.720299603286,-67.4290787416208,
2.53934298880809));
#17354=CARTESIAN_POINT('Ctrl Pts',(-203.889760787264,-67.7617427938084,
2.6982513076124));
#17355=CARTESIAN_POINT('Ctrl Pts',(-202.077076852765,-65.5624719004209,
2.8571596264167));
#17356=CARTESIAN_POINT('Ctrl Pts',(-202.944096200361,-62.8475330648997,
3.01606794522101));
#17357=CARTESIAN_POINT('Ctrl Pts',(-205.695945168382,-62.1059518531665,
3.17497626402531));
#17358=CARTESIAN_POINT('Ctrl Pts',(-207.809759386736,-64.0176016385234,
3.33388458282963));
#17359=CARTESIAN_POINT('Ctrl Pts',(-207.347617602327,-66.8299032605253,
3.49279290163393));
#17360=CARTESIAN_POINT('Ctrl Pts',(-204.733206239477,-67.9645700262592,
3.65170122043824));
#17361=CARTESIAN_POINT('Ctrl Pts',(-202.363388414116,-66.3813521260468,
3.81060953924254));
#17362=CARTESIAN_POINT('Ctrl Pts',(-202.410786621957,-63.5317260358873,
3.96951785804685));
#17363=CARTESIAN_POINT('Ctrl Pts',(-204.831946715624,-62.0281971053708,
4.12842617685115));
#17364=CARTESIAN_POINT('Ctrl Pts',(-207.40717618214,-63.2491838534535,4.28733449565546));
#17365=CARTESIAN_POINT('Ctrl Pts',(-207.775533429366,-66.0752992761655,
4.44624281445977));
#17366=CARTESIAN_POINT('Ctrl Pts',(-205.59931265012,-67.9155923408937,4.60515113326408));
#17367=CARTESIAN_POINT('Ctrl Pts',(-202.873648731634,-67.0829029344599,
4.76405945206838));
#17368=CARTESIAN_POINT('Ctrl Pts',(-202.097399890199,-64.3406313978904,
4.92296777087269));
#17369=CARTESIAN_POINT('Ctrl Pts',(-203.982222387668,-62.2028616261076,
5.08187608967699));
#17370=CARTESIAN_POINT('Ctrl Pts',(-206.800132024633,-62.6294770524725,
5.2407844084813));
#17371=CARTESIAN_POINT('Ctrl Pts',(-207.967700741118,-65.2293614222855,
5.39969272728561));
#17372=CARTESIAN_POINT('Ctrl Pts',(-206.414514587523,-67.6189698036725,
5.55860104608992));
#17373=CARTESIAN_POINT('Ctrl Pts',(-203.564517269825,-67.6075359407365,
5.71750936489422));
#17374=CARTESIAN_POINT('Ctrl Pts',(-202.030554475057,-65.2055422712234,
5.87641768369853));
#17375=CARTESIAN_POINT('Ctrl Pts',(-203.218946148679,-62.6151097447562,
6.03532600250284));
#17376=CARTESIAN_POINT('Ctrl Pts',(-206.040188086721,-62.2111179488711,
6.19423432130714));
#17377=CARTESIAN_POINT('Ctrl Pts',(-207.907797212825,-64.363942046703,6.35314264011145));
#17378=CARTESIAN_POINT('Ctrl Pts',(-207.109570354059,-67.0998969670293,
6.51205095891575));
#17379=CARTESIAN_POINT('Ctrl Pts',(-204.377312972924,-67.9106898180974,
6.67095927772007));
#17380=CARTESIAN_POINT('Ctrl Pts',(-202.215928098567,-66.0529947761121,
6.82986759652436));
#17381=CARTESIAN_POINT('Ctrl Pts',(-202.606949226449,-63.2299258924922,
6.98877591532868));
#17382=CARTESIAN_POINT('Ctrl Pts',(-205.191892556888,-62.0296411668831,
7.14768423413298));
#17383=CARTESIAN_POINT('Ctrl Pts',(-207.600910935916,-63.552548220389,7.30659255293729));
#17384=CARTESIAN_POINT('Ctrl Pts',(-207.62544323874,-66.4024628875731,7.46550087174159));
#17385=CARTESIAN_POINT('Ctrl Pts',(-205.242998524324,-67.9666152544678,
7.6244091905459));
#17386=CARTESIAN_POINT('Ctrl Pts',(-202.637775478752,-66.8110079133119,
7.78331750935021));
#17387=CARTESIAN_POINT('Ctrl Pts',(-202.198213472165,-63.9950887584926,
7.94222582815451));
#17388=CARTESIAN_POINT('Ctrl Pts',(-204.327298039309,-62.1004609982022,
8.10113414695882));
#17389=CARTESIAN_POINT('Ctrl Pts',(-207.073108245363,-62.864098187212,8.26004246576313));
#17390=CARTESIAN_POINT('Ctrl Pts',(-207.918315982771,-65.5859062856529,
8.41895078456743));
#17391=CARTESIAN_POINT('Ctrl Pts',(-206.088044244589,-67.7705620499607,
8.57785910337174));
#17392=CARTESIAN_POINT('Ctrl Pts',(-203.260265703813,-67.4151974928637,
8.73676742217605));
#17393=CARTESIAN_POINT('Ctrl Pts',(-202.027456121131,-64.8456068684723,
8.89567574098036));
#17394=CARTESIAN_POINT('Ctrl Pts',(-203.519841543088,-62.4175621414454,
9.05458405978466));
#17395=CARTESIAN_POINT('Ctrl Pts',(-206.369219694917,-62.3570675797674,
9.21349237858898));
#17396=CARTESIAN_POINT('Ctrl Pts',(-207.963312533931,-64.7195839214493,
9.37240069739327));
#17397=CARTESIAN_POINT('Ctrl Pts',(-206.840673562169,-67.3391825897941,
9.53130901619758));
#17398=CARTESIAN_POINT('Ctrl Pts',(-204.030525641438,-67.8142448043757,
9.69021733500189));
#17399=CARTESIAN_POINT('Ctrl Pts',(-202.109180977022,-65.7092388365381,
9.84912565380619));
#17400=CARTESIAN_POINT('Ctrl Pts',(-202.838106882786,-62.9540106303781,
10.0080339726105));
#17401=CARTESIAN_POINT('Ctrl Pts',(-205.549032235379,-62.0745226106873,
10.1669422914148));
#17402=CARTESIAN_POINT('Ctrl Pts',(-207.756610970996,-63.8770795640624,
10.3258506102191));
#17403=CARTESIAN_POINT('Ctrl Pts',(-207.436959578475,-66.7091174224556,
10.4847589290234));
#17404=CARTESIAN_POINT('Ctrl Pts',(-204.883130881801,-67.9742555303935,
10.6436672478277));
#17405=CARTESIAN_POINT('Ctrl Pts',(-202.43644648647,-66.5126294107058,10.802575566632));
#17406=CARTESIAN_POINT('Ctrl Pts',(-202.339999300035,-63.6642415536293,
10.9614838854363));
#17407=CARTESIAN_POINT('Ctrl Pts',(-204.68221102505,-62.0404621106893,11.1203922042406));
#17408=CARTESIAN_POINT('Ctrl Pts',(-207.315768130438,-63.1299539265266,
11.279300523045));
#17409=CARTESIAN_POINT('Ctrl Pts',(-207.826254896701,-65.9338830814056,
11.4382088418493));
#17410=CARTESIAN_POINT('Ctrl Pts',(-205.745662762136,-67.8816386650706,
11.5971171606536));
#17411=CARTESIAN_POINT('Ctrl Pts',(-202.981455341363,-67.1875401280777,
11.7560254794579));
#17412=CARTESIAN_POINT('Ctrl Pts',(-202.067827102772,-64.4879292513482,
11.9149337982622));
#17413=CARTESIAN_POINT('Ctrl Pts',(-203.84238220407,-62.2577791136714,12.0738421170665));
#17414=CARTESIAN_POINT('Ctrl Pts',(-206.678228362221,-62.5416664353495,
12.2327504358708));
#17415=CARTESIAN_POINT('Ctrl Pts',(-207.975493515101,-65.0793264928035,
12.3916587546751));
#17416=CARTESIAN_POINT('Ctrl Pts',(-206.544859469809,-67.5442609082911,
12.5505670734794));
#17417=CARTESIAN_POINT('Ctrl Pts',(-203.697915529178,-67.6766453596943,
12.7094753922837));
#17418=CARTESIAN_POINT('Ctrl Pts',(-202.044708078252,-65.3551112617265,
12.868383711088));
#17419=CARTESIAN_POINT('Ctrl Pts',(-203.100879230531,-62.7080151278382,
13.0272920298923));
#17420=CARTESIAN_POINT('Ctrl Pts',(-205.89814307811,-62.1621851080667,13.1862003486966));
#17421=CARTESIAN_POINT('Ctrl Pts',(-207.871999390178,-64.2180320628083,
13.3451086675009));
#17422=CARTESIAN_POINT('Ctrl Pts',(-207.212838760785,-66.9907784839988,
13.5040169863053));
#17423=CARTESIAN_POINT('Ctrl Pts',(-204.52497228854,-67.9384014384382,13.6629253051096));
#17424=CARTESIAN_POINT('Ctrl Pts',(-202.272605911651,-66.192130802488,13.8218336239139));
#17425=CARTESIAN_POINT('Ctrl Pts',(-202.520683953961,-63.3529279577067,
13.9807419427182));
#17426=CARTESIAN_POINT('Ctrl Pts',(-205.041771231286,-62.0237423797161,
14.1396502615225));
#17427=CARTESIAN_POINT('Ctrl Pts',(-207.524563121323,-63.4231564665784,
14.2985585803268));
#17428=CARTESIAN_POINT('Ctrl Pts',(-207.692863736251,-66.2682031969519,
14.4574668991311));
#17429=CARTESIAN_POINT('Ctrl Pts',(-205.392377020657,-67.9505751717419,
14.6163752179354));
#17430=CARTESIAN_POINT('Ctrl Pts',(-202.7321633448,-66.9278932992014,14.7752835367397));
#17431=CARTESIAN_POINT('Ctrl Pts',(-202.151077159244,-64.137739384431,14.934191855544));
#17432=CARTESIAN_POINT('Ctrl Pts',(-204.181851197098,-62.1380984505328,
15.0931001743483));
#17433=CARTESIAN_POINT('Ctrl Pts',(-206.962695726708,-62.7622125762542,
15.2520084931526));
#17434=CARTESIAN_POINT('Ctrl Pts',(-207.944161075907,-65.4379140408516,
15.4109168119569));
#17435=CARTESIAN_POINT('Ctrl Pts',(-206.226455904891,-67.7121226083924,
15.5698251307612));
#17436=CARTESIAN_POINT('Ctrl Pts',(-203.38434257,-67.499924947054,15.7287334495656));
#17437=CARTESIAN_POINT('Ctrl Pts',(-202.023460521812,-64.9957469056093,
15.8876417683698));
#17438=CARTESIAN_POINT('Ctrl Pts',(-203.391406516217,-62.4956268392649,
16.0465500871742));
#17439=CARTESIAN_POINT('Ctrl Pts',(-206.234154969769,-62.2911612074372,
16.2054584059785));
#17440=CARTESIAN_POINT('Ctrl Pts',(-207.945316474004,-64.5708017076279,
16.3643667247828));
#17441=CARTESIAN_POINT('Ctrl Pts',(-206.956507449152,-67.2425409827873,
16.5232750435871));
#17442=CARTESIAN_POINT('Ctrl Pts',(-204.173461621541,-67.8612079114822,
16.6821833623914));
#17443=CARTESIAN_POINT('Ctrl Pts',(-202.149338763299,-65.8508590967375,
16.8410916811957));
#17444=CARTESIAN_POINT('Ctrl Pts',(-202.542049969887,-64.0008464354096,
16.9470305603986));
#17445=CARTESIAN_POINT('Ctrl Pts',(-203.086534003335,-63.3640127966251,
17.));
#17446=CARTESIAN_POINT('Ctrl Pts',(-202.485823045017,-64.9986459985219,
0.88741669750801));
#17447=CARTESIAN_POINT('Ctrl Pts',(-202.484195117705,-64.6662426784437,
0.90836439859368));
#17448=CARTESIAN_POINT('Ctrl Pts',(-202.545417607547,-64.3344135715533,
0.92931209967935));
#17449=CARTESIAN_POINT('Ctrl Pts',(-202.672298713642,-64.0299481803337,
0.95025980076502));
#17450=CARTESIAN_POINT('Ctrl Pts',(-202.993136836089,-63.2600612564664,
1.00322924036646));
#17451=CARTESIAN_POINT('Ctrl Pts',(-203.733801359758,-62.6651401014436,
1.05619867996789));
#17452=CARTESIAN_POINT('Ctrl Pts',(-204.554762005529,-62.5178795580052,
1.10916811956933));
#17453=CARTESIAN_POINT('Ctrl Pts',(-205.3757226513,-62.3706190145667,1.16213755917076));
#17454=CARTESIAN_POINT('Ctrl Pts',(-206.276979419173,-62.6710190827126,
1.2151069987722));
#17455=CARTESIAN_POINT('Ctrl Pts',(-206.845407946952,-63.2813846998858,
1.26807643837363));
#17456=CARTESIAN_POINT('Ctrl Pts',(-207.41383647473,-63.891750317059,1.32104587797507));
#17457=CARTESIAN_POINT('Ctrl Pts',(-207.649436762413,-64.8120814832594,
1.37401531757651));
#17458=CARTESIAN_POINT('Ctrl Pts',(-207.444207698485,-65.6205003048866,
1.42698475717794));
#17459=CARTESIAN_POINT('Ctrl Pts',(-207.238978634558,-66.4289191265138,
1.47995419677938));
#17460=CARTESIAN_POINT('Ctrl Pts',(-206.59292021902,-67.1254256035676,1.53292363638081));
#17461=CARTESIAN_POINT('Ctrl Pts',(-205.80218360085,-67.3907466283802,1.58589307598225));
#17462=CARTESIAN_POINT('Ctrl Pts',(-205.011446982681,-67.6560676531927,
1.63886251558368));
#17463=CARTESIAN_POINT('Ctrl Pts',(-204.07603216188,-67.4902032257639,1.69183195518512));
#17464=CARTESIAN_POINT('Ctrl Pts',(-203.424727296512,-66.9691839105433,
1.74480139478655));
#17465=CARTESIAN_POINT('Ctrl Pts',(-202.840201318028,-66.5015851849195,
1.79233982902704));
#17466=CARTESIAN_POINT('Ctrl Pts',(-202.484511916232,-65.7479266885556,
1.83987826326752));
#17467=CARTESIAN_POINT('Ctrl Pts',(-202.479332426993,-64.9985362476049,
1.88741669750801));
#17468=CARTESIAN_POINT('Ctrl Pts',(-204.206200717467,-67.9692229537457,
-8.32667268468867E-16));
#17469=CARTESIAN_POINT('Ctrl Pts',(-204.113162270877,-67.935189074383,-8.43666019689578E-16));
#17470=CARTESIAN_POINT('Ctrl Pts',(-204.022191224303,-67.8963833673696,
-7.93411407245791E-16));
#17471=CARTESIAN_POINT('Ctrl Pts',(-203.933495016826,-67.8531352315209,
-8.39606162372775E-16));
#17472=CARTESIAN_POINT('Ctrl Pts',(-203.84282083649,-67.8089226391153,-8.86831085242262E-16));
#17473=CARTESIAN_POINT('Ctrl Pts',(-203.754523420144,-67.7600666539124,
-9.43046358883727E-16));
#17474=CARTESIAN_POINT('Ctrl Pts',(-203.668853328449,-67.706873635749,-9.61036805691151E-16));
#17475=CARTESIAN_POINT('Ctrl Pts',(-203.585825222369,-67.6553210405853,
-9.78472443921523E-16));
#17476=CARTESIAN_POINT('Ctrl Pts',(-203.505264559179,-67.599693926327,-6.24341674353395E-16));
#17477=CARTESIAN_POINT('Ctrl Pts',(-203.427433248919,-67.5402403758356,
-5.27355936696949E-16));
#17478=CARTESIAN_POINT('Ctrl Pts',(-203.359330852442,-67.4882185191557,
-4.42493416247559E-16));
#17479=CARTESIAN_POINT('Ctrl Pts',(-203.293318414644,-67.4332663265531,
-7.68735084580293E-16));
#17480=CARTESIAN_POINT('Ctrl Pts',(-203.229596756254,-67.3755369799182,
-7.56339435525888E-16));
#17481=CARTESIAN_POINT('Ctrl Pts',(-203.216348808853,-67.3635348543143,
-7.53762338337633E-16));
#17482=CARTESIAN_POINT('Ctrl Pts',(-203.203198226301,-67.3514108995448,
-7.71802573975562E-16));
#17483=CARTESIAN_POINT('Ctrl Pts',(-203.190163693746,-67.3391825254392,
-7.63278329429795E-16));
#17484=CARTESIAN_POINT('Ctrl Pts',(-203.117740153311,-67.2712382287989,
-7.15915221706024E-16));
#17485=CARTESIAN_POINT('Ctrl Pts',(-203.048782419931,-67.1999720891002,
-1.01902361823498E-15));
#17486=CARTESIAN_POINT('Ctrl Pts',(-202.983529622551,-67.1256761154066,
-1.06858966120171E-15));
#17487=CARTESIAN_POINT('Ctrl Pts',(-202.918635398475,-67.0517884085421,
-1.11788333178828E-15));
#17488=CARTESIAN_POINT('Ctrl Pts',(-202.857405018863,-66.9749032753298,
-6.33633973634577E-16));
#17489=CARTESIAN_POINT('Ctrl Pts',(-202.800117313271,-66.8952811970425,
-6.52256026967279E-16));
#17490=CARTESIAN_POINT('Ctrl Pts',(-202.744165816032,-66.8175162656787,
-6.7044372980576E-16));
#17491=CARTESIAN_POINT('Ctrl Pts',(-202.691974930395,-66.7371398344541,
-1.00351063719331E-15));
#17492=CARTESIAN_POINT('Ctrl Pts',(-202.643851583745,-66.6543804051971,
-9.85322934354826E-16));
#17493=CARTESIAN_POINT('Ctrl Pts',(-202.623072237245,-66.6186454246452,
-9.77469603162805E-16));
#17494=CARTESIAN_POINT('Ctrl Pts',(-202.603051895676,-66.5824660271048,
-9.98257832788744E-16));
#17495=CARTESIAN_POINT('Ctrl Pts',(-202.583818283756,-66.5458602757777,
-9.85322934354826E-16));
#17496=CARTESIAN_POINT('Ctrl Pts',(-202.569903871651,-66.5193781198792,
-9.75965279220305E-16));
#17497=CARTESIAN_POINT('Ctrl Pts',(-202.556401247797,-66.4926728201715,
-7.49717931409916E-16));
#17498=CARTESIAN_POINT('Ctrl Pts',(-202.543321546688,-66.4657512130594,
-7.21644966006352E-16));
#17499=CARTESIAN_POINT('Ctrl Pts',(-202.537160136435,-66.4530693432883,
-7.08420729806322E-16));
#17500=CARTESIAN_POINT('Ctrl Pts',(-202.531094761039,-66.4403438700637,
-5.91077345936009E-16));
#17501=CARTESIAN_POINT('Ctrl Pts',(-202.525129585519,-66.4275826355722,
-5.96744875736022E-16));
#17502=CARTESIAN_POINT('Ctrl Pts',(-202.485113226786,-66.3419760787267,
-6.34764529110435E-16));
#17503=CARTESIAN_POINT('Ctrl Pts',(-202.449555099265,-66.2546652571579,
-7.35539575560742E-16));
#17504=CARTESIAN_POINT('Ctrl Pts',(-202.418706921757,-66.1658877660811,
-6.38378239159465E-16));
#17505=CARTESIAN_POINT('Ctrl Pts',(-202.38854293449,-66.0790792954752,-5.4337187084792E-16));
#17506=CARTESIAN_POINT('Ctrl Pts',(-202.362882072143,-65.9908678196851,
-9.23815234263263E-16));
#17507=CARTESIAN_POINT('Ctrl Pts',(-202.342008857865,-65.9014669200007,
-9.99200722162641E-16));
#17508=CARTESIAN_POINT('Ctrl Pts',(-202.338628864872,-65.8869902605616,
-1.01140787039958E-15));
#17509=CARTESIAN_POINT('Ctrl Pts',(-202.335374520679,-65.8724824066537,
-1.33627779352685E-15));
#17510=CARTESIAN_POINT('Ctrl Pts',(-202.332247164121,-65.8579442614285,
-1.36002320516582E-15));
#17511=CARTESIAN_POINT('Ctrl Pts',(-202.312208856065,-65.7647921608561,
-1.54206868173359E-15));
#17512=CARTESIAN_POINT('Ctrl Pts',(-202.297379937046,-65.6703953939466,
-1.18629651745573E-15));
#17513=CARTESIAN_POINT('Ctrl Pts',(-202.287681809579,-65.5751623462816,
-1.11022302462516E-15));
#17514=CARTESIAN_POINT('Ctrl Pts',(-202.284326013292,-65.5422093139731,
-1.08389968069644E-15));
#17515=CARTESIAN_POINT('Ctrl Pts',(-202.281584984168,-65.5091562792113,
-4.63048300924823E-16));
#17516=CARTESIAN_POINT('Ctrl Pts',(-202.279456820056,-65.4760206859389,
-4.16333634234434E-16));
#17517=CARTESIAN_POINT('Ctrl Pts',(-202.278429738568,-65.4600289895105,
-3.93788488827538E-16));
#17518=CARTESIAN_POINT('Ctrl Pts',(-202.277545413196,-65.4440180689878,
-4.83296287894591E-16));
#17519=CARTESIAN_POINT('Ctrl Pts',(-202.276803684951,-65.4279899164929,
-4.71844785465692E-16));
#17520=CARTESIAN_POINT('Ctrl Pts',(-202.276227068944,-65.4155297070277,
-4.62942441979656E-16));
#17521=CARTESIAN_POINT('Ctrl Pts',(-202.275736729878,-65.4030602298859,
-7.24983344813615E-16));
#17522=CARTESIAN_POINT('Ctrl Pts',(-202.2753327434,-65.3905923140717,-7.21644966006352E-16));
#17523=CARTESIAN_POINT('Ctrl Pts',(-202.272313671571,-65.2974170829925,
-6.96696592803443E-16));
#17524=CARTESIAN_POINT('Ctrl Pts',(-202.2741053936,-65.2041782507755,-5.18105779583049E-16));
#17525=CARTESIAN_POINT('Ctrl Pts',(-202.280568206079,-65.1112502594295,
-6.10622663543836E-16));
#17526=CARTESIAN_POINT('Ctrl Pts',(-202.287044515393,-65.0181281987396,
-7.03332758298409E-16));
#17527=CARTESIAN_POINT('Ctrl Pts',(-202.298211829298,-64.9253172978478,
-8.84079863654896E-16));
#17528=CARTESIAN_POINT('Ctrl Pts',(-202.313980641549,-64.8332063229902,
-8.04911692853238E-16));
#17529=CARTESIAN_POINT('Ctrl Pts',(-202.32952814569,-64.7423880837798,-7.26854611329152E-16));
#17530=CARTESIAN_POINT('Ctrl Pts',(-202.349549362971,-64.6522494151919,
-6.30136933924858E-16));
#17531=CARTESIAN_POINT('Ctrl Pts',(-202.374001579135,-64.5631880635913,
-6.10622663543836E-16));
#17532=CARTESIAN_POINT('Ctrl Pts',(-202.383514240645,-64.5285404682246,
-6.03031014283114E-16));
#17533=CARTESIAN_POINT('Ctrl Pts',(-202.393697939845,-64.4940562580039,
-8.08693639224482E-16));
#17534=CARTESIAN_POINT('Ctrl Pts',(-202.404551732242,-64.4597603152699,
-8.32667268468867E-16));
#17535=CARTESIAN_POINT('Ctrl Pts',(-202.410350756828,-64.4414364881864,
-8.45476032474648E-16));
#17536=CARTESIAN_POINT('Ctrl Pts',(-202.416341081224,-64.4231664197207,
-4.41954415849099E-16));
#17537=CARTESIAN_POINT('Ctrl Pts',(-202.422522657021,-64.4049540190092,
-4.44089209850063E-16));
#17538=CARTESIAN_POINT('Ctrl Pts',(-202.428041258764,-64.3886948984179,
-4.45995047177558E-16));
#17539=CARTESIAN_POINT('Ctrl Pts',(-202.433712830842,-64.3724804931878,
-1.04911529577836E-15));
#17540=CARTESIAN_POINT('Ctrl Pts',(-202.439531012802,-64.3563305530537,
-1.08246744900953E-15));
#17541=CARTESIAN_POINT('Ctrl Pts',(-202.47036464237,-64.2707434615647,-1.25921818407324E-15));
#17542=CARTESIAN_POINT('Ctrl Pts',(-202.505348632287,-64.1868546674516,
-1.34967217968898E-15));
#17543=CARTESIAN_POINT('Ctrl Pts',(-202.544418706298,-64.105044870123,-9.99200722162641E-16));
#17544=CARTESIAN_POINT('Ctrl Pts',(-202.57588160692,-64.0391639218935,-7.16968120406447E-16));
#17545=CARTESIAN_POINT('Ctrl Pts',(-202.60999524185,-63.9746315046024,-1.14052024783077E-15));
#17546=CARTESIAN_POINT('Ctrl Pts',(-202.646744245718,-63.911664139129,-1.38777878078145E-15));
#17547=CARTESIAN_POINT('Ctrl Pts',(-202.661986529103,-63.8855473379223,
-1.49033352327672E-15));
#17548=CARTESIAN_POINT('Ctrl Pts',(-202.677682360038,-63.859699991663,-9.26822014599923E-16));
#17549=CARTESIAN_POINT('Ctrl Pts',(-202.693831375288,-63.8341385429959,
-9.43689570931383E-16));
#17550=CARTESIAN_POINT('Ctrl Pts',(-202.702298017956,-63.8207371281978,
-9.52532931962022E-16));
#17551=CARTESIAN_POINT('Ctrl Pts',(-202.710887811084,-63.8074166610173,
-1.22761254702973E-15));
#17552=CARTESIAN_POINT('Ctrl Pts',(-202.719595895668,-63.7941863862979,
-1.22124532708767E-15));
#17553=CARTESIAN_POINT('Ctrl Pts',(-202.767005235546,-63.7221569308133,
-1.18658033372179E-15));
#17554=CARTESIAN_POINT('Ctrl Pts',(-202.817957036884,-63.6527358475527,
-4.93484857439899E-16));
#17555=CARTESIAN_POINT('Ctrl Pts',(-202.872414575612,-63.5862784909644,
-5.55111512312578E-16));
#17556=CARTESIAN_POINT('Ctrl Pts',(-202.92687211434,-63.5198211343761,-6.16738167185258E-16));
#17557=CARTESIAN_POINT('Ctrl Pts',(-202.984835721377,-63.4563268124908,
-5.65027584124604E-16));
#17558=CARTESIAN_POINT('Ctrl Pts',(-203.046298166971,-63.3961948799941,
-6.66133814775094E-16));
#17559=CARTESIAN_POINT('Ctrl Pts',(-203.058348982186,-63.3844049357444,
-6.85768708283518E-16));
#17560=CARTESIAN_POINT('Ctrl Pts',(-203.070534385631,-63.3727444059762,
-1.54261645251009E-16));
#17561=CARTESIAN_POINT('Ctrl Pts',(-203.082851793447,-63.3612143523573,
-1.66533453693773E-16));
#17562=CARTESIAN_POINT('Origin',(-205.,-65.,9.));
#17563=CARTESIAN_POINT('Origin',(-205.,65.,17.));
#17564=CARTESIAN_POINT('Ctrl Pts',(-203.086534003335,66.6359872033749,17.));
#17565=CARTESIAN_POINT('Ctrl Pts',(-203.024405959645,66.5776020979941,17.));
#17566=CARTESIAN_POINT('Ctrl Pts',(-202.965656494088,66.5159622835985,17.));
#17567=CARTESIAN_POINT('Ctrl Pts',(-202.910296236763,66.4514444609274,17.));
#17568=CARTESIAN_POINT('Ctrl Pts',(-202.853578930092,66.3853451089548,17.));
#17569=CARTESIAN_POINT('Ctrl Pts',(-202.800418561819,66.3162244307376,17.));
#17570=CARTESIAN_POINT('Ctrl Pts',(-202.750855500683,66.2444412342179,17.));
#17571=CARTESIAN_POINT('Ctrl Pts',(-202.737942217452,66.2257386616427,17.));
#17572=CARTESIAN_POINT('Ctrl Pts',(-202.725273298507,66.2068551349331,17.));
#17573=CARTESIAN_POINT('Ctrl Pts',(-202.71284983158,66.1877965690358,17.));
#17574=CARTESIAN_POINT('Ctrl Pts',(-202.702648131353,66.1721463663022,17.));
#17575=CARTESIAN_POINT('Ctrl Pts',(-202.692611475546,66.1563771828948,17.));
#17576=CARTESIAN_POINT('Ctrl Pts',(-202.682749390262,66.1405070166588,17.));
#17577=CARTESIAN_POINT('Ctrl Pts',(-202.635317887944,66.064179768932,17.));
#17578=CARTESIAN_POINT('Ctrl Pts',(-202.59187115121,65.9854441421124,17.));
#17579=CARTESIAN_POINT('Ctrl Pts',(-202.552442406189,65.9046931376478,17.));
#17580=CARTESIAN_POINT('Ctrl Pts',(-202.520315548909,65.838896572369,17.));
#17581=CARTESIAN_POINT('Ctrl Pts',(-202.49085676949,65.7717608847253,17.));
#17582=CARTESIAN_POINT('Ctrl Pts',(-202.464101805081,65.7034802673812,17.));
#17583=CARTESIAN_POINT('Ctrl Pts',(-202.455215975848,65.6808029841515,17.));
#17584=CARTESIAN_POINT('Ctrl Pts',(-202.44662852597,65.6579992976328,17.));
#17585=CARTESIAN_POINT('Ctrl Pts',(-202.438341197581,65.635076009318,17.));
#17586=CARTESIAN_POINT('Ctrl Pts',(-202.431659305257,65.6165934613812,17.));
#17587=CARTESIAN_POINT('Ctrl Pts',(-202.425171725505,65.5980304421231,17.));
#17588=CARTESIAN_POINT('Ctrl Pts',(-202.418887047983,65.5794139527973,17.));
#17589=CARTESIAN_POINT('Ctrl Pts',(-202.38936981961,65.4919779363867,17.));
#17590=CARTESIAN_POINT('Ctrl Pts',(-202.364286281244,65.4032613105746,17.));
#17591=CARTESIAN_POINT('Ctrl Pts',(-202.343667590228,65.3136623471474,17.));
#17592=CARTESIAN_POINT('Ctrl Pts',(-202.322591143159,65.2220741949864,17.));
#17593=CARTESIAN_POINT('Ctrl Pts',(-202.306179437392,65.12956330341,17.));
#17594=CARTESIAN_POINT('Ctrl Pts',(-202.294508583617,65.0365211410702,17.));
#17595=CARTESIAN_POINT('Ctrl Pts',(-202.283004950542,64.9448120924728,17.));
#17596=CARTESIAN_POINT('Ctrl Pts',(-202.276106995875,64.8525859269892,17.));
#17597=CARTESIAN_POINT('Ctrl Pts',(-202.273934698214,64.7601983422578,17.));
#17598=CARTESIAN_POINT('Ctrl Pts',(-202.272809661586,64.7123506560533,17.));
#17599=CARTESIAN_POINT('Ctrl Pts',(-202.272952952458,64.6644594453727,17.));
#17600=CARTESIAN_POINT('Ctrl Pts',(-202.27438671825,64.6165733453971,17.));
#17601=CARTESIAN_POINT('Ctrl Pts',(-202.275036414498,64.5948742508328,17.));
#17602=CARTESIAN_POINT('Ctrl Pts',(-202.275951668491,64.5731691349364,17.));
#17603=CARTESIAN_POINT('Ctrl Pts',(-202.277132318497,64.5515006305554,17.));
#17604=CARTESIAN_POINT('Ctrl Pts',(-202.282342225116,64.4558830606592,17.));
#17605=CARTESIAN_POINT('Ctrl Pts',(-202.292716069493,64.3608730697258,17.));
#17606=CARTESIAN_POINT('Ctrl Pts',(-202.308320883029,64.2668677599894,17.));
#17607=CARTESIAN_POINT('Ctrl Pts',(-202.312169901591,64.2436808003145,17.));
#17608=CARTESIAN_POINT('Ctrl Pts',(-202.316337397629,64.2205548712098,17.));
#17609=CARTESIAN_POINT('Ctrl Pts',(-202.320824840019,64.1974957764614,17.));
#17610=CARTESIAN_POINT('Ctrl Pts',(-202.33832966782,64.1075457675858,17.));
#17611=CARTESIAN_POINT('Ctrl Pts',(-202.360698767987,64.0186128346896,17.));
#17612=CARTESIAN_POINT('Ctrl Pts',(-202.387628946164,63.9309270453222,17.));
#17613=CARTESIAN_POINT('Ctrl Pts',(-202.415161416494,63.8412801674492,17.));
#17614=CARTESIAN_POINT('Ctrl Pts',(-202.447461481234,63.7529361397536,17.));
#17615=CARTESIAN_POINT('Ctrl Pts',(-202.484259321795,63.6661452513196,17.));
#17616=CARTESIAN_POINT('Ctrl Pts',(-202.498888428792,63.6316412376634,17.));
#17617=CARTESIAN_POINT('Ctrl Pts',(-202.514228975924,63.5973828031145,17.));
#17618=CARTESIAN_POINT('Ctrl Pts',(-202.530266183054,63.5633862551367,17.));
#17619=CARTESIAN_POINT('Ctrl Pts',(-202.538262705644,63.546434789606,17.));
#17620=CARTESIAN_POINT('Ctrl Pts',(-202.546434285539,63.5295449770387,17.));
#17621=CARTESIAN_POINT('Ctrl Pts',(-202.554766777349,63.5127432414087,17.));
#17622=CARTESIAN_POINT('Ctrl Pts',(-202.597561732177,63.426450985303,17.));
#17623=CARTESIAN_POINT('Ctrl Pts',(-202.644651926136,63.3423600645501,17.));
#17624=CARTESIAN_POINT('Ctrl Pts',(-202.695691913412,63.2607170650344,17.));
#17625=CARTESIAN_POINT('Ctrl Pts',(-202.747749229102,63.17744675823,17.));
#17626=CARTESIAN_POINT('Ctrl Pts',(-202.803915679762,63.0967221624598,17.));
#17627=CARTESIAN_POINT('Ctrl Pts',(-202.863879846291,63.0188121011017,17.));
#17628=CARTESIAN_POINT('Ctrl Pts',(-202.92434189817,62.9402551487678,17.));
#17629=CARTESIAN_POINT('Ctrl Pts',(-202.98866545666,62.8645588312244,17.));
#17630=CARTESIAN_POINT('Ctrl Pts',(-203.056580646588,62.7920181029229,17.));
#17631=CARTESIAN_POINT('Ctrl Pts',(-203.094626893211,62.7513806189939,17.));
#17632=CARTESIAN_POINT('Ctrl Pts',(-203.133801134145,62.71173385957,17.));
#17633=CARTESIAN_POINT('Ctrl Pts',(-203.174061757578,62.673133821284,17.));
#17634=CARTESIAN_POINT('Ctrl Pts',(-203.185603246106,62.6620683716942,17.));
#17635=CARTESIAN_POINT('Ctrl Pts',(-203.197234036914,62.6510889631318,17.));
#17636=CARTESIAN_POINT('Ctrl Pts',(-203.208953206155,62.6401969707666,17.));
#17637=CARTESIAN_POINT('Ctrl Pts',(-203.219358434025,62.6305261775393,17.));
#17638=CARTESIAN_POINT('Ctrl Pts',(-203.229830124301,62.6209273315836,17.));
#17639=CARTESIAN_POINT('Ctrl Pts',(-203.240361443976,62.6114066232139,17.));
#17640=CARTESIAN_POINT('Ctrl Pts',(-203.316072000031,62.5429614380971,17.));
#17641=CARTESIAN_POINT('Ctrl Pts',(-203.394951774449,62.4784678301501,17.));
#17642=CARTESIAN_POINT('Ctrl Pts',(-203.476670244702,62.4182049299063,17.));
#17643=CARTESIAN_POINT('Ctrl Pts',(-203.558481705369,62.3578734543199,17.));
#17644=CARTESIAN_POINT('Ctrl Pts',(-203.643138907573,62.3017814875231,17.));
#17645=CARTESIAN_POINT('Ctrl Pts',(-203.730355413283,62.2502350560919,17.));
#17646=CARTESIAN_POINT('Ctrl Pts',(-203.815753129695,62.1997635599272,17.));
#17647=CARTESIAN_POINT('Ctrl Pts',(-203.903605194206,62.1536493286983,17.));
#17648=CARTESIAN_POINT('Ctrl Pts',(-203.99367653385,62.1122153753288,17.));
#17649=CARTESIAN_POINT('Ctrl Pts',(-204.044060613228,62.0890380627258,17.));
#17650=CARTESIAN_POINT('Ctrl Pts',(-204.095139669776,62.0673259342666,17.));
#17651=CARTESIAN_POINT('Ctrl Pts',(-204.146876157629,62.0471417471569,17.));
#17652=CARTESIAN_POINT('Ctrl Pts',(-204.165972597182,62.0396915678916,17.));
#17653=CARTESIAN_POINT('Ctrl Pts',(-204.185158628751,62.0324496078491,17.));
#17654=CARTESIAN_POINT('Ctrl Pts',(-204.204431285565,62.0254151804089,17.));
#17655=CARTESIAN_POINT('Ctrl Pts',(-205.793799282533,62.0307770462544,17.));
#17656=CARTESIAN_POINT('Ctrl Pts',(-205.888627163302,62.0654655086331,17.));
#17657=CARTESIAN_POINT('Ctrl Pts',(-205.98140929384,62.1051486930793,17.));
#17658=CARTESIAN_POINT('Ctrl Pts',(-206.071905809173,62.1495050655195,17.));
#17659=CARTESIAN_POINT('Ctrl Pts',(-206.163687726546,62.1944914707457,17.));
#17660=CARTESIAN_POINT('Ctrl Pts',(-206.253119305857,62.2442854648945,17.));
#17661=CARTESIAN_POINT('Ctrl Pts',(-206.339916279455,62.2985923241862,17.));
#17662=CARTESIAN_POINT('Ctrl Pts',(-206.364296640601,62.3138465523854,17.));
#17663=CARTESIAN_POINT('Ctrl Pts',(-206.388468896561,62.329457048441,17.));
#17664=CARTESIAN_POINT('Ctrl Pts',(-206.412426161583,62.3454177286137,17.));
#17665=CARTESIAN_POINT('Ctrl Pts',(-206.431863584532,62.3583672239246,17.));
#17666=CARTESIAN_POINT('Ctrl Pts',(-206.451161692209,62.3715489324215,17.));
#17667=CARTESIAN_POINT('Ctrl Pts',(-206.470297259089,62.3849456542333,17.));
#17668=CARTESIAN_POINT('Ctrl Pts',(-206.553008850231,62.4428516563967,17.));
#17669=CARTESIAN_POINT('Ctrl Pts',(-206.632764575627,62.5048222618196,17.));
#17670=CARTESIAN_POINT('Ctrl Pts',(-206.709299005451,62.5705587218441,17.));
#17671=CARTESIAN_POINT('Ctrl Pts',(-206.768827177178,62.621688276087,17.));
#17672=CARTESIAN_POINT('Ctrl Pts',(-206.826405951603,62.6750969629653,17.));
#17673=CARTESIAN_POINT('Ctrl Pts',(-206.88189230934,62.7306563357683,17.));
#17674=CARTESIAN_POINT('Ctrl Pts',(-206.912069704626,62.760873441797,17.));
#17675=CARTESIAN_POINT('Ctrl Pts',(-206.941627879906,62.7917268692334,17.));
#17676=CARTESIAN_POINT('Ctrl Pts',(-206.970541572236,62.8231968742563,17.));
#17677=CARTESIAN_POINT('Ctrl Pts',(-206.982346396854,62.8360453851206,17.));
#17678=CARTESIAN_POINT('Ctrl Pts',(-206.994038687849,62.8489912085626,17.));
#17679=CARTESIAN_POINT('Ctrl Pts',(-207.005612070685,62.8620271047964,17.));
#17680=CARTESIAN_POINT('Ctrl Pts',(-207.071011765377,62.9356912741935,17.));
#17681=CARTESIAN_POINT('Ctrl Pts',(-207.132669287851,63.0122850945349,17.));
#17682=CARTESIAN_POINT('Ctrl Pts',(-207.190339507946,63.0915302946758,17.));
#17683=CARTESIAN_POINT('Ctrl Pts',(-207.247552291736,63.1701469272205,17.));
#17684=CARTESIAN_POINT('Ctrl Pts',(-207.300841218128,63.2513738284823,17.));
#17685=CARTESIAN_POINT('Ctrl Pts',(-207.349920642778,63.3349611348081,17.));
#17686=CARTESIAN_POINT('Ctrl Pts',(-207.397481392412,63.4159619814392,17.));
#17687=CARTESIAN_POINT('Ctrl Pts',(-207.441089305762,63.4991801155586,17.));
#17688=CARTESIAN_POINT('Ctrl Pts',(-207.480436533273,63.5843978591788,17.));
#17689=CARTESIAN_POINT('Ctrl Pts',(-207.501052452161,63.629047563909,17.));
#17690=CARTESIAN_POINT('Ctrl Pts',(-207.520497896918,63.6742463055229,17.));
#17691=CARTESIAN_POINT('Ctrl Pts',(-207.538722823233,63.7199629468458,17.));
#17692=CARTESIAN_POINT('Ctrl Pts',(-207.545019377446,63.7357576505121,17.));
#17693=CARTESIAN_POINT('Ctrl Pts',(-207.551170208915,63.7516141714125,17.));
#17694=CARTESIAN_POINT('Ctrl Pts',(-207.557173136494,63.7675312180113,17.));
#17695=CARTESIAN_POINT('Ctrl Pts',(-207.562735096129,63.7822790172345,17.));
#17696=CARTESIAN_POINT('Ctrl Pts',(-207.568167313965,63.7970715617822,17.));
#17697=CARTESIAN_POINT('Ctrl Pts',(-207.573465961202,63.8119004887879,17.));
#17698=CARTESIAN_POINT('Ctrl Pts',(-207.604700101148,63.8993131359471,17.));
#17699=CARTESIAN_POINT('Ctrl Pts',(-207.631326724125,63.9880676646163,17.));
#17700=CARTESIAN_POINT('Ctrl Pts',(-207.653093596572,64.0779404437609,17.));
#17701=CARTESIAN_POINT('Ctrl Pts',(-207.658254733772,64.0992501539593,17.));
#17702=CARTESIAN_POINT('Ctrl Pts',(-207.663142425011,64.1206227749284,17.));
#17703=CARTESIAN_POINT('Ctrl Pts',(-207.667752876821,64.1420553867836,17.));
#17704=CARTESIAN_POINT('Ctrl Pts',(-207.687563068899,64.2341470461388,17.));
#17705=CARTESIAN_POINT('Ctrl Pts',(-207.702258853542,64.3273466761675,17.));
#17706=CARTESIAN_POINT('Ctrl Pts',(-207.711951692842,64.4212621179871,17.));
#17707=CARTESIAN_POINT('Ctrl Pts',(-207.722120103753,64.5197854478193,17.));
#17708=CARTESIAN_POINT('Ctrl Pts',(-207.726782615872,64.6190978352621,17.));
#17709=CARTESIAN_POINT('Ctrl Pts',(-207.726009639275,64.718730548459,17.));
#17710=CARTESIAN_POINT('Ctrl Pts',(-207.725769558652,64.7496757076122,17.));
#17711=CARTESIAN_POINT('Ctrl Pts',(-207.725004722666,64.7806515775433,17.));
#17712=CARTESIAN_POINT('Ctrl Pts',(-207.723716174804,64.8116435095492,17.));
#17713=CARTESIAN_POINT('Ctrl Pts',(-207.723127503835,64.8258021226421,17.));
#17714=CARTESIAN_POINT('Ctrl Pts',(-207.722429444061,64.8399641697794,17.));
#17715=CARTESIAN_POINT('Ctrl Pts',(-207.721623107401,64.8541137317494,17.));
#17716=CARTESIAN_POINT('Ctrl Pts',(-207.716331548034,64.9469697940972,17.));
#17717=CARTESIAN_POINT('Ctrl Pts',(-207.706375553367,65.0394451487277,17.));
#17718=CARTESIAN_POINT('Ctrl Pts',(-207.691882946519,65.131168594172,17.));
#17719=CARTESIAN_POINT('Ctrl Pts',(-207.677420973782,65.2226981568877,17.));
#17720=CARTESIAN_POINT('Ctrl Pts',(-207.658441130303,65.3134799320582,17.));
#17721=CARTESIAN_POINT('Ctrl Pts',(-207.635021707819,65.4031281056214,17.));
#17722=CARTESIAN_POINT('Ctrl Pts',(-207.611997363202,65.4912639443185,17.));
#17723=CARTESIAN_POINT('Ctrl Pts',(-207.584681489474,65.578304892392,17.));
#17724=CARTESIAN_POINT('Ctrl Pts',(-207.553108104886,65.6638552077799,17.));
#17725=CARTESIAN_POINT('Ctrl Pts',(-207.536805169438,65.708029162759,17.));
#17726=CARTESIAN_POINT('Ctrl Pts',(-207.519366485957,65.7518051379706,17.));
#17727=CARTESIAN_POINT('Ctrl Pts',(-207.500793026226,65.7951245042335,17.));
#17728=CARTESIAN_POINT('Ctrl Pts',(-207.49498264897,65.8086761991856,17.));
#17729=CARTESIAN_POINT('Ctrl Pts',(-207.489060429026,65.822184902516,17.));
#17730=CARTESIAN_POINT('Ctrl Pts',(-207.483028782271,65.8356433357431,17.));
#17731=CARTESIAN_POINT('Ctrl Pts',(-207.446484708349,65.9171842479814,17.));
#17732=CARTESIAN_POINT('Ctrl Pts',(-207.406050922741,65.9966090453918,17.));
#17733=CARTESIAN_POINT('Ctrl Pts',(-207.361807140979,66.0735724370544,17.));
#17734=CARTESIAN_POINT('Ctrl Pts',(-207.318274246064,66.149299219623,17.));
#17735=CARTESIAN_POINT('Ctrl Pts',(-207.271052339791,66.2226437477733,17.));
#17736=CARTESIAN_POINT('Ctrl Pts',(-207.220180215582,66.2932441543424,17.));
#17737=CARTESIAN_POINT('Ctrl Pts',(-207.170937073537,66.3615838571394,17.));
#17738=CARTESIAN_POINT('Ctrl Pts',(-207.118273276478,66.4273528076824,17.));
#17739=CARTESIAN_POINT('Ctrl Pts',(-207.06219578552,66.4901836495188,17.));
#17740=CARTESIAN_POINT('Ctrl Pts',(-207.027350691367,66.5292251002338,17.));
#17741=CARTESIAN_POINT('Ctrl Pts',(-206.991187020073,66.5671313315531,17.));
#17742=CARTESIAN_POINT('Ctrl Pts',(-206.953701799746,66.6038050912543,17.));
#17743=CARTESIAN_POINT('Ctrl Pts',(-206.941652995692,66.6155930690407,17.));
#17744=CARTESIAN_POINT('Ctrl Pts',(-206.929467627116,66.6272536523146,17.));
#17745=CARTESIAN_POINT('Ctrl Pts',(-206.917148172614,66.6387856228502,17.));
#17746=CARTESIAN_POINT('Origin',(-205.,65.,-2.20842344717744));
#17747=CARTESIAN_POINT('Ctrl Pts',(-201.923731627295,65.0022750736124,0.291576552822547));
#17748=CARTESIAN_POINT('Ctrl Pts',(-201.922496052185,65.1502516884003,0.299259877064296));
#17749=CARTESIAN_POINT('Ctrl Pts',(-201.999549699837,66.317125995226,0.359912640907481));
#17750=CARTESIAN_POINT('Ctrl Pts',(-203.493276988919,68.3070967035895,0.473534844352101));
#17751=CARTESIAN_POINT('Ctrl Pts',(-206.96385777596,68.0574739600344,0.632443163156408));
#17752=CARTESIAN_POINT('Ctrl Pts',(-208.633920120295,65.0051924190987,0.791351481960715));
#17753=CARTESIAN_POINT('Ctrl Pts',(-206.972481828636,61.9479566315291,0.95025980076502));
#17754=CARTESIAN_POINT('Ctrl Pts',(-203.502676407862,61.6888942785303,1.10916811956933));
#17755=CARTESIAN_POINT('Ctrl Pts',(-202.001256849451,63.6767448554868,1.22294037025517));
#17756=CARTESIAN_POINT('Ctrl Pts',(-201.922527685932,64.8467465056595,1.28374318133958));
#17757=CARTESIAN_POINT('Ctrl Pts',(-201.923803965215,64.9976529174956,1.29157655282255));
#17758=CARTESIAN_POINT('Ctrl Pts',(-201.929611540575,64.9968423971894,0.208423447177456));
#17759=CARTESIAN_POINT('Ctrl Pts',(-201.934956993548,65.702126874876,0.244887843987842));
#17760=CARTESIAN_POINT('Ctrl Pts',(-202.52503086706,67.4423464487146,0.334321680399663));
#17761=CARTESIAN_POINT('Ctrl Pts',(-205.417645976078,68.6092463233164,0.47672495641292));
#17762=CARTESIAN_POINT('Ctrl Pts',(-208.260115679803,66.6049913509854,0.635633275217227));
#17763=CARTESIAN_POINT('Ctrl Pts',(-208.114970174343,63.128085617879,0.794541594021532));
#17764=CARTESIAN_POINT('Ctrl Pts',(-205.113461133577,61.3679192540746,0.95344991282584));
#17765=CARTESIAN_POINT('Ctrl Pts',(-202.417561343649,62.7304356237314,1.09141053054448));
#17766=CARTESIAN_POINT('Ctrl Pts',(-201.93359519178,64.3813018489966,1.17640170866169));
#17767=CARTESIAN_POINT('Ctrl Pts',(-201.930557054308,65.0016530359719,1.20842344717746));
#17768=CARTESIAN_POINT('Ctrl Pts',(-206.913465996665,66.6359872033749,0.));
#17769=CARTESIAN_POINT('Ctrl Pts',(-207.457950030113,65.9991535645904,0.0529694396014356));
#17770=CARTESIAN_POINT('Ctrl Pts',(-207.850661636903,64.1491413375017,0.158908318804307));
#17771=CARTESIAN_POINT('Ctrl Pts',(-205.826538235528,62.1387920084224,0.317816637608613));
#17772=CARTESIAN_POINT('Ctrl Pts',(-203.043492655661,62.757459158079,0.47672495641292));
#17773=CARTESIAN_POINT('Ctrl Pts',(-202.054683559188,65.4291982286823,0.635633275217226));
#17774=CARTESIAN_POINT('Ctrl Pts',(-203.76584506901,67.7088387672967,0.794541594021534));
#17775=CARTESIAN_POINT('Ctrl Pts',(-206.608593444275,67.504373090739,0.953449912825839));
#17776=CARTESIAN_POINT('Ctrl Pts',(-207.976539418527,65.0042531039795,1.11235823163015));
#17777=CARTESIAN_POINT('Ctrl Pts',(-206.615657395019,62.500075100008,1.27126655043445));
#17778=CARTESIAN_POINT('Ctrl Pts',(-203.773544121293,62.2878774511794,1.43017486923876));
#17779=CARTESIAN_POINT('Ctrl Pts',(-202.055838985475,64.5620859668133,1.58908318804307));
#17780=CARTESIAN_POINT('Ctrl Pts',(-203.037304314461,67.237787377709,1.74799150684737));
#17781=CARTESIAN_POINT('Ctrl Pts',(-205.818148785739,67.8619014891644,1.90689982565168));
#17782=CARTESIAN_POINT('Ctrl Pts',(-207.848922781157,65.8622605977419,2.06580814445599));
#17783=CARTESIAN_POINT('Ctrl Pts',(-207.267836607737,63.0721067410292,2.22471646326029));
#17784=CARTESIAN_POINT('Ctrl Pts',(-204.607622987557,62.0494248900596,2.3836247820646));
#17785=CARTESIAN_POINT('Ctrl Pts',(-202.307136320099,63.7317968295565,2.54253310086891));
#17786=CARTESIAN_POINT('Ctrl Pts',(-202.475436931506,66.57684350044,2.70144141967321));
#17787=CARTESIAN_POINT('Ctrl Pts',(-204.958228769587,67.9762575579951,2.86034973847752));
#17788=CARTESIAN_POINT('Ctrl Pts',(-207.479315994157,66.6470720078308,3.01925805728183));
#17789=CARTESIAN_POINT('Ctrl Pts',(-207.727394031276,63.8078692224566,3.17816637608614));
#17790=CARTESIAN_POINT('Ctrl Pts',(-205.475027701519,62.0615986230515,3.33707469489044));
#17791=CARTESIAN_POINT('Ctrl Pts',(-202.787161285521,63.0092215576596,3.49598301369475));
#17792=CARTESIAN_POINT('Ctrl Pts',(-202.128000669921,65.7819679208284,3.65489133249905));
#17793=CARTESIAN_POINT('Ctrl Pts',(-204.101856940684,67.8378148325493,3.81379965130336));
#17794=CARTESIAN_POINT('Ctrl Pts',(-206.899120729728,67.2919848242,3.97270797010767));
#17795=CARTESIAN_POINT('Ctrl Pts',(-207.955291859906,64.6448887457045,4.13161628891197));
#17796=CARTESIAN_POINT('Ctrl Pts',(-206.302084443574,62.323354696317,4.29052460771628));
#17797=CARTESIAN_POINT('Ctrl Pts',(-203.455140562519,62.4557391449499,4.44943292652058));
#17798=CARTESIAN_POINT('Ctrl Pts',(-202.024506547164,64.9206735088564,4.60834124532489));
#17799=CARTESIAN_POINT('Ctrl Pts',(-203.321771672898,67.4583335132076,4.7672495641292));
#17800=CARTESIAN_POINT('Ctrl Pts',(-206.157617771706,67.7422208289451,4.92615788293351));
#17801=CARTESIAN_POINT('Ctrl Pts',(-207.93217283587,65.5120707379364,5.08506620173782));
#17802=CARTESIAN_POINT('Ctrl Pts',(-207.018544616397,62.8124599176985,5.24397452054212));
#17803=CARTESIAN_POINT('Ctrl Pts',(-204.254337253468,62.1183613952304,5.40288283934643));
#17804=CARTESIAN_POINT('Ctrl Pts',(-202.173745162441,64.0661169381366,5.56179115815074));
#17805=CARTESIAN_POINT('Ctrl Pts',(-202.684231918022,66.870046034341,5.72069947695504));
#17806=CARTESIAN_POINT('Ctrl Pts',(-205.3177889683,67.9595378273796,5.87960779575935));
#17807=CARTESIAN_POINT('Ctrl Pts',(-207.660000644302,66.3357584184189,6.03851611456366));
#17808=CARTESIAN_POINT('Ctrl Pts',(-207.563553459886,63.4873706209475,6.19742443336795));
#17809=CARTESIAN_POINT('Ctrl Pts',(-205.116869115753,62.0257445318455,6.35633275217228));
#17810=CARTESIAN_POINT('Ctrl Pts',(-202.56304047252,63.2908826133093,6.51524107097657));
#17811=CARTESIAN_POINT('Ctrl Pts',(-202.243389086688,66.1229204124393,6.67414938978089));
#17812=CARTESIAN_POINT('Ctrl Pts',(-204.45096777611,67.9254773280944,6.83305770858519));
#17813=CARTESIAN_POINT('Ctrl Pts',(-207.161893071975,67.0459893268077,6.99196602738949));
#17814=CARTESIAN_POINT('Ctrl Pts',(-207.890818962485,64.2907611783034,7.1508743461938));
#17815=CARTESIAN_POINT('Ctrl Pts',(-205.969474338275,62.185755254515,7.30978266499811));
#17816=CARTESIAN_POINT('Ctrl Pts',(-203.159326476349,62.6608174591554,7.46869098380242));
#17817=CARTESIAN_POINT('Ctrl Pts',(-202.036687528078,65.2804160726826,7.62759930260672));
#17818=CARTESIAN_POINT('Ctrl Pts',(-203.630780333736,67.6429323649268,7.78650762141104));
#17819=CARTESIAN_POINT('Ctrl Pts',(-206.480158425938,67.5824378045147,7.94541594021533));
#17820=CARTESIAN_POINT('Ctrl Pts',(-207.972543816666,65.154393128297,8.10432425901965));
#17821=CARTESIAN_POINT('Ctrl Pts',(-206.739734259782,62.5848025576766,8.26323257782394));
#17822=CARTESIAN_POINT('Ctrl Pts',(-203.91195577818,62.2294380080158,8.42214089662826));
#17823=CARTESIAN_POINT('Ctrl Pts',(-202.081684078297,64.4140937266076,8.58104921543256));
#17824=CARTESIAN_POINT('Ctrl Pts',(-202.926891798018,67.1359017680923,8.73995753423687));
#17825=CARTESIAN_POINT('Ctrl Pts',(-205.672701946614,67.8995389411223,8.89886585304117));
#17826=CARTESIAN_POINT('Ctrl Pts',(-207.801786469205,66.0049112204788,9.05777417184548));
#17827=CARTESIAN_POINT('Ctrl Pts',(-207.362224471816,63.1889921245852,9.21668249064979));
#17828=CARTESIAN_POINT('Ctrl Pts',(-204.757001480761,62.0333848076113,9.37559080945409));
#17829=CARTESIAN_POINT('Ctrl Pts',(-202.3745568162,63.5975371417748,9.53449912825841));
#17830=CARTESIAN_POINT('Ctrl Pts',(-202.399089118511,66.4474517493217,9.6934074470627));
#17831=CARTESIAN_POINT('Ctrl Pts',(-204.808107447128,67.9703587709594,9.85231576586701));
#17832=CARTESIAN_POINT('Ctrl Pts',(-207.393050723475,66.7700740704675,10.0112240846713));
#17833=CARTESIAN_POINT('Ctrl Pts',(-207.784071843173,63.9470052459228,10.1701324034756));
#17834=CARTESIAN_POINT('Ctrl Pts',(-205.622687014046,62.0893102428115,10.3290407222799));
#17835=CARTESIAN_POINT('Ctrl Pts',(-202.890429690085,62.900103076913,10.4879490410842));
#17836=CARTESIAN_POINT('Ctrl Pts',(-202.092202848023,65.6360579399868,10.6468573598885));
#17837=CARTESIAN_POINT('Ctrl Pts',(-203.959811935046,67.7888819927689,10.8057656786929));
#17838=CARTESIAN_POINT('Ctrl Pts',(-206.781053814051,67.3848902053379,10.9646739974972));
#17839=CARTESIAN_POINT('Ctrl Pts',(-207.969445462805,64.7944577330778,11.1235823163015));
#17840=CARTESIAN_POINT('Ctrl Pts',(-206.435482700137,62.3924641138286,11.2824906351058));
#17841=CARTESIAN_POINT('Ctrl Pts',(-203.585485442077,62.3810302511319,11.4413989539101));
#17842=CARTESIAN_POINT('Ctrl Pts',(-202.032299320984,64.770638582514,11.6003072727144));
#17843=CARTESIAN_POINT('Ctrl Pts',(-203.199868013036,67.3705228979221,11.7592155915187));
#17844=CARTESIAN_POINT('Ctrl Pts',(-206.017777591034,67.7971383153597,11.918123910323));
#17845=CARTESIAN_POINT('Ctrl Pts',(-207.902600049061,65.6593685883118,12.0770322291273));
#17846=CARTESIAN_POINT('Ctrl Pts',(-207.12635122387,62.9170971091267,12.2359405479316));
#17847=CARTESIAN_POINT('Ctrl Pts',(-204.400687362422,62.0844077201178,12.3948488667359));
#17848=CARTESIAN_POINT('Ctrl Pts',(-202.224466628715,63.924700746336,12.5537571855402));
#17849=CARTESIAN_POINT('Ctrl Pts',(-202.592823868233,66.7508161099091,12.7126655043445));
#17850=CARTESIAN_POINT('Ctrl Pts',(-205.168053280859,67.9718028324414,12.8715738231488));
#17851=CARTESIAN_POINT('Ctrl Pts',(-207.589213323861,66.4682739333878,13.0304821419531));
#17852=CARTESIAN_POINT('Ctrl Pts',(-207.63661153071,63.6186479028593,13.1893904607575));
#17853=CARTESIAN_POINT('Ctrl Pts',(-205.26679375494,62.0354300357772,13.3482987795618));
#17854=CARTESIAN_POINT('Ctrl Pts',(-202.652382446799,63.1700967777672,13.5072070983661));
#17855=CARTESIAN_POINT('Ctrl Pts',(-202.190240672061,65.9823983409187,13.6661154171704));
#17856=CARTESIAN_POINT('Ctrl Pts',(-204.304054846181,67.8940480862733,13.8250237359747));
#17857=CARTESIAN_POINT('Ctrl Pts',(-207.055903756617,67.1524668900571,13.983932054779));
#17858=CARTESIAN_POINT('Ctrl Pts',(-207.922923086071,64.437528111351,14.1428403735833));
#17859=CARTESIAN_POINT('Ctrl Pts',(-206.110239189501,62.2382572639803,14.3017486923876));
#17860=CARTESIAN_POINT('Ctrl Pts',(-203.279700432717,62.5709213092164,14.4606570111919));
#17861=CARTESIAN_POINT('Ctrl Pts',(-202.026313051011,65.1305375083974,14.6195653299962));
#17862=CARTESIAN_POINT('Ctrl Pts',(-203.499168711792,67.5704784621524,14.7784736488005));
#17863=CARTESIAN_POINT('Ctrl Pts',(-206.347969550324,67.6538333200658,14.9373819676048));
#17864=CARTESIAN_POINT('Ctrl Pts',(-207.96096732682,65.3041838044336,15.0962902864091));
#17865=CARTESIAN_POINT('Ctrl Pts',(-206.859382619904,62.6756612501156,15.2551986052134));
#17866=CARTESIAN_POINT('Ctrl Pts',(-204.053138216533,62.1780679787958,15.4141069240178));
#17867=CARTESIAN_POINT('Ctrl Pts',(-202.114963009909,64.2675873651587,15.5730152428221));
#17868=CARTESIAN_POINT('Ctrl Pts',(-202.821763859197,67.0285808080553,15.7319235616264));
#17869=CARTESIAN_POINT('Ctrl Pts',(-205.525534104406,67.9297809896548,15.8908318804307));
#17870=CARTESIAN_POINT('Ctrl Pts',(-207.747527632094,66.1450175695412,16.049740199235));
#17871=CARTESIAN_POINT('Ctrl Pts',(-207.450562796655,63.3104595362684,16.2086485180393));
#17872=CARTESIAN_POINT('Ctrl Pts',(-204.907064123563,62.0249671649789,16.3675568368436));
#17873=CARTESIAN_POINT('Ctrl Pts',(-202.448531805715,63.4667172751089,16.5264651556479));
#17874=CARTESIAN_POINT('Ctrl Pts',(-202.329643294205,66.314646385853,16.6853734744522));
#17875=CARTESIAN_POINT('Ctrl Pts',(-204.657906700394,67.9563292425747,16.8442817932565));
#17876=CARTESIAN_POINT('Ctrl Pts',(-207.301858734717,66.8897415144046,17.0031901120608));
#17877=CARTESIAN_POINT('Ctrl Pts',(-207.831197468937,64.0864612085167,17.1620984308651));
#17878=CARTESIAN_POINT('Ctrl Pts',(-206.459639356019,62.7843106836637,17.268037310068));
#17879=CARTESIAN_POINT('Ctrl Pts',(-205.650199997975,62.567913197965,17.3210067496694));
#17880=CARTESIAN_POINT('Ctrl Pts',(-207.054331550342,66.7564253212268,-0.107002249889811));
#17881=CARTESIAN_POINT('Ctrl Pts',(-207.63889941333,66.0727092589846,-0.0540328102883751));
#17882=CARTESIAN_POINT('Ctrl Pts',(-208.060521666048,64.0865028182897,0.0519060689144961));
#17883=CARTESIAN_POINT('Ctrl Pts',(-205.88738633337,61.9281555776621,0.210814387718803));
#17884=CARTESIAN_POINT('Ctrl Pts',(-202.899458483737,62.5923677700475,0.36972270652311));
#17885=CARTESIAN_POINT('Ctrl Pts',(-201.837855231999,65.4607949470069,0.528631025327416));
#17886=CARTESIAN_POINT('Ctrl Pts',(-203.674989042313,67.9082580793944,0.687539344131723));
#17887=CARTESIAN_POINT('Ctrl Pts',(-206.72701488817,67.6887400471708,0.846447662936029));
#17888=CARTESIAN_POINT('Ctrl Pts',(-208.195666319116,65.0045662090192,1.00535598174034));
#17889=CARTESIAN_POINT('Ctrl Pts',(-206.734598872892,62.316035610515,1.16426430054464));
#17890=CARTESIAN_POINT('Ctrl Pts',(-203.683254883482,62.0882163936298,1.32317261934895));
#17891=CARTESIAN_POINT('Ctrl Pts',(-201.839095718467,64.5298476083291,1.48208093815326));
#17892=CARTESIAN_POINT('Ctrl Pts',(-202.89281456919,67.4025288251776,1.64098925695756));
#17893=CARTESIAN_POINT('Ctrl Pts',(-205.878379269006,68.0725889738351,1.79989757576187));
#17894=CARTESIAN_POINT('Ctrl Pts',(-208.058654799208,65.9257385047058,1.95880589456618));
#17895=CARTESIAN_POINT('Ctrl Pts',(-207.43479021964,62.9301790810506,2.11771421337048));
#17896=CARTESIAN_POINT('Ctrl Pts',(-204.578736973798,61.8322094301289,2.27662253217479));
#17897=CARTESIAN_POINT('Ctrl Pts',(-202.108893062102,63.6384342393193,2.4355308509791));
#17898=CARTESIAN_POINT('Ctrl Pts',(-202.289583629145,66.6929275767385,2.5944391697834));
#17899=CARTESIAN_POINT('Ctrl Pts',(-204.955153654843,68.1953637085738,2.75334748858771));
#17900=CARTESIAN_POINT('Ctrl Pts',(-207.66183829707,66.7683261668979,2.91225580739201));
#17901=CARTESIAN_POINT('Ctrl Pts',(-207.928179344933,63.7201069301938,3.07116412619632));
#17902=CARTESIAN_POINT('Ctrl Pts',(-205.509998294309,61.8452793690848,3.23007244500063));
#17903=CARTESIAN_POINT('Ctrl Pts',(-202.624256508924,62.8626644157938,3.38898076380494));
#17904=CARTESIAN_POINT('Ctrl Pts',(-201.916569802324,65.8395348409185,3.54788908260924));
#17905=CARTESIAN_POINT('Ctrl Pts',(-204.035737438403,68.0467291055579,3.70679740141355));
#17906=CARTESIAN_POINT('Ctrl Pts',(-207.038930213439,67.460716179679,3.86570572021786));
#17907=CARTESIAN_POINT('Ctrl Pts',(-208.17285455757,64.6187461627998,4.02461403902216));
#17908=CARTESIAN_POINT('Ctrl Pts',(-206.397941305624,62.1263054028582,4.18352235782647));
#17909=CARTESIAN_POINT('Ctrl Pts',(-203.3414110892,62.2684357307946,4.34243067663078));
#17910=CARTESIAN_POINT('Ctrl Pts',(-201.805456648484,64.9148336506537,4.50133899543508));
#17911=CARTESIAN_POINT('Ctrl Pts',(-203.198223847691,67.6393111276853,4.66024731423939));
#17912=CARTESIAN_POINT('Ctrl Pts',(-206.242839285253,67.9440976619002,4.8191556330437));
#17913=CARTESIAN_POINT('Ctrl Pts',(-208.148033557054,65.5497683652509,4.978063951848));
#17914=CARTESIAN_POINT('Ctrl Pts',(-207.167145848667,62.6514175759892,5.13697227065231));
#17915=CARTESIAN_POINT('Ctrl Pts',(-204.199443047964,61.9062209034394,5.29588058945662));
#17916=CARTESIAN_POINT('Ctrl Pts',(-201.965681913227,63.9973663280875,5.45478890826092));
#17917=CARTESIAN_POINT('Ctrl Pts',(-202.513749686499,67.0077150969155,5.61369722706523));
#17918=CARTESIAN_POINT('Ctrl Pts',(-205.341183958882,68.1774131047081,5.77260554586954));
#17919=CARTESIAN_POINT('Ctrl Pts',(-207.855824591105,66.4340942913934,5.93151386467385));
#17920=CARTESIAN_POINT('Ctrl Pts',(-207.752277157164,63.3760138603049,6.09042218347815));
#17921=CARTESIAN_POINT('Ctrl Pts',(-205.125472787168,61.8067857711313,6.24933050228246));
#17922=CARTESIAN_POINT('Ctrl Pts',(-202.38363636828,63.1650607970895,6.40823882108677));
#17923=CARTESIAN_POINT('Ctrl Pts',(-202.040452884397,66.2055875755397,6.56714713989107));
#17924=CARTESIAN_POINT('Ctrl Pts',(-204.410549117854,68.1408451393384,6.72605545869538));
#17925=CARTESIAN_POINT('Ctrl Pts',(-207.321047331891,67.1966109839683,6.88496377749969));
#17926=CARTESIAN_POINT('Ctrl Pts',(-208.103635293917,64.2385484295628,7.04387209630399));
#17927=CARTESIAN_POINT('Ctrl Pts',(-206.04084510717,61.9785761643475,7.2027804151083));
#17928=CARTESIAN_POINT('Ctrl Pts',(-203.02381975948,62.4886115018288,7.36168873391261));
#17929=CARTESIAN_POINT('Ctrl Pts',(-201.818534368941,65.3010597451634,7.52059705271691));
#17930=CARTESIAN_POINT('Ctrl Pts',(-203.529981110373,67.8374997790149,7.67950537152123));
#17931=CARTESIAN_POINT('Ctrl Pts',(-206.589124739718,67.7725517296137,7.83841369032552));
#17932=CARTESIAN_POINT('Ctrl Pts',(-208.191376569008,65.1657592427404,7.99732200912984));
#17933=CARTESIAN_POINT('Ctrl Pts',(-206.867810029188,62.4070005347793,8.15623032793413));
#17934=CARTESIAN_POINT('Ctrl Pts',(-203.831856130734,62.0254747551137,8.31513864673844));
#17935=CARTESIAN_POINT('Ctrl Pts',(-201.866843475521,64.3709604743062,8.47404696554275));
#17936=CARTESIAN_POINT('Ctrl Pts',(-202.774273703308,67.2931426000101,8.63295528434706));
#17937=CARTESIAN_POINT('Ctrl Pts',(-205.722224923419,68.1129972200054,8.79186360315136));
#17938=CARTESIAN_POINT('Ctrl Pts',(-208.008048405898,66.0788907820261,8.95077192195567));
#17939=CARTESIAN_POINT('Ctrl Pts',(-207.536126730185,63.0556693336245,9.10968024075997));
#17940=CARTESIAN_POINT('Ctrl Pts',(-204.739112414002,61.8149885087741,9.26858855956429));
#17941=CARTESIAN_POINT('Ctrl Pts',(-202.181276920776,63.4942906208646,9.42749687836859));
#17942=CARTESIAN_POINT('Ctrl Pts',(-202.207615242297,66.5540102627441,9.5864051971729));
#17943=CARTESIAN_POINT('Ctrl Pts',(-204.793980699773,68.1890306645911,9.7453135159772));
#17944=CARTESIAN_POINT('Ctrl Pts',(-207.569222349063,66.9003833962775,9.90422183478151));
#17945=CARTESIAN_POINT('Ctrl Pts',(-207.989029664398,63.8694858704489,10.0631301535858));
#17946=CARTESIAN_POINT('Ctrl Pts',(-205.668527991181,61.8750310630701,10.2220384723901));
#17947=CARTESIAN_POINT('Ctrl Pts',(-202.735127327647,62.745512849937,10.3809467911944));
#17948=CARTESIAN_POINT('Ctrl Pts',(-201.878136616114,65.6828832580448,10.5398551099987));
#17949=CARTESIAN_POINT('Ctrl Pts',(-203.883235362505,67.9941939276222,10.698763428803));
#17950=CARTESIAN_POINT('Ctrl Pts',(-206.912171446705,67.560461069842,10.8576717476073));
#17951=CARTESIAN_POINT('Ctrl Pts',(-208.18805012051,64.7793261209747,11.0165800664117));
#17952=CARTESIAN_POINT('Ctrl Pts',(-206.541160076009,62.2005025179714,11.175488385216));
#17953=CARTESIAN_POINT('Ctrl Pts',(-203.48135169905,62.1882269170874,11.3343967040203));
#17954=CARTESIAN_POINT('Ctrl Pts',(-201.813823110784,64.7537534520113,11.4933050228246));
#17955=CARTESIAN_POINT('Ctrl Pts',(-203.06734588331,67.5450360698843,11.6522133416289));
#17956=CARTESIAN_POINT('Ctrl Pts',(-206.092704349143,68.0030580642296,11.8111216604332));
#17957=CARTESIAN_POINT('Ctrl Pts',(-208.11628368061,65.7079099898478,11.9700299792375));
#17958=CARTESIAN_POINT('Ctrl Pts',(-207.282888963754,62.763757948938,12.1289382980418));
#17959=CARTESIAN_POINT('Ctrl Pts',(-204.356567160304,61.869767626425,12.2878466168461));
#17960=CARTESIAN_POINT('Ctrl Pts',(-202.020137392775,63.8455393580491,12.4467549356504));
#17961=CARTESIAN_POINT('Ctrl Pts',(-202.415612358234,66.8797077030384,12.6056632544547));
#17962=CARTESIAN_POINT('Ctrl Pts',(-205.180425028513,68.1905810350019,12.764571573259));
#17963=CARTESIAN_POINT('Ctrl Pts',(-207.779826049193,66.5763653345084,12.9234798920633));
#17964=CARTESIAN_POINT('Ctrl Pts',(-207.830713617579,63.5169555141125,13.0823882108676));
#17965=CARTESIAN_POINT('Ctrl Pts',(-205.286434579534,61.8171843025619,13.241296529672));
#17966=CARTESIAN_POINT('Ctrl Pts',(-202.479555520672,63.0353829490269,13.4002048484763));
#17967=CARTESIAN_POINT('Ctrl Pts',(-201.983391789395,66.0547205491346,13.5591131672806));
#17968=CARTESIAN_POINT('Ctrl Pts',(-204.252820750779,68.1071021393641,13.7180214860849));
#17969=CARTESIAN_POINT('Ctrl Pts',(-207.207255294343,67.3109272132444,13.8769298048892));
#17970=CARTESIAN_POINT('Ctrl Pts',(-208.138102859107,64.3961200517564,14.0358381236935));
#17971=CARTESIAN_POINT('Ctrl Pts',(-206.191972786239,62.034943267128,14.1947464424978));
#17972=CARTESIAN_POINT('Ctrl Pts',(-203.153055406645,62.3920973764689,14.3536547613021));
#17973=CARTESIAN_POINT('Ctrl Pts',(-201.807396143545,65.1401474196413,14.5125630801064));
#17974=CARTESIAN_POINT('Ctrl Pts',(-203.388680503087,67.7597119642983,14.6714713989107));
#17975=CARTESIAN_POINT('Ctrl Pts',(-206.447204382496,67.8492032407486,14.830379717715));
#17976=CARTESIAN_POINT('Ctrl Pts',(-208.178947841049,65.3265772099636,14.9892880365193));
#17977=CARTESIAN_POINT('Ctrl Pts',(-206.996266663157,62.5045480630999,15.1481963553236));
#17978=CARTESIAN_POINT('Ctrl Pts',(-203.983432138862,61.9703229667084,15.3071046741279));
#17979=CARTESIAN_POINT('Ctrl Pts',(-201.902572335763,64.2136686064732,15.4660129929322));
#17980=CARTESIAN_POINT('Ctrl Pts',(-202.66140645512,67.1779208847556,15.6249213117366));
#17981=CARTESIAN_POINT('Ctrl Pts',(-205.564222877932,68.1454656278869,15.7838296305408));
#17982=CARTESIAN_POINT('Ctrl Pts',(-207.949795141323,66.2293114813142,15.9427379493452));
#17983=CARTESIAN_POINT('Ctrl Pts',(-207.630968346465,63.1860789341055,16.1016462681495));
#17984=CARTESIAN_POINT('Ctrl Pts',(-204.900222369535,61.805951176065,16.2605545869538));
#17985=CARTESIAN_POINT('Ctrl Pts',(-202.260697801607,63.353840056302,16.4194629057581));
#17986=CARTESIAN_POINT('Ctrl Pts',(-202.133056954791,66.4114280330604,16.5783712245624));
#17987=CARTESIAN_POINT('Ctrl Pts',(-204.632722473373,68.1739683102836,16.7372795433667));
#17988=CARTESIAN_POINT('Ctrl Pts',(-207.471316987812,67.0288605189738,16.896187862171));
#17989=CARTESIAN_POINT('Ctrl Pts',(-208.039624584823,64.0192083031125,17.0550961809753));
#17990=CARTESIAN_POINT('Ctrl Pts',(-206.56709509676,62.6211960514382,17.1610350601782));
#17991=CARTESIAN_POINT('Ctrl Pts',(-205.698066426161,62.3888678140614,17.2140044997796));
#17992=CARTESIAN_POINT('Ctrl Pts',(-207.195197104019,66.8768634390787,-0.214004499779621));
#17993=CARTESIAN_POINT('Ctrl Pts',(-207.819848796546,66.1462649533789,-0.161035060178185));
#17994=CARTESIAN_POINT('Ctrl Pts',(-208.270381695193,64.0238642990776,-0.0550961809753146));
#17995=CARTESIAN_POINT('Ctrl Pts',(-205.948234431212,61.7175191469019,0.103812137828992));
#17996=CARTESIAN_POINT('Ctrl Pts',(-202.755424311813,62.4272763820159,0.262720456633299));
#17997=CARTESIAN_POINT('Ctrl Pts',(-201.621026904811,65.4923916653317,0.421628775437605));
#17998=CARTESIAN_POINT('Ctrl Pts',(-203.584133015616,68.107677391492,0.580537094241912));
#17999=CARTESIAN_POINT('Ctrl Pts',(-206.845436332065,67.8731070036025,0.739445413046219));
#18000=CARTESIAN_POINT('Ctrl Pts',(-208.414793219705,65.004879314059,0.898353731850525));
#18001=CARTESIAN_POINT('Ctrl Pts',(-206.853540350764,62.131996121022,1.05726205065483));
#18002=CARTESIAN_POINT('Ctrl Pts',(-203.592965645672,61.88855533608,1.21617036945914));
#18003=CARTESIAN_POINT('Ctrl Pts',(-201.622352451459,64.4976092498449,1.37507868826345));
#18004=CARTESIAN_POINT('Ctrl Pts',(-202.748324823919,67.5672702726462,1.53398700706775));
#18005=CARTESIAN_POINT('Ctrl Pts',(-205.938609752273,68.2832764585058,1.69289532587206));
#18006=CARTESIAN_POINT('Ctrl Pts',(-208.268386817258,65.9892164116696,1.85180364467637));
#18007=CARTESIAN_POINT('Ctrl Pts',(-207.601743831544,62.7882514210722,2.01071196348067));
#18008=CARTESIAN_POINT('Ctrl Pts',(-204.549850960038,61.6149939701982,2.16962028228498));
#18009=CARTESIAN_POINT('Ctrl Pts',(-201.910649804104,63.545071649082,2.32852860108929));
#18010=CARTESIAN_POINT('Ctrl Pts',(-202.103730326783,66.8090116530371,2.48743691989359));
#18011=CARTESIAN_POINT('Ctrl Pts',(-204.952078540099,68.4144698591525,2.6463452386979));
#18012=CARTESIAN_POINT('Ctrl Pts',(-207.844360599983,66.8895803259649,2.80525355750221));
#18013=CARTESIAN_POINT('Ctrl Pts',(-208.128964658589,63.6323446379311,2.96416187630651));
#18014=CARTESIAN_POINT('Ctrl Pts',(-205.544968887098,61.6289601151182,3.12307019511082));
#18015=CARTESIAN_POINT('Ctrl Pts',(-202.461351732326,62.7161072739279,3.28197851391513));
#18016=CARTESIAN_POINT('Ctrl Pts',(-201.705138934727,65.8971017610087,3.44088683271943));
#18017=CARTESIAN_POINT('Ctrl Pts',(-203.969617936122,68.2556433785665,3.59979515152374));
#18018=CARTESIAN_POINT('Ctrl Pts',(-207.178739697151,67.629447535158,3.75870347032805));
#18019=CARTESIAN_POINT('Ctrl Pts',(-208.390417255234,64.592603579895,3.91761178913235));
#18020=CARTESIAN_POINT('Ctrl Pts',(-206.493798167673,61.9292561093994,4.07652010793666));
#18021=CARTESIAN_POINT('Ctrl Pts',(-203.227681615882,62.0811323166393,4.23542842674096));
#18022=CARTESIAN_POINT('Ctrl Pts',(-201.586406749804,64.908993792451,4.39433674554527));
#18023=CARTESIAN_POINT('Ctrl Pts',(-203.074676022485,67.8202887421631,4.55324506434958));
#18024=CARTESIAN_POINT('Ctrl Pts',(-206.328060798801,68.1459744948553,4.71215338315388));
#18025=CARTESIAN_POINT('Ctrl Pts',(-208.363894278238,65.5874659925654,4.8710617019582));
#18026=CARTESIAN_POINT('Ctrl Pts',(-207.315747080937,62.4903752342799,5.0299700207625));
#18027=CARTESIAN_POINT('Ctrl Pts',(-204.144548842459,61.6940804116484,5.18887833956681));
#18028=CARTESIAN_POINT('Ctrl Pts',(-201.757618664014,63.9286157180384,5.34778665837111));
#18029=CARTESIAN_POINT('Ctrl Pts',(-202.343267454975,67.14538415949,5.50669497717542));
#18030=CARTESIAN_POINT('Ctrl Pts',(-205.364578949465,68.3952883820365,5.66560329597973));
#18031=CARTESIAN_POINT('Ctrl Pts',(-208.051648537909,66.5324301643681,5.82451161478404));
#18032=CARTESIAN_POINT('Ctrl Pts',(-207.941000854442,63.2646570996623,5.98341993358834));
#18033=CARTESIAN_POINT('Ctrl Pts',(-205.134076458582,61.5878270104172,6.14232825239265));
#18034=CARTESIAN_POINT('Ctrl Pts',(-202.204232264038,63.0392389808696,6.30123657119695));
#18035=CARTESIAN_POINT('Ctrl Pts',(-201.837516682106,66.2882547386403,6.46014489000126));
#18036=CARTESIAN_POINT('Ctrl Pts',(-204.370130459597,68.3562129505824,6.61905320880557));
#18037=CARTESIAN_POINT('Ctrl Pts',(-207.480201591807,67.3472326411288,6.77796152760987));
#18038=CARTESIAN_POINT('Ctrl Pts',(-208.316451625349,64.1863356808223,6.93686984641418));
#18039=CARTESIAN_POINT('Ctrl Pts',(-206.112215876065,61.77139707418,7.09577816521849));
#18040=CARTESIAN_POINT('Ctrl Pts',(-202.888313042611,62.3164055445022,7.25468648402279));
#18041=CARTESIAN_POINT('Ctrl Pts',(-201.600381209803,65.3217034176442,7.4135948028271));
#18042=CARTESIAN_POINT('Ctrl Pts',(-203.429181887011,68.0320671931028,7.57250312163141));
#18043=CARTESIAN_POINT('Ctrl Pts',(-206.698091053498,67.9626656547127,7.73141144043571));
#18044=CARTESIAN_POINT('Ctrl Pts',(-208.410209321351,65.1771253571837,7.89031975924002));
#18045=CARTESIAN_POINT('Ctrl Pts',(-206.995885798594,62.229198511882,8.04922807804433));
#18046=CARTESIAN_POINT('Ctrl Pts',(-203.751756483289,61.8215115022116,8.20813639684863));
#18047=CARTESIAN_POINT('Ctrl Pts',(-201.652002872745,64.3278272220048,8.36704471565294));
#18048=CARTESIAN_POINT('Ctrl Pts',(-202.621655608597,67.4503834319279,8.52595303445724));
#18049=CARTESIAN_POINT('Ctrl Pts',(-205.771747900224,68.3264554988884,8.68486135326156));
#18050=CARTESIAN_POINT('Ctrl Pts',(-208.214310342592,66.1528703435735,8.84376967206586));
#18051=CARTESIAN_POINT('Ctrl Pts',(-207.710028988554,62.9223465426638,9.00267799087016));
#18052=CARTESIAN_POINT('Ctrl Pts',(-204.721223347243,61.5965922099369,9.16158630967448));
#18053=CARTESIAN_POINT('Ctrl Pts',(-201.987997025351,63.3910440999545,9.32049462847878));
#18054=CARTESIAN_POINT('Ctrl Pts',(-202.016141366082,66.6605687761665,9.47940294728308));
#18055=CARTESIAN_POINT('Ctrl Pts',(-204.779853952418,68.4077025582228,9.63831126608739));
#18056=CARTESIAN_POINT('Ctrl Pts',(-207.74539397465,67.0306927220875,9.7972195848917));
#18057=CARTESIAN_POINT('Ctrl Pts',(-208.193987485624,63.7919664949749,9.95612790369601));
#18058=CARTESIAN_POINT('Ctrl Pts',(-205.714368968315,61.6607518833287,10.1150362225003));
#18059=CARTESIAN_POINT('Ctrl Pts',(-202.579824965209,62.5909226229609,10.2739445413046));
#18060=CARTESIAN_POINT('Ctrl Pts',(-201.664070384204,65.7297085761028,10.4328528601089));
#18061=CARTESIAN_POINT('Ctrl Pts',(-203.806658789964,68.1995058624756,10.5917611789132));
#18062=CARTESIAN_POINT('Ctrl Pts',(-207.043289079357,67.7360319343462,10.7506694977175));
#18063=CARTESIAN_POINT('Ctrl Pts',(-208.406654778216,64.7641945088715,10.9095778165218));
#18064=CARTESIAN_POINT('Ctrl Pts',(-206.646837451881,62.0085409221143,11.0684861353262));
#18065=CARTESIAN_POINT('Ctrl Pts',(-203.377217956024,61.9954235830429,11.2273944541305));
#18066=CARTESIAN_POINT('Ctrl Pts',(-201.595346900585,64.7368683215086,11.3863027729348));
#18067=CARTESIAN_POINT('Ctrl Pts',(-202.934823753585,67.7195492418465,11.5452110917391));
#18068=CARTESIAN_POINT('Ctrl Pts',(-206.167631107251,68.2089778130996,11.7041194105434));
#18069=CARTESIAN_POINT('Ctrl Pts',(-208.32996731216,65.7564513913839,11.8630277293477));
#18070=CARTESIAN_POINT('Ctrl Pts',(-207.439426703638,62.6104187887493,12.021936048152));
#18071=CARTESIAN_POINT('Ctrl Pts',(-204.312446958186,61.6551275327322,12.1808443669563));
#18072=CARTESIAN_POINT('Ctrl Pts',(-201.815808156835,63.7663779697622,12.3397526857606));
#18073=CARTESIAN_POINT('Ctrl Pts',(-202.238400848236,67.0085992961677,12.4986610045649));
#18074=CARTESIAN_POINT('Ctrl Pts',(-205.192796776167,68.4093592375623,12.6575693233692));
#18075=CARTESIAN_POINT('Ctrl Pts',(-207.970438774524,66.6844567356291,12.8164776421735));
#18076=CARTESIAN_POINT('Ctrl Pts',(-208.024815704448,63.4152631253657,12.9753859609778));
#18077=CARTESIAN_POINT('Ctrl Pts',(-205.306075404128,61.5989385693468,13.1342942797821));
#18078=CARTESIAN_POINT('Ctrl Pts',(-202.306728594544,62.9006691202864,13.2932025985865));
#18079=CARTESIAN_POINT('Ctrl Pts',(-201.776542906729,66.1270427573506,13.4521109173907));
#18080=CARTESIAN_POINT('Ctrl Pts',(-204.201586655377,68.3201561924549,13.6110192361951));
#18081=CARTESIAN_POINT('Ctrl Pts',(-207.35860683207,67.4693875364316,13.7699275549993));
#18082=CARTESIAN_POINT('Ctrl Pts',(-208.353282632143,64.3547119921617,13.9288358738037));
#18083=CARTESIAN_POINT('Ctrl Pts',(-206.273706382977,61.8316292702757,14.087744192608));
#18084=CARTESIAN_POINT('Ctrl Pts',(-203.026410380573,62.2132734437214,14.2466525114123));
#18085=CARTESIAN_POINT('Ctrl Pts',(-201.588479236079,65.1497573308851,14.4055608302166));
#18086=CARTESIAN_POINT('Ctrl Pts',(-203.278192294382,67.9489454664442,14.5644691490209));
#18087=CARTESIAN_POINT('Ctrl Pts',(-206.546439214669,68.0445731614314,14.7233774678252));
#18088=CARTESIAN_POINT('Ctrl Pts',(-208.396928355277,65.3489706154936,14.8822857866295));
#18089=CARTESIAN_POINT('Ctrl Pts',(-207.133150706409,62.3334348760842,15.0411941054338));
#18090=CARTESIAN_POINT('Ctrl Pts',(-203.913726061192,61.7625779546212,15.2001024242381));
#18091=CARTESIAN_POINT('Ctrl Pts',(-201.690181661616,64.1597498477878,15.3590107430424));
#18092=CARTESIAN_POINT('Ctrl Pts',(-202.501049051044,67.3272609614558,15.5179190618467));
#18093=CARTESIAN_POINT('Ctrl Pts',(-205.602911651457,68.361150266119,15.6768273806511));
#18094=CARTESIAN_POINT('Ctrl Pts',(-208.152062650551,66.3136053930871,15.8357356994553));
#18095=CARTESIAN_POINT('Ctrl Pts',(-207.811373896275,63.0616983319427,15.9946440182597));
#18096=CARTESIAN_POINT('Ctrl Pts',(-204.893380615506,61.5869351871512,16.153552337064));
#18097=CARTESIAN_POINT('Ctrl Pts',(-202.0728637975,63.240962837495,16.3124606558683));
#18098=CARTESIAN_POINT('Ctrl Pts',(-201.936470615377,66.5082096802679,16.4713689746726));
#18099=CARTESIAN_POINT('Ctrl Pts',(-204.607538246351,68.3916073779926,16.6302772934769));
#18100=CARTESIAN_POINT('Ctrl Pts',(-207.640775240907,67.167979523543,16.7891856122812));
#18101=CARTESIAN_POINT('Ctrl Pts',(-208.248051700709,63.9519553977084,16.9480939310855));
#18102=CARTESIAN_POINT('Ctrl Pts',(-206.674550837501,62.4580814192127,17.0540328102884));
#18103=CARTESIAN_POINT('Ctrl Pts',(-205.745932854347,62.2098224301579,17.1070022498898));
#18104=CARTESIAN_POINT('Ctrl Pts',(-207.336062657696,66.9973015569306,-0.321006749669432));
#18105=CARTESIAN_POINT('Ctrl Pts',(-208.000798179763,66.2198206477731,-0.268037310067996));
#18106=CARTESIAN_POINT('Ctrl Pts',(-208.480241724338,63.9612257798655,-0.162098430865125));
#18107=CARTESIAN_POINT('Ctrl Pts',(-206.009082529054,61.5068827161415,-0.00319011206081843));
#18108=CARTESIAN_POINT('Ctrl Pts',(-202.61139013989,62.2621849939844,0.155718206743488));
#18109=CARTESIAN_POINT('Ctrl Pts',(-201.404198577622,65.5239883836563,0.314626525547794));
#18110=CARTESIAN_POINT('Ctrl Pts',(-203.493276988919,68.3070967035895,0.473534844352101));
#18111=CARTESIAN_POINT('Ctrl Pts',(-206.96385777596,68.0574739600344,0.632443163156408));
#18112=CARTESIAN_POINT('Ctrl Pts',(-208.633920120295,65.0051924190987,0.791351481960715));
#18113=CARTESIAN_POINT('Ctrl Pts',(-206.972481828636,61.9479566315291,0.95025980076502));
#18114=CARTESIAN_POINT('Ctrl Pts',(-203.502676407862,61.6888942785303,1.10916811956933));
#18115=CARTESIAN_POINT('Ctrl Pts',(-201.405609184451,64.4653708913607,1.26807643837363));
#18116=CARTESIAN_POINT('Ctrl Pts',(-202.603835078648,67.7320117201147,1.42698475717794));
#18117=CARTESIAN_POINT('Ctrl Pts',(-205.998840235539,68.4939639431765,1.58589307598225));
#18118=CARTESIAN_POINT('Ctrl Pts',(-208.478118835308,66.0526943186335,1.74480139478656));
#18119=CARTESIAN_POINT('Ctrl Pts',(-207.768697443447,62.6463237610936,1.90370971359086));
#18120=CARTESIAN_POINT('Ctrl Pts',(-204.520964946279,61.3977785102674,2.06261803239517));
#18121=CARTESIAN_POINT('Ctrl Pts',(-201.712406546107,63.4517090588448,2.22152635119947));
#18122=CARTESIAN_POINT('Ctrl Pts',(-201.917877024422,66.9250957293356,2.38043467000378));
#18123=CARTESIAN_POINT('Ctrl Pts',(-204.949003425354,68.6335760097311,2.53934298880809));
#18124=CARTESIAN_POINT('Ctrl Pts',(-208.026882902896,67.010834485032,2.6982513076124));
#18125=CARTESIAN_POINT('Ctrl Pts',(-208.329749972245,63.5445823456684,2.8571596264167));
#18126=CARTESIAN_POINT('Ctrl Pts',(-205.579939479888,61.4126408611514,3.01606794522101));
#18127=CARTESIAN_POINT('Ctrl Pts',(-202.298446955729,62.5695501320622,3.17497626402532));
#18128=CARTESIAN_POINT('Ctrl Pts',(-201.493708067131,65.9546686810988,3.33388458282962));
#18129=CARTESIAN_POINT('Ctrl Pts',(-203.90349843384,68.4645576515751,3.49279290163393));
#18130=CARTESIAN_POINT('Ctrl Pts',(-207.318549180862,67.7981788906371,3.65170122043823));
#18131=CARTESIAN_POINT('Ctrl Pts',(-208.607979952898,64.5664609969902,3.81060953924254));
#18132=CARTESIAN_POINT('Ctrl Pts',(-206.589655029722,61.7322068159406,3.96951785804685));
#18133=CARTESIAN_POINT('Ctrl Pts',(-203.113952142563,61.893828902484,4.12842617685116));
#18134=CARTESIAN_POINT('Ctrl Pts',(-201.367356851125,64.9031539342483,4.28733449565546));
#18135=CARTESIAN_POINT('Ctrl Pts',(-202.951128197279,68.0012663566409,4.44624281445977));
#18136=CARTESIAN_POINT('Ctrl Pts',(-206.413282312349,68.3478513278105,4.60515113326408));
#18137=CARTESIAN_POINT('Ctrl Pts',(-208.579754999423,65.6251636198798,4.76405945206838));
#18138=CARTESIAN_POINT('Ctrl Pts',(-207.464348313206,62.3293328925706,4.92296777087269));
#18139=CARTESIAN_POINT('Ctrl Pts',(-204.089654636955,61.4819399198572,5.081876089677));
#18140=CARTESIAN_POINT('Ctrl Pts',(-201.549555414801,63.8598651079893,5.2407844084813));
#18141=CARTESIAN_POINT('Ctrl Pts',(-202.172785223452,67.2830532220644,5.39969272728561));
#18142=CARTESIAN_POINT('Ctrl Pts',(-205.387973940047,68.613163659365,5.55860104608992));
#18143=CARTESIAN_POINT('Ctrl Pts',(-208.247472484712,66.6307660373427,5.71750936489423));
#18144=CARTESIAN_POINT('Ctrl Pts',(-208.129724551721,63.1533003390197,5.87641768369853));
#18145=CARTESIAN_POINT('Ctrl Pts',(-205.142680129997,61.368868249703,6.03532600250284));
#18146=CARTESIAN_POINT('Ctrl Pts',(-202.024828159798,62.9134171646498,6.19423432130715));
#18147=CARTESIAN_POINT('Ctrl Pts',(-201.634580479816,66.3709219017407,6.35314264011145));
#18148=CARTESIAN_POINT('Ctrl Pts',(-204.32971180134,68.5715807618264,6.51205095891576));
#18149=CARTESIAN_POINT('Ctrl Pts',(-207.639355851724,67.4978542982895,6.67095927772006));
#18150=CARTESIAN_POINT('Ctrl Pts',(-208.529267956781,64.1341229320817,6.82986759652437));
#18151=CARTESIAN_POINT('Ctrl Pts',(-206.18358664496,61.5642179840126,6.98877591532868));
#18152=CARTESIAN_POINT('Ctrl Pts',(-202.752806325743,62.1441995871754,7.14768423413298));
#18153=CARTESIAN_POINT('Ctrl Pts',(-201.382228050665,65.3423470901251,7.30659255293729));
#18154=CARTESIAN_POINT('Ctrl Pts',(-203.328382663649,68.2266346071907,7.4655008717416));
#18155=CARTESIAN_POINT('Ctrl Pts',(-206.807057367278,68.1527795798118,7.62440919054589));
#18156=CARTESIAN_POINT('Ctrl Pts',(-208.629042073693,65.1884914716269,7.78331750935022));
#18157=CARTESIAN_POINT('Ctrl Pts',(-207.123961567999,62.0513964889848,7.94222582815451));
#18158=CARTESIAN_POINT('Ctrl Pts',(-203.671656835844,61.6175482493094,8.10113414695882));
#18159=CARTESIAN_POINT('Ctrl Pts',(-201.437162269969,64.2846939697036,8.26004246576313));
#18160=CARTESIAN_POINT('Ctrl Pts',(-202.469037513887,67.6076242638456,8.41895078456743));
#18161=CARTESIAN_POINT('Ctrl Pts',(-205.821270877028,68.5399137777715,8.57785910337175));
#18162=CARTESIAN_POINT('Ctrl Pts',(-208.420572279286,66.2268499051207,8.73676742217605));
#18163=CARTESIAN_POINT('Ctrl Pts',(-207.883931246923,62.7890237517031,8.89567574098036));
#18164=CARTESIAN_POINT('Ctrl Pts',(-204.703334280485,61.3781959110996,9.05458405978466));
#18165=CARTESIAN_POINT('Ctrl Pts',(-201.794717129927,63.2877975790446,9.21349237858897));
#18166=CARTESIAN_POINT('Ctrl Pts',(-201.824667489868,66.7671272895889,9.37240069739327));
#18167=CARTESIAN_POINT('Ctrl Pts',(-204.765727205063,68.6263744518545,9.53130901619758));
#18168=CARTESIAN_POINT('Ctrl Pts',(-207.921565600238,67.1610020478975,9.69021733500189));
#18169=CARTESIAN_POINT('Ctrl Pts',(-208.398945306849,63.714447119501,9.84912565380619));
#18170=CARTESIAN_POINT('Ctrl Pts',(-205.76020994545,61.4464727035873,10.0080339726105));
#18171=CARTESIAN_POINT('Ctrl Pts',(-202.424522602772,62.4363323959849,10.1669422914148));
#18172=CARTESIAN_POINT('Ctrl Pts',(-201.450004152294,65.7765338941607,10.3258506102191));
#18173=CARTESIAN_POINT('Ctrl Pts',(-203.730082217424,68.4048177973288,10.4847589290234));
#18174=CARTESIAN_POINT('Ctrl Pts',(-207.174406712011,67.9116027988503,10.6436672478277));
#18175=CARTESIAN_POINT('Ctrl Pts',(-208.625259435921,64.7490628967685,10.802575566632));
#18176=CARTESIAN_POINT('Ctrl Pts',(-206.752514827754,61.816579326257,10.9614838854363));
#18177=CARTESIAN_POINT('Ctrl Pts',(-203.273084212998,61.8026202489985,11.1203922042406));
#18178=CARTESIAN_POINT('Ctrl Pts',(-201.376870690385,64.7199831910058,11.279300523045));
#18179=CARTESIAN_POINT('Ctrl Pts',(-202.80230162386,67.8940624138088,11.4382088418493));
#18180=CARTESIAN_POINT('Ctrl Pts',(-206.24255786536,68.4148975619695,11.5971171606536));
#18181=CARTESIAN_POINT('Ctrl Pts',(-208.54365094371,65.80499279292,11.7560254794579));
#18182=CARTESIAN_POINT('Ctrl Pts',(-207.595964443522,62.4570796285605,11.9149337982622));
#18183=CARTESIAN_POINT('Ctrl Pts',(-204.268326756069,61.4404874390394,12.0738421170665));
#18184=CARTESIAN_POINT('Ctrl Pts',(-201.611478920896,63.6872165814752,12.2327504358708));
#18185=CARTESIAN_POINT('Ctrl Pts',(-202.061189338237,67.1374908892971,12.3916587546751));
#18186=CARTESIAN_POINT('Ctrl Pts',(-205.205168523821,68.6281374401227,12.5505670734794));
#18187=CARTESIAN_POINT('Ctrl Pts',(-208.161051499856,66.7925481367497,12.7094753922837));
#18188=CARTESIAN_POINT('Ctrl Pts',(-208.218917791317,63.3135707366188,12.868383711088));
#18189=CARTESIAN_POINT('Ctrl Pts',(-205.325716228722,61.3806928361316,13.0272920298923));
#18190=CARTESIAN_POINT('Ctrl Pts',(-202.133901668416,62.7659552915461,13.1862003486966));
#18191=CARTESIAN_POINT('Ctrl Pts',(-201.569694024063,66.1993649655665,13.3451086675009));
#18192=CARTESIAN_POINT('Ctrl Pts',(-204.150352559975,68.5332102455456,13.5040169863053));
#18193=CARTESIAN_POINT('Ctrl Pts',(-207.509958369796,67.627847859619,13.6629253051095));
#18194=CARTESIAN_POINT('Ctrl Pts',(-208.568462405179,64.313303932567,13.8218336239139));
#18195=CARTESIAN_POINT('Ctrl Pts',(-206.355439979715,61.6283152734234,13.9807419427182));
#18196=CARTESIAN_POINT('Ctrl Pts',(-202.899765354501,62.0344495109738,14.1396502615225));
#18197=CARTESIAN_POINT('Ctrl Pts',(-201.369562328613,65.1593672421288,14.2985585803268));
#18198=CARTESIAN_POINT('Ctrl Pts',(-203.167704085678,68.1381789685902,14.4574668991311));
#18199=CARTESIAN_POINT('Ctrl Pts',(-206.645674046841,68.2399430821141,14.6163752179354));
#18200=CARTESIAN_POINT('Ctrl Pts',(-208.614908869506,65.3713640210235,14.7752835367397));
#18201=CARTESIAN_POINT('Ctrl Pts',(-207.270034749662,62.1623216890685,14.934191855544));
#18202=CARTESIAN_POINT('Ctrl Pts',(-203.844019983521,61.5548329425339,15.0931001743483));
#18203=CARTESIAN_POINT('Ctrl Pts',(-201.47779098747,64.1058310891023,15.2520084931526));
#18204=CARTESIAN_POINT('Ctrl Pts',(-202.340691646968,67.4766010381562,15.4109168119569));
#18205=CARTESIAN_POINT('Ctrl Pts',(-205.641600424982,68.5768349043511,15.5698251307612));
#18206=CARTESIAN_POINT('Ctrl Pts',(-208.354330159779,66.3978993048601,15.7287334495655));
#18207=CARTESIAN_POINT('Ctrl Pts',(-207.991779446085,62.9373177297799,15.8876417683699));
#18208=CARTESIAN_POINT('Ctrl Pts',(-204.886538861478,61.3679191982373,16.0465500871742));
#18209=CARTESIAN_POINT('Ctrl Pts',(-201.885029793392,63.1280856186881,16.2054584059785));
#18210=CARTESIAN_POINT('Ctrl Pts',(-201.739884275964,66.6049913274753,16.3643667247828));
#18211=CARTESIAN_POINT('Ctrl Pts',(-204.58235401933,68.6092464457014,16.5232750435871));
#18212=CARTESIAN_POINT('Ctrl Pts',(-207.810233494003,67.3070985281123,16.6821833623914));
#18213=CARTESIAN_POINT('Ctrl Pts',(-208.456478816595,63.8847024923042,16.8410916811957));
#18214=CARTESIAN_POINT('Ctrl Pts',(-206.782006578242,62.2949667869872,16.9470305603986));
#18215=CARTESIAN_POINT('Ctrl Pts',(-205.793799282533,62.0307770462544,17.));
#18216=CARTESIAN_POINT('Ctrl Pts',(-206.913465996665,66.6359872033749,0.));
#18217=CARTESIAN_POINT('Ctrl Pts',(-206.975064353962,66.5780998731382,1.31385826762081E-17));
#18218=CARTESIAN_POINT('Ctrl Pts',(-207.033290473413,66.517061027268,-9.08596571292744E-17));
#18219=CARTESIAN_POINT('Ctrl Pts',(-207.088148064904,66.4532556948983,-9.36750677027476E-17));
#18220=CARTESIAN_POINT('Ctrl Pts',(-207.144459507376,66.3877593760565,-9.65650930617943E-17));
#18221=CARTESIAN_POINT('Ctrl Pts',(-207.197221943433,66.3193475595673,1.65439813454464E-17));
#18222=CARTESIAN_POINT('Ctrl Pts',(-207.246413817218,66.2483881525801,-6.24500451351651E-17));
#18223=CARTESIAN_POINT('Ctrl Pts',(-207.297364147824,66.1748921670169,-1.44267862903041E-16));
#18224=CARTESIAN_POINT('Ctrl Pts',(-207.344484671467,66.0986626833147,-2.11570137502538E-16));
#18225=CARTESIAN_POINT('Ctrl Pts',(-207.387716349603,66.0200643070203,-1.45716771982052E-16));
#18226=CARTESIAN_POINT('Ctrl Pts',(-207.406630208787,65.9856775173915,-1.16905924566839E-16));
#18227=CARTESIAN_POINT('Ctrl Pts',(-207.424799222197,65.950836798184,4.63322983862409E-16));
#18228=CARTESIAN_POINT('Ctrl Pts',(-207.442215989061,65.9155705830685,5.06539254985228E-16));
#18229=CARTESIAN_POINT('Ctrl Pts',(-207.451672386856,65.8964228640095,5.30003440623795E-16));
#18230=CARTESIAN_POINT('Ctrl Pts',(-207.460907000843,65.8771496923497,-3.05997193293947E-17));
#18231=CARTESIAN_POINT('Ctrl Pts',(-207.46991844596,65.8577554924582,-2.77555756156289E-17));
#18232=CARTESIAN_POINT('Ctrl Pts',(-207.478568341098,65.839139411115,-2.50255423570532E-17));
#18233=CARTESIAN_POINT('Ctrl Pts',(-207.487015107733,65.8204058124637,-3.76747677011534E-16));
#18234=CARTESIAN_POINT('Ctrl Pts',(-207.495243417805,65.8015914143888,-3.60822483003176E-16));
#18235=CARTESIAN_POINT('Ctrl Pts',(-207.53178628096,65.7180345274726,-2.90096880750225E-16));
#18236=CARTESIAN_POINT('Ctrl Pts',(-207.564069677878,65.6327939693891,9.41786769087706E-16));
#18237=CARTESIAN_POINT('Ctrl Pts',(-207.592069998968,65.5462689644831,8.32667268468867E-16));
#18238=CARTESIAN_POINT('Ctrl Pts',(-207.620534587111,65.4583093078501,7.21738481850149E-16));
#18239=CARTESIAN_POINT('Ctrl Pts',(-207.644573379561,65.3690215011792,1.52679044846908E-16));
#18240=CARTESIAN_POINT('Ctrl Pts',(-207.664122455327,65.278787817363,1.80411241501588E-16));
#18241=CARTESIAN_POINT('Ctrl Pts',(-207.683373891228,65.1899279653208,2.07721208105181E-16));
#18242=CARTESIAN_POINT('Ctrl Pts',(-207.698271558591,65.1001499107623,4.03184391054926E-16));
#18243=CARTESIAN_POINT('Ctrl Pts',(-207.7087114019,65.0097957225238,4.16333634234434E-16));
#18244=CARTESIAN_POINT('Ctrl Pts',(-207.712805706108,64.9743605610785,4.21490512559996E-16));
#18245=CARTESIAN_POINT('Ctrl Pts',(-207.716213877993,64.9388366075109,3.54060526755959E-16));
#18246=CARTESIAN_POINT('Ctrl Pts',(-207.718927650427,64.9032439712385,4.02455846426619E-16));
#18247=CARTESIAN_POINT('Ctrl Pts',(-207.720523480385,64.8823137729101,4.30914644227349E-16));
#18248=CARTESIAN_POINT('Ctrl Pts',(-207.721879164357,64.8613598200859,1.01489021387037E-17));
#18249=CARTESIAN_POINT('Ctrl Pts',(-207.722992828189,64.8403861801911,-1.38777878078145E-17));
#18250=CARTESIAN_POINT('Ctrl Pts',(-207.723754506584,64.826041484871,-3.03105838585251E-17));
#18251=CARTESIAN_POINT('Ctrl Pts',(-207.724402910459,64.8116871985238,1.32396209708937E-16));
#18252=CARTESIAN_POINT('Ctrl Pts',(-207.724937054538,64.7973399810991,1.38777878078145E-16));
#18253=CARTESIAN_POINT('Ctrl Pts',(-207.728480924081,64.7021509323424,1.81118139856045E-16));
#18254=CARTESIAN_POINT('Ctrl Pts',(-207.727008512663,64.6071119050743,-3.51651214267614E-17));
#18255=CARTESIAN_POINT('Ctrl Pts',(-207.720461908733,64.5126221906688,-2.77555756156289E-17));
#18256=CARTESIAN_POINT('Ctrl Pts',(-207.713937327651,64.4184503406908,-2.03709555972342E-17));
#18257=CARTESIAN_POINT('Ctrl Pts',(-207.702372994406,64.3248231595109,-6.60606084003931E-17));
#18258=CARTESIAN_POINT('Ctrl Pts',(-207.685663588442,64.2321180011441,-5.55111512312578E-17));
#18259=CARTESIAN_POINT('Ctrl Pts',(-207.683580824393,64.2205626549263,-5.41962014253678E-17));
#18260=CARTESIAN_POINT('Ctrl Pts',(-207.68141805756,64.2090216217805,-4.52545427453158E-17));
#18261=CARTESIAN_POINT('Ctrl Pts',(-207.679175027131,64.1974956243958,-5.55111512312578E-17));
#18262=CARTESIAN_POINT('Ctrl Pts',(-207.661554797347,64.1069526162377,-1.64870956444071E-16));
#18263=CARTESIAN_POINT('Ctrl Pts',(-207.638985905053,64.0173371417335,4.55048391484254E-16));
#18264=CARTESIAN_POINT('Ctrl Pts',(-207.611743404672,63.9288865787528,5.27355936696949E-16));
#18265=CARTESIAN_POINT('Ctrl Pts',(-207.600816806121,63.8934102539034,5.56357515393362E-16));
#18266=CARTESIAN_POINT('Ctrl Pts',(-207.589137769353,63.858121381592,2.22458913192123E-16));
#18267=CARTESIAN_POINT('Ctrl Pts',(-207.576721747478,63.823035642348,2.22044604925031E-16));
#18268=CARTESIAN_POINT('Ctrl Pts',(-207.570942626356,63.806704748379,2.21851762347786E-16));
#18269=CARTESIAN_POINT('Ctrl Pts',(-207.565003819633,63.7904178674733,1.86961011374093E-16));
#18270=CARTESIAN_POINT('Ctrl Pts',(-207.55890679455,63.7741766065144,1.94289029309402E-16));
#18271=CARTESIAN_POINT('Ctrl Pts',(-207.553840826645,63.7606818766017,2.00377819033484E-16));
#18272=CARTESIAN_POINT('Ctrl Pts',(-207.548668946019,63.7472275150126,-2.33100565213495E-16));
#18273=CARTESIAN_POINT('Ctrl Pts',(-207.543393212818,63.7338163202487,-2.22044604925031E-16));
#18274=CARTESIAN_POINT('Ctrl Pts',(-207.509159730858,63.6467929859398,-1.50304051959292E-16));
#18275=CARTESIAN_POINT('Ctrl Pts',(-207.4705477531,63.5615605760055,2.94289231251776E-17));
#18276=CARTESIAN_POINT('Ctrl Pts',(-207.42788979993,63.4783502782173,-2.77555756156289E-17));
#18277=CARTESIAN_POINT('Ctrl Pts',(-207.383652831604,63.3920598907493,-8.70568001595249E-17));
#18278=CARTESIAN_POINT('Ctrl Pts',(-207.335064684792,63.3079433607353,2.06427004750576E-16));
#18279=CARTESIAN_POINT('Ctrl Pts',(-207.282440228002,63.2262620943519,1.66533453693773E-16));
#18280=CARTESIAN_POINT('Ctrl Pts',(-207.229239513817,63.143686387689,1.2620305339923E-16));
#18281=CARTESIAN_POINT('Ctrl Pts',(-207.171913188856,63.0635987542449,7.73907681327724E-17));
#18282=CARTESIAN_POINT('Ctrl Pts',(-207.110734970838,62.9862846789063,0.));
#18283=CARTESIAN_POINT('Ctrl Pts',(-207.08664473883,62.9558406079157,-3.04742704188559E-17));
#18284=CARTESIAN_POINT('Ctrl Pts',(-207.061956723682,62.9258268275662,6.15201622997646E-17));
#18285=CARTESIAN_POINT('Ctrl Pts',(-207.036685701927,62.8962618494865,5.55111512312578E-17));
#18286=CARTESIAN_POINT('Ctrl Pts',(-207.022377248651,62.8795221580103,5.21088489839094E-17));
#18287=CARTESIAN_POINT('Ctrl Pts',(-207.007881874863,62.8629263573898,1.92101835007536E-16));
#18288=CARTESIAN_POINT('Ctrl Pts',(-206.993202121486,62.8464779169567,1.94289029309402E-16));
#18289=CARTESIAN_POINT('Ctrl Pts',(-206.979146903046,62.8307292584226,1.96383171690125E-16));
#18290=CARTESIAN_POINT('Ctrl Pts',(-206.96491979389,62.8151127633992,1.78167578031119E-16));
#18291=CARTESIAN_POINT('Ctrl Pts',(-206.950542135111,62.7996517246072,1.66533453693773E-16));
#18292=CARTESIAN_POINT('Ctrl Pts',(-206.881823170714,62.7257546742894,1.10927392346557E-16));
#18293=CARTESIAN_POINT('Ctrl Pts',(-206.809592952989,62.6553193670047,2.26493089832809E-16));
#18294=CARTESIAN_POINT('Ctrl Pts',(-206.734165057036,62.5886325600171,2.22044604925031E-16));
#18295=CARTESIAN_POINT('Ctrl Pts',(-206.669049633309,62.5310631470145,2.18204315121696E-16));
#18296=CARTESIAN_POINT('Ctrl Pts',(-206.601550089891,62.476287232394,-5.66442745991914E-17));
#18297=CARTESIAN_POINT('Ctrl Pts',(-206.53184161149,62.4245048556646,0.));
#18298=CARTESIAN_POINT('Ctrl Pts',(-206.504681474983,62.4043291689635,2.20700016087845E-17));
#18299=CARTESIAN_POINT('Ctrl Pts',(-206.477185765765,62.3846081125284,1.56807690272953E-16));
#18300=CARTESIAN_POINT('Ctrl Pts',(-206.449363978737,62.3653543217963,1.66533453693773E-16));
#18301=CARTESIAN_POINT('Ctrl Pts',(-206.434093585115,62.3547865979153,1.71871580808257E-16));
#18302=CARTESIAN_POINT('Ctrl Pts',(-206.418726217455,62.3443606145378,-1.45925441287982E-16));
#18303=CARTESIAN_POINT('Ctrl Pts',(-206.403273624565,62.3340849578763,-1.11022302462516E-16));
#18304=CARTESIAN_POINT('Ctrl Pts',(-206.316688826831,62.2765078470346,8.4548838057753E-17));
#18305=CARTESIAN_POINT('Ctrl Pts',(-206.22734730699,62.2235888009188,7.07438163739693E-17));
#18306=CARTESIAN_POINT('Ctrl Pts',(-206.135559047579,62.1756508392814,-1.11022302462516E-16));
#18307=CARTESIAN_POINT('Ctrl Pts',(-206.043770788168,62.127712877644,-2.92788421299001E-16));
#18308=CARTESIAN_POINT('Ctrl Pts',(-205.949535136959,62.0847550816221,-2.90501423862547E-16));
#18309=CARTESIAN_POINT('Ctrl Pts',(-205.853123850132,62.0471417176263,-3.33066907387547E-16));
#18310=CARTESIAN_POINT('Ctrl Pts',(-205.834023263537,62.0396899208525,-3.41271880709564E-16));
#18311=CARTESIAN_POINT('Ctrl Pts',(-205.814837181401,62.0324480470172,-1.75194258867014E-16));
#18312=CARTESIAN_POINT('Ctrl Pts',(-205.795568724168,62.0254151527766,-1.66533453693773E-16));
#18313=CARTESIAN_POINT('Ctrl Pts',(-202.480291681284,64.9980775076607,1.61258330249194));
#18314=CARTESIAN_POINT('Ctrl Pts',(-202.479246282523,64.8744702547577,1.60474993100897));
#18315=CARTESIAN_POINT('Ctrl Pts',(-202.487554291616,64.7510041347843,1.596916559526));
#18316=CARTESIAN_POINT('Ctrl Pts',(-202.505700729609,64.6290014493569,1.58908318804303));
#18317=CARTESIAN_POINT('Ctrl Pts',(-202.628407364081,63.804016461602,1.53611374844159));
#18318=CARTESIAN_POINT('Ctrl Pts',(-203.200975742687,63.0459469563907,1.48314430884016));
#18319=CARTESIAN_POINT('Ctrl Pts',(-203.960945477611,62.7022784785898,1.43017486923872));
#18320=CARTESIAN_POINT('Ctrl Pts',(-204.720915212535,62.3586100007889,1.37720542963728));
#18321=CARTESIAN_POINT('Ctrl Pts',(-205.668286303777,62.4293425503984,1.32423599003585));
#18322=CARTESIAN_POINT('Ctrl Pts',(-206.368785519983,62.8820718258651,1.27126655043441));
#18323=CARTESIAN_POINT('Ctrl Pts',(-207.069284736189,63.3348011013318,1.21829711083298));
#18324=CARTESIAN_POINT('Ctrl Pts',(-207.522912077358,64.1695271026556,1.16532767123154));
#18325=CARTESIAN_POINT('Ctrl Pts',(-207.521734752234,65.0035767677775,1.11235823163011));
#18326=CARTESIAN_POINT('Ctrl Pts',(-207.52055742711,65.8376264328994,1.05938879202867));
#18327=CARTESIAN_POINT('Ctrl Pts',(-207.064575435692,66.6709997618192,1.00641935242723));
#18328=CARTESIAN_POINT('Ctrl Pts',(-206.362793044106,67.1217640390388,0.953449912825799));
#18329=CARTESIAN_POINT('Ctrl Pts',(-205.66101065252,67.5725283162583,0.900480473224363));
#18330=CARTESIAN_POINT('Ctrl Pts',(-204.713427860765,67.6406835417775,0.847511033622928));
#18331=CARTESIAN_POINT('Ctrl Pts',(-203.954442879917,67.2948210647681,0.794541594021492));
#18332=CARTESIAN_POINT('Ctrl Pts',(-203.195457899069,66.9489585877586,0.741572154420057));
#18333=CARTESIAN_POINT('Ctrl Pts',(-202.625070729129,66.1890784082204,0.688602714818621));
#18334=CARTESIAN_POINT('Ctrl Pts',(-202.504678660237,65.3638484733508,0.635633275217186));
#18335=CARTESIAN_POINT('Ctrl Pts',(-202.487215547386,65.2441472038771,0.627949950975436));
#18336=CARTESIAN_POINT('Ctrl Pts',(-202.47922037136,65.1230709697569,0.620266626733685));
#18337=CARTESIAN_POINT('Ctrl Pts',(-202.480232429385,65.0018635099461,0.612583302491936));
#18338=CARTESIAN_POINT('Ctrl Pts',(-204.206200717467,62.0307770462543,-5.55111512312578E-16));
#18339=CARTESIAN_POINT('Ctrl Pts',(-203.217993421758,62.2949667869871,0.052969439601435));
#18340=CARTESIAN_POINT('Ctrl Pts',(-201.543521124928,63.884702084602,0.158908318804306));
#18341=CARTESIAN_POINT('Ctrl Pts',(-202.189766556512,67.3070986306701,0.317816637608613));
#18342=CARTESIAN_POINT('Ctrl Pts',(-205.417645976078,68.6092463233164,0.47672495641292));
#18343=CARTESIAN_POINT('Ctrl Pts',(-208.260115679803,66.6049913509854,0.635633275217227));
#18344=CARTESIAN_POINT('Ctrl Pts',(-208.114970174343,63.128085617879,0.794541594021532));
#18345=CARTESIAN_POINT('Ctrl Pts',(-205.113461133577,61.3679192540746,0.95344991282584));
#18346=CARTESIAN_POINT('Ctrl Pts',(-202.00822059199,62.9373177478322,1.11235823163015));
#18347=CARTESIAN_POINT('Ctrl Pts',(-201.645669878913,66.3978992916336,1.27126655043445));
#18348=CARTESIAN_POINT('Ctrl Pts',(-204.358399583502,68.5768348597731,1.43017486923876));
#18349=CARTESIAN_POINT('Ctrl Pts',(-207.659308320785,67.4766010095058,1.58908318804307));
#18350=CARTESIAN_POINT('Ctrl Pts',(-208.522208970686,64.1058310992964,1.74799150684737));
#18351=CARTESIAN_POINT('Ctrl Pts',(-206.155980002522,61.5548329839681,1.90689982565168));
#18352=CARTESIAN_POINT('Ctrl Pts',(-202.729965277546,62.162321722855,2.06580814445599));
#18353=CARTESIAN_POINT('Ctrl Pts',(-201.385091173662,65.3713640166521,2.22471646326029));
#18354=CARTESIAN_POINT('Ctrl Pts',(-203.354325972851,68.2399430433535,2.3836247820646));
#18355=CARTESIAN_POINT('Ctrl Pts',(-206.83229589241,68.1381789310981,2.54253310086891));
#18356=CARTESIAN_POINT('Ctrl Pts',(-208.630437627999,65.1593672402151,2.70144141967321));
#18357=CARTESIAN_POINT('Ctrl Pts',(-207.100234620393,62.0344495464248,2.86034973847752));
#18358=CARTESIAN_POINT('Ctrl Pts',(-203.644560036488,61.6283153137219,3.01925805728183));
#18359=CARTESIAN_POINT('Ctrl Pts',(-201.431537637472,64.3133039407759,3.17816637608613));
#18360=CARTESIAN_POINT('Ctrl Pts',(-202.490041660205,67.6278478282085,3.33707469489044));
#18361=CARTESIAN_POINT('Ctrl Pts',(-205.849647429869,68.5332102033146,3.49598301369475));
#18362=CARTESIAN_POINT('Ctrl Pts',(-208.430305934935,66.1993649512308,3.65489133249905));
#18363=CARTESIAN_POINT('Ctrl Pts',(-207.866098297326,62.7659553182491,3.81379965130336));
#18364=CARTESIAN_POINT('Ctrl Pts',(-204.674283775171,61.380692879392,3.97270797010767));
#18365=CARTESIAN_POINT('Ctrl Pts',(-201.781082247158,63.3135707567762,4.13161628891197));
#18366=CARTESIAN_POINT('Ctrl Pts',(-201.838948537927,66.7925481153239,4.29052460771628));
#18367=CARTESIAN_POINT('Ctrl Pts',(-204.794831478631,68.6281373967567,4.44943292652058));
#18368=CARTESIAN_POINT('Ctrl Pts',(-207.938810626636,67.1374908637484,4.60834124532489));
#18369=CARTESIAN_POINT('Ctrl Pts',(-208.388521038603,63.6872165971666,4.7672495641292));
#18370=CARTESIAN_POINT('Ctrl Pts',(-205.731673235186,61.4404874815853,4.92615788293351));
#18371=CARTESIAN_POINT('Ctrl Pts',(-202.404035587507,62.4570796589551,5.08506620173781));
#18372=CARTESIAN_POINT('Ctrl Pts',(-201.456349098646,65.8049927832981,5.24397452054212));
#18373=CARTESIAN_POINT('Ctrl Pts',(-203.757442149492,68.4148975211522,5.40288283934643));
#18374=CARTESIAN_POINT('Ctrl Pts',(-207.197698349872,67.894062379217,5.56179115815073));
#18375=CARTESIAN_POINT('Ctrl Pts',(-208.623129266309,64.7199831943528,5.72069947695504));
#18376=CARTESIAN_POINT('Ctrl Pts',(-206.726915766361,61.8026202872159,5.87960779575935));
#18377=CARTESIAN_POINT('Ctrl Pts',(-203.247485193193,61.8165793643074,6.03851611456365));
#18378=CARTESIAN_POINT('Ctrl Pts',(-201.374740607411,64.7490628997678,6.19742443336797));
#18379=CARTESIAN_POINT('Ctrl Pts',(-202.825593313979,67.9116027640487,6.35633275217227));
#18380=CARTESIAN_POINT('Ctrl Pts',(-206.269917767397,68.4048177566322,6.51524107097658));
#18381=CARTESIAN_POINT('Ctrl Pts',(-208.549995805274,65.7765338848791,6.67414938978088));
#18382=CARTESIAN_POINT('Ctrl Pts',(-207.575477366445,62.4363324266277,6.83305770858519));
#18383=CARTESIAN_POINT('Ctrl Pts',(-204.239790063637,61.4464727460615,6.99196602738949));
#18384=CARTESIAN_POINT('Ctrl Pts',(-201.601054733778,63.7144471348668,7.1508743461938));
#18385=CARTESIAN_POINT('Ctrl Pts',(-202.078434434683,67.1610020220675,7.3097826649981));
#18386=CARTESIAN_POINT('Ctrl Pts',(-205.234272792136,68.6263744085096,7.46869098380242));
#18387=CARTESIAN_POINT('Ctrl Pts',(-208.175332472178,66.7671272684671,7.62759930260672));
#18388=CARTESIAN_POINT('Ctrl Pts',(-208.205282831762,63.2877975995101,7.78650762141103));
#18389=CARTESIAN_POINT('Ctrl Pts',(-205.29666571597,61.3781959543899,7.94541594021533));
#18390=CARTESIAN_POINT('Ctrl Pts',(-202.116068787548,62.7890237781302,8.10432425901964));
#18391=CARTESIAN_POINT('Ctrl Pts',(-201.579427761599,66.2268498904564,8.26323257782394));
#18392=CARTESIAN_POINT('Ctrl Pts',(-204.178729132788,68.5399137354599,8.42214089662826));
#18393=CARTESIAN_POINT('Ctrl Pts',(-207.530962455862,67.6076242326776,8.58104921543256));
#18394=CARTESIAN_POINT('Ctrl Pts',(-208.562837687446,64.2846939782535,8.73995753423686));
#18395=CARTESIAN_POINT('Ctrl Pts',(-206.328343148279,61.6175482897389,8.89886585304117));
#18396=CARTESIAN_POINT('Ctrl Pts',(-202.876038457388,62.0513965242284,9.05777417184548));
#18397=CARTESIAN_POINT('Ctrl Pts',(-201.370957969684,65.1884914693738,9.21668249064979));
#18398=CARTESIAN_POINT('Ctrl Pts',(-203.192942654321,68.1527795421275,9.37559080945409));
#18399=CARTESIAN_POINT('Ctrl Pts',(-206.671617316371,68.2266345686238,9.5344991282584));
#18400=CARTESIAN_POINT('Ctrl Pts',(-208.617771906093,65.3423470860332,9.69340744706271));
#18401=CARTESIAN_POINT('Ctrl Pts',(-207.247193647397,62.1441996213101,9.85231576586701));
#18402=CARTESIAN_POINT('Ctrl Pts',(-203.816413369187,61.5642180250794,10.0112240846713));
#18403=CARTESIAN_POINT('Ctrl Pts',(-201.470732085403,64.1341229424312,10.1701324034756));
#18404=CARTESIAN_POINT('Ctrl Pts',(-202.360644179824,67.4978542684331,10.3290407222799));
#18405=CARTESIAN_POINT('Ctrl Pts',(-205.670288190648,68.5715807191365,10.4879490410843));
#18406=CARTESIAN_POINT('Ctrl Pts',(-208.365419479959,66.3709218853546,10.6468573598885));
#18407=CARTESIAN_POINT('Ctrl Pts',(-207.975171804641,62.9134171895902,10.8057656786929));
#18408=CARTESIAN_POINT('Ctrl Pts',(-204.857319871709,61.3688682931048,10.9646739974972));
#18409=CARTESIAN_POINT('Ctrl Pts',(-201.870275485688,63.1533003610926,11.1235823163015));
#18410=CARTESIAN_POINT('Ctrl Pts',(-201.752527554104,66.6307660178506,11.2824906351058));
#18411=CARTESIAN_POINT('Ctrl Pts',(-204.61202606459,68.6131636161778,11.4413989539101));
#18412=CARTESIAN_POINT('Ctrl Pts',(-207.827214742755,67.2830531947759,11.6003072727144));
#18413=CARTESIAN_POINT('Ctrl Pts',(-208.450444543957,63.859865121617,11.7592155915187));
#18414=CARTESIAN_POINT('Ctrl Pts',(-205.910345352164,61.4819399619076,11.918123910323));
#18415=CARTESIAN_POINT('Ctrl Pts',(-202.535651716249,62.3293329244922,12.0770322291273));
#18416=CARTESIAN_POINT('Ctrl Pts',(-201.420245043365,65.6251636124073,12.2359405479316));
#18417=CARTESIAN_POINT('Ctrl Pts',(-203.586717704544,68.3478512877946,12.3948488667359));
#18418=CARTESIAN_POINT('Ctrl Pts',(-207.048871778231,68.0012663207677,12.5537571855402));
#18419=CARTESIAN_POINT('Ctrl Pts',(-208.632643105455,64.9031539354061,12.7126655043445));
#18420=CARTESIAN_POINT('Ctrl Pts',(-206.886047834894,61.8938289396112,12.8715738231488));
#18421=CARTESIAN_POINT('Ctrl Pts',(-203.410344989279,61.7322068549995,13.0304821419532));
#18422=CARTESIAN_POINT('Ctrl Pts',(-201.392020090227,64.5664610021721,13.1893904607575));
#18423=CARTESIAN_POINT('Ctrl Pts',(-202.681450846851,67.7981788571913,13.3482987795618));
#18424=CARTESIAN_POINT('Ctrl Pts',(-206.096501553054,68.4645576101642,13.5072070983661));
#18425=CARTESIAN_POINT('Ctrl Pts',(-208.506291890959,65.9546686696882,13.6661154171704));
#18426=CARTESIAN_POINT('Ctrl Pts',(-207.70155301198,62.5695501611123,13.8250237359747));
#18427=CARTESIAN_POINT('Ctrl Pts',(-204.420060527044,61.4126409040308,13.983932054779));
#18428=CARTESIAN_POINT('Ctrl Pts',(-201.670250067554,63.5445823630629,14.1428403735833));
#18429=CARTESIAN_POINT('Ctrl Pts',(-201.973117133283,67.0108344609999,14.3017486923876));
#18430=CARTESIAN_POINT('Ctrl Pts',(-205.050996574037,68.6335759662945,14.4606570111919));
#18431=CARTESIAN_POINT('Ctrl Pts',(-208.082122938738,66.9250957063364,14.6195653299962));
#18432=CARTESIAN_POINT('Ctrl Pts',(-208.287593414598,63.4517090773303,14.7784736488005));
#18433=CARTESIAN_POINT('Ctrl Pts',(-205.479035047994,61.3977785533642,14.9373819676048));
#18434=CARTESIAN_POINT('Ctrl Pts',(-202.231302589651,62.6463237891479,15.0962902864091));
#18435=CARTESIAN_POINT('Ctrl Pts',(-201.521881206253,66.0526943062019,15.2551986052135));
#18436=CARTESIAN_POINT('Ctrl Pts',(-204.001159776429,68.4939639011247,15.4141069240177));
#18437=CARTESIAN_POINT('Ctrl Pts',(-207.396164892643,67.7320116880119,15.5730152428221));
#18438=CARTESIAN_POINT('Ctrl Pts',(-208.594390772745,64.4653708967053,15.7319235616264));
#18439=CARTESIAN_POINT('Ctrl Pts',(-206.497323573879,61.6888943200732,15.8908318804307));
#18440=CARTESIAN_POINT('Ctrl Pts',(-203.027518195758,61.9479566643454,16.049740199235));
#18441=CARTESIAN_POINT('Ctrl Pts',(-201.366079921308,65.0051924257885,16.2086485180393));
#18442=CARTESIAN_POINT('Ctrl Pts',(-203.036142251593,68.0574739112173,16.3675568368436));
#18443=CARTESIAN_POINT('Ctrl Pts',(-206.506722984033,68.3070966859805,16.5264651556479));
#18444=CARTESIAN_POINT('Ctrl Pts',(-208.595801399242,65.5239883392264,16.6853734744522));
#18445=CARTESIAN_POINT('Ctrl Pts',(-207.388609787001,62.2621850922406,16.8442817932565));
#18446=CARTESIAN_POINT('Ctrl Pts',(-203.990917570668,61.5068826602371,17.0031901120608));
#18447=CARTESIAN_POINT('Ctrl Pts',(-201.519757996531,63.9612260827295,17.1620984308651));
#18448=CARTESIAN_POINT('Ctrl Pts',(-201.999201820237,66.219820647773,17.268037310068));
#18449=CARTESIAN_POINT('Ctrl Pts',(-202.663937342304,66.9973015569306,17.3210067496694));
#18450=CARTESIAN_POINT('Ctrl Pts',(-204.254067145653,62.2098224301579,-0.107002249889811));
#18451=CARTESIAN_POINT('Ctrl Pts',(-203.325449162499,62.4580814192126,-0.0540328102883756));
#18452=CARTESIAN_POINT('Ctrl Pts',(-201.75194824434,63.9519550145908,0.0519060689144955));
#18453=CARTESIAN_POINT('Ctrl Pts',(-202.359224806561,67.1679796199166,0.210814387718803));
#18454=CARTESIAN_POINT('Ctrl Pts',(-205.392461749333,68.3916072629874,0.369722706523109));
#18455=CARTESIAN_POINT('Ctrl Pts',(-208.063529343057,66.5082097023603,0.528631025327416));
#18456=CARTESIAN_POINT('Ctrl Pts',(-207.927136172181,63.2409628367347,0.687539344131722));
#18457=CARTESIAN_POINT('Ctrl Pts',(-205.106619379847,61.5869352396215,0.846447662936029));
#18458=CARTESIAN_POINT('Ctrl Pts',(-202.188626139504,63.0616983489064,1.00535598174034));
#18459=CARTESIAN_POINT('Ctrl Pts',(-201.847937385808,66.3136053806583,1.16426430054464));
#18460=CARTESIAN_POINT('Ctrl Pts',(-204.397088356516,68.3611502242289,1.32317261934895));
#18461=CARTESIAN_POINT('Ctrl Pts',(-207.498950918653,67.3272609345331,1.48208093815326));
#18462=CARTESIAN_POINT('Ctrl Pts',(-208.309818299063,64.1597498573671,1.64098925695756));
#18463=CARTESIAN_POINT('Ctrl Pts',(-206.086273925693,61.7625779935569,1.79989757576187));
#18464=CARTESIAN_POINT('Ctrl Pts',(-202.866849319158,62.3334349078333,1.95880589456617));
#18465=CARTESIAN_POINT('Ctrl Pts',(-201.603071685287,65.3489706113857,2.11771421337048));
#18466=CARTESIAN_POINT('Ctrl Pts',(-203.453560803836,68.0445731250081,2.27662253217479));
#18467=CARTESIAN_POINT('Ctrl Pts',(-206.721807685027,67.9489454312129,2.4355308509791));
#18468=CARTESIAN_POINT('Ctrl Pts',(-208.41152072315,65.1497573290867,2.5944391697834));
#18469=CARTESIAN_POINT('Ctrl Pts',(-206.973589595835,62.2132734770346,2.75334748858771));
#18470=CARTESIAN_POINT('Ctrl Pts',(-203.726293632249,61.8316293081442,2.91225580739202));
#18471=CARTESIAN_POINT('Ctrl Pts',(-201.646717407937,64.3547119998756,3.07116412619632));
#18472=CARTESIAN_POINT('Ctrl Pts',(-202.641393196122,67.4693875069152,3.23007244500063));
#18473=CARTESIAN_POINT('Ctrl Pts',(-205.79841333508,68.3201561527704,3.38898076380493));
#18474=CARTESIAN_POINT('Ctrl Pts',(-208.223457054742,66.1270427438794,3.54788908260924));
#18475=CARTESIAN_POINT('Ctrl Pts',(-207.693271373264,62.9006691453792,3.70679740141355));
#18476=CARTESIAN_POINT('Ctrl Pts',(-204.69392459953,61.5989386099986,3.86570572021786));
#18477=CARTESIAN_POINT('Ctrl Pts',(-201.975184331707,63.4152631443075,4.02461403902216));
#18478=CARTESIAN_POINT('Ctrl Pts',(-202.02956126098,66.6844567154952,4.18352235782647));
#18479=CARTESIAN_POINT('Ctrl Pts',(-204.807203226137,68.4093591968113,4.34243067663077));
#18480=CARTESIAN_POINT('Ctrl Pts',(-207.761599118756,67.0085992721596,4.50133899543508));
#18481=CARTESIAN_POINT('Ctrl Pts',(-208.184191805105,63.7663779845074,4.66024731423939));
#18482=CARTESIAN_POINT('Ctrl Pts',(-205.687553033595,61.6551275727124,4.8191556330437));
#18483=CARTESIAN_POINT('Ctrl Pts',(-202.56057332552,62.6104188173111,4.97806395184801));
#18484=CARTESIAN_POINT('Ctrl Pts',(-201.670032727642,65.7564513823422,5.13697227065231));
#18485=CARTESIAN_POINT('Ctrl Pts',(-203.832368906705,68.2089777747436,5.29588058945662));
#18486=CARTESIAN_POINT('Ctrl Pts',(-207.06517622173,67.7195492093407,5.45478890826092));
#18487=CARTESIAN_POINT('Ctrl Pts',(-208.404653058721,64.7368683246537,5.61369722706523));
#18488=CARTESIAN_POINT('Ctrl Pts',(-206.622782024579,61.9954236189558,5.77260554586954));
#18489=CARTESIAN_POINT('Ctrl Pts',(-203.353162567803,62.0085409578702,5.93151386467384));
#18490=CARTESIAN_POINT('Ctrl Pts',(-201.593345262503,64.76419451169,6.09042218347815));
#18491=CARTESIAN_POINT('Ctrl Pts',(-202.956710945065,67.7360319016432,6.24933050228246));
#18492=CARTESIAN_POINT('Ctrl Pts',(-206.193341195772,68.1995058242328,6.40823882108676));
#18493=CARTESIAN_POINT('Ctrl Pts',(-208.335929575923,65.729708567381,6.56714713989107));
#18494=CARTESIAN_POINT('Ctrl Pts',(-207.420175005863,62.5909226517559,6.72605545869538));
#18495=CARTESIAN_POINT('Ctrl Pts',(-204.285631040223,61.6607519232417,6.88496377749968));
#18496=CARTESIAN_POINT('Ctrl Pts',(-201.806012552553,63.7919665094142,7.04387209630399));
#18497=CARTESIAN_POINT('Ctrl Pts',(-202.254606058165,67.0306926978151,7.2027804151083));
#18498=CARTESIAN_POINT('Ctrl Pts',(-205.22014604495,68.4077025174916,7.3616887339126));
#18499=CARTESIAN_POINT('Ctrl Pts',(-207.983858598253,66.6605687563183,7.52059705271691));
#18500=CARTESIAN_POINT('Ctrl Pts',(-208.012002938647,63.391044119186,7.67950537152122));
#18501=CARTESIAN_POINT('Ctrl Pts',(-205.278776649425,61.5965922506168,7.83841369032552));
#18502=CARTESIAN_POINT('Ctrl Pts',(-202.289971043838,62.9223465674972,7.99732200912984));
#18503=CARTESIAN_POINT('Ctrl Pts',(-201.785689695828,66.1528703297934,8.15623032793413));
#18504=CARTESIAN_POINT('Ctrl Pts',(-204.228252109001,68.3264554591282,8.31513864673845));
#18505=CARTESIAN_POINT('Ctrl Pts',(-207.378344362975,67.4503834026392,8.47404696554275));
#18506=CARTESIAN_POINT('Ctrl Pts',(-208.347997087237,64.3278272300392,8.63295528434705));
#18507=CARTESIAN_POINT('Ctrl Pts',(-206.248243501792,61.8215115402032,8.79186360315136));
#18508=CARTESIAN_POINT('Ctrl Pts',(-203.004114225263,62.2291985450005,8.95077192195567));
#18509=CARTESIAN_POINT('Ctrl Pts',(-201.589790719411,65.1771253550663,9.10968024075998));
#18510=CARTESIAN_POINT('Ctrl Pts',(-203.301908966799,67.9626656193009,9.26858855956429));
#18511=CARTESIAN_POINT('Ctrl Pts',(-206.570818094213,68.0320671568614,9.42749687836859));
#18512=CARTESIAN_POINT('Ctrl Pts',(-208.399618749562,65.3217034137992,9.58640519717289));
#18513=CARTESIAN_POINT('Ctrl Pts',(-207.111686932148,62.3164055765784,9.7453135159772));
#18514=CARTESIAN_POINT('Ctrl Pts',(-203.887784137229,61.7713971127705,9.90422183478151));
#18515=CARTESIAN_POINT('Ctrl Pts',(-201.683548414291,64.1863356905477,10.0631301535858));
#18516=CARTESIAN_POINT('Ctrl Pts',(-202.519798437837,67.347232613073,10.2220384723901));
#18517=CARTESIAN_POINT('Ctrl Pts',(-205.629869532874,68.3562129104667,10.3809467911944));
#18518=CARTESIAN_POINT('Ctrl Pts',(-208.162483280093,66.2882547232422,10.5398551099987));
#18519=CARTESIAN_POINT('Ctrl Pts',(-207.795767702545,63.0392390043061,10.698763428803));
#18520=CARTESIAN_POINT('Ctrl Pts',(-204.86592354302,61.5878270512018,10.8576717476073));
#18521=CARTESIAN_POINT('Ctrl Pts',(-202.05899918071,63.2646571204042,11.0165800664117));
#18522=CARTESIAN_POINT('Ctrl Pts',(-201.948351498567,66.5324301460514,11.175488385216));
#18523=CARTESIAN_POINT('Ctrl Pts',(-204.635421054893,68.3952883414536,11.3343967040203));
#18524=CARTESIAN_POINT('Ctrl Pts',(-207.65673251327,67.145384133847,11.4933050228246));
#18525=CARTESIAN_POINT('Ctrl Pts',(-208.242381297231,63.9286157308444,11.6522133416289));
#18526=CARTESIAN_POINT('Ctrl Pts',(-205.855451147316,61.694080451163,11.8111216604332));
#18527=CARTESIAN_POINT('Ctrl Pts',(-202.684252946743,62.4903752642767,11.9700299792375));
#18528=CARTESIAN_POINT('Ctrl Pts',(-201.636105761969,65.5874659855433,12.1289382980418));
#18529=CARTESIAN_POINT('Ctrl Pts',(-203.671939217073,68.1459744572525,12.2878466168461));
#18530=CARTESIAN_POINT('Ctrl Pts',(-206.925323954502,67.8202887084531,12.4467549356504));
#18531=CARTESIAN_POINT('Ctrl Pts',(-208.413593209394,64.9089937935389,12.6056632544547));
#18532=CARTESIAN_POINT('Ctrl Pts',(-206.772318362935,62.0811323515277,12.764571573259));
#18533=CARTESIAN_POINT('Ctrl Pts',(-203.506201850182,61.929256146103,12.9234798920633));
#18534=CARTESIAN_POINT('Ctrl Pts',(-201.609582785291,64.5926035847644,13.0823882108676));
#18535=CARTESIAN_POINT('Ctrl Pts',(-202.821260328891,67.6294475037291,13.241296529672));
#18536=CARTESIAN_POINT('Ctrl Pts',(-206.030382051563,68.2556433396526,13.4002048484763));
#18537=CARTESIAN_POINT('Ctrl Pts',(-208.29486102589,65.8971017502862,13.5591131672806));
#18538=CARTESIAN_POINT('Ctrl Pts',(-207.53864823733,62.7161073012263,13.7180214860849));
#18539=CARTESIAN_POINT('Ctrl Pts',(-204.455031119415,61.6289601554119,13.8769298048892));
#18540=CARTESIAN_POINT('Ctrl Pts',(-201.871035378811,63.6323446542768,14.0358381236935));
#18541=CARTESIAN_POINT('Ctrl Pts',(-202.155639434015,66.889580303382,14.1947464424978));
#18542=CARTESIAN_POINT('Ctrl Pts',(-205.047921459329,68.4144698183351,14.3536547613021));
#18543=CARTESIAN_POINT('Ctrl Pts',(-207.896269638598,66.8090116314247,14.5125630801064));
#18544=CARTESIAN_POINT('Ctrl Pts',(-208.089350158971,63.5450716664528,14.6714713989107));
#18545=CARTESIAN_POINT('Ctrl Pts',(-205.45014903458,61.6149940106962,14.830379717715));
#18546=CARTESIAN_POINT('Ctrl Pts',(-202.398256199559,62.7882514474348,14.9892880365193));
#18547=CARTESIAN_POINT('Ctrl Pts',(-201.731613221797,65.9892163999876,15.1481963553236));
#18548=CARTESIAN_POINT('Ctrl Pts',(-204.061390258974,68.2832764189897,15.3071046741279));
#18549=CARTESIAN_POINT('Ctrl Pts',(-207.251675149103,67.5672702424791,15.4660129929322));
#18550=CARTESIAN_POINT('Ctrl Pts',(-208.377647508318,64.4976092548672,15.6249213117366));
#18551=CARTESIAN_POINT('Ctrl Pts',(-206.40703433717,61.8885553751179,15.7838296305409));
#18552=CARTESIAN_POINT('Ctrl Pts',(-203.146459672159,62.1319961518595,15.9427379493452));
#18553=CARTESIAN_POINT('Ctrl Pts',(-201.585206819389,65.0048793203454,16.1016462681495));
#18554=CARTESIAN_POINT('Ctrl Pts',(-203.154563693826,67.8731069577291,16.2605545869538));
#18555=CARTESIAN_POINT('Ctrl Pts',(-206.415866958967,68.1076773749448,16.4194629057581));
#18556=CARTESIAN_POINT('Ctrl Pts',(-208.378973073449,65.4923916235809,16.5783712245624));
#18557=CARTESIAN_POINT('Ctrl Pts',(-207.244575619486,62.4272764743473,16.7372795433667));
#18558=CARTESIAN_POINT('Ctrl Pts',(-204.051765662497,61.7175190943685,16.896187862171));
#18559=CARTESIAN_POINT('Ctrl Pts',(-201.729618042508,64.0238645836787,17.0550961809753));
#18560=CARTESIAN_POINT('Ctrl Pts',(-202.180151203454,66.1462649533788,17.1610350601782));
#18561=CARTESIAN_POINT('Ctrl Pts',(-202.804802895981,66.8768634390786,17.2140044997796));
#18562=CARTESIAN_POINT('Ctrl Pts',(-204.301933573839,62.3888678140614,-0.214004499779622));
#18563=CARTESIAN_POINT('Ctrl Pts',(-203.43290490324,62.6211960514381,-0.161035060178186));
#18564=CARTESIAN_POINT('Ctrl Pts',(-201.960375363752,64.0192079445796,-0.0550961809753149));
#18565=CARTESIAN_POINT('Ctrl Pts',(-202.52868305661,67.0288606091631,0.103812137828991));
#18566=CARTESIAN_POINT('Ctrl Pts',(-205.367277522588,68.1739682026583,0.262720456633299));
#18567=CARTESIAN_POINT('Ctrl Pts',(-207.86694300631,66.4114280537352,0.421628775437604));
#18568=CARTESIAN_POINT('Ctrl Pts',(-207.739302170019,63.3538400555904,0.580537094241912));
#18569=CARTESIAN_POINT('Ctrl Pts',(-205.099777626116,61.8059512251683,0.739445413046217));
#18570=CARTESIAN_POINT('Ctrl Pts',(-202.369031687018,63.1860789499808,0.898353731850525));
#18571=CARTESIAN_POINT('Ctrl Pts',(-202.050204892703,66.229311469683,1.05726205065483));
#18572=CARTESIAN_POINT('Ctrl Pts',(-204.43577712953,68.1454655886849,1.21617036945914));
#18573=CARTESIAN_POINT('Ctrl Pts',(-207.338593516521,67.1779208595605,1.37507868826344));
#18574=CARTESIAN_POINT('Ctrl Pts',(-208.09742762744,64.2136686154378,1.53398700706775));
#18575=CARTESIAN_POINT('Ctrl Pts',(-206.016567848864,61.9703230031457,1.69289532587206));
#18576=CARTESIAN_POINT('Ctrl Pts',(-203.00373336077,62.5045480928116,1.85180364467637));
#18577=CARTESIAN_POINT('Ctrl Pts',(-201.821052196913,65.3265772061194,2.01071196348067));
#18578=CARTESIAN_POINT('Ctrl Pts',(-203.55279563482,67.8492032066626,2.16962028228498));
#18579=CARTESIAN_POINT('Ctrl Pts',(-206.611319477643,67.7597119313279,2.32852860108929));
#18580=CARTESIAN_POINT('Ctrl Pts',(-208.1926038183,65.1401474179583,2.48743691989359));
#18581=CARTESIAN_POINT('Ctrl Pts',(-206.846944571277,62.3920974076444,2.6463452386979));
#18582=CARTESIAN_POINT('Ctrl Pts',(-203.80802722801,62.0349433025665,2.80525355750221));
#18583=CARTESIAN_POINT('Ctrl Pts',(-201.861897178401,64.3961200589753,2.96416187630651));
#18584=CARTESIAN_POINT('Ctrl Pts',(-202.79274473204,67.310927185622,3.12307019511082));
#18585=CARTESIAN_POINT('Ctrl Pts',(-205.74717924029,68.1071021022261,3.28197851391513));
#18586=CARTESIAN_POINT('Ctrl Pts',(-208.016608174548,66.0547205365278,3.44088683271943));
#18587=CARTESIAN_POINT('Ctrl Pts',(-207.520444449202,63.0353829725094,3.59979515152374));
#18588=CARTESIAN_POINT('Ctrl Pts',(-204.713565423889,61.8171843406052,3.75870347032804));
#18589=CARTESIAN_POINT('Ctrl Pts',(-202.169286416255,63.5169555318388,3.91761178913235));
#18590=CARTESIAN_POINT('Ctrl Pts',(-202.220173984034,66.5763653156666,4.07652010793666));
#18591=CARTESIAN_POINT('Ctrl Pts',(-204.819574973643,68.1905809968658,4.23542842674096));
#18592=CARTESIAN_POINT('Ctrl Pts',(-207.584387610876,66.8797076805709,4.39433674554527));
#18593=CARTESIAN_POINT('Ctrl Pts',(-207.979862571607,63.8455393718481,4.55324506434958));
#18594=CARTESIAN_POINT('Ctrl Pts',(-205.643432832005,61.8697676638397,4.71215338315388));
#18595=CARTESIAN_POINT('Ctrl Pts',(-202.717111063532,62.7637579756671,4.87106170195819));
#18596=CARTESIAN_POINT('Ctrl Pts',(-201.883716356637,65.7079099813863,5.0299700207625));
#18597=CARTESIAN_POINT('Ctrl Pts',(-203.907295663918,68.003058028335,5.18887833956681));
#18598=CARTESIAN_POINT('Ctrl Pts',(-206.932654093589,67.5450360394643,5.34778665837111));
#18599=CARTESIAN_POINT('Ctrl Pts',(-208.186176851132,64.7537534549547,5.50669497717542));
#18600=CARTESIAN_POINT('Ctrl Pts',(-206.518648282798,62.1882269506957,5.66560329597972));
#18601=CARTESIAN_POINT('Ctrl Pts',(-203.458839942412,62.200502551433,5.82451161478403));
#18602=CARTESIAN_POINT('Ctrl Pts',(-201.811949917596,64.7793261236122,5.98341993358834));
#18603=CARTESIAN_POINT('Ctrl Pts',(-203.087828576151,67.5604610392376,6.14232825239265));
#18604=CARTESIAN_POINT('Ctrl Pts',(-206.116764624146,67.9941938918335,6.30123657119695));
#18605=CARTESIAN_POINT('Ctrl Pts',(-208.121863346572,65.6828832498826,6.46014489000126));
#18606=CARTESIAN_POINT('Ctrl Pts',(-207.264872645281,62.7455128768842,6.61905320880557));
#18607=CARTESIAN_POINT('Ctrl Pts',(-204.33147201681,61.8750311004219,6.77796152760987));
#18608=CARTESIAN_POINT('Ctrl Pts',(-202.010970371329,63.8694858839615,6.93686984641418));
#18609=CARTESIAN_POINT('Ctrl Pts',(-202.430777681647,66.9003833735627,7.09577816521848));
#18610=CARTESIAN_POINT('Ctrl Pts',(-205.206019297764,68.1890306264736,7.25468648402279));
#18611=CARTESIAN_POINT('Ctrl Pts',(-207.792384724327,66.5540102441695,7.4135948028271));
#18612=CARTESIAN_POINT('Ctrl Pts',(-207.818723045533,63.494290638862,7.57250312163141));
#18613=CARTESIAN_POINT('Ctrl Pts',(-205.260887582879,61.8149885468436,7.73141144043571));
#18614=CARTESIAN_POINT('Ctrl Pts',(-202.463873300128,63.0556693568644,7.89031975924003));
#18615=CARTESIAN_POINT('Ctrl Pts',(-201.991951630056,66.0788907691303,8.04922807804431));
#18616=CARTESIAN_POINT('Ctrl Pts',(-204.277775085214,68.1129971827966,8.20813639684864));
#18617=CARTESIAN_POINT('Ctrl Pts',(-207.225726270089,67.2931425726009,8.36704471565293));
#18618=CARTESIAN_POINT('Ctrl Pts',(-208.133156487029,64.370960481825,8.52595303445724));
#18619=CARTESIAN_POINT('Ctrl Pts',(-206.168143855303,62.0254747906674,8.68486135326155));
#18620=CARTESIAN_POINT('Ctrl Pts',(-203.132189993138,62.4070005657726,8.84376967206587));
#18621=CARTESIAN_POINT('Ctrl Pts',(-201.808623469137,65.1657592407589,9.00267799087016));
#18622=CARTESIAN_POINT('Ctrl Pts',(-203.410875279276,67.7725516964743,9.16158630967448));
#18623=CARTESIAN_POINT('Ctrl Pts',(-206.470018872056,67.8374997450991,9.32049462847877));
#18624=CARTESIAN_POINT('Ctrl Pts',(-208.181465593032,65.301059741565,9.47940294728309));
#18625=CARTESIAN_POINT('Ctrl Pts',(-206.9761802169,62.4886115318467,9.63831126608739));
#18626=CARTESIAN_POINT('Ctrl Pts',(-203.959154905271,61.9785762004616,9.7972195848917));
#18627=CARTESIAN_POINT('Ctrl Pts',(-201.89636474318,64.2385484386642,9.95612790369601));
#18628=CARTESIAN_POINT('Ctrl Pts',(-202.678952695852,67.1966109577127,10.1150362225003));
#18629=CARTESIAN_POINT('Ctrl Pts',(-205.589450875101,68.1408451017969,10.2739445413046));
#18630=CARTESIAN_POINT('Ctrl Pts',(-207.959547080228,66.2055875611298,10.4328528601089));
#18631=CARTESIAN_POINT('Ctrl Pts',(-207.616363600448,63.165060819022,10.5917611789132));
#18632=CARTESIAN_POINT('Ctrl Pts',(-204.874527214332,61.8067858092989,10.7506694977175));
#18633=CARTESIAN_POINT('Ctrl Pts',(-202.247722875733,63.3760138797158,10.9095778165218));
#18634=CARTESIAN_POINT('Ctrl Pts',(-202.144175443029,66.4340942742521,11.0684861353262));
#18635=CARTESIAN_POINT('Ctrl Pts',(-204.658816045196,68.1774130667293,11.2273944541305));
#18636=CARTESIAN_POINT('Ctrl Pts',(-207.486250283784,67.007715072918,11.3863027729348));
#18637=CARTESIAN_POINT('Ctrl Pts',(-208.034318050505,63.9973663400718,11.5452110917391));
#18638=CARTESIAN_POINT('Ctrl Pts',(-205.800556942468,61.9062209404184,11.7041194105434));
#18639=CARTESIAN_POINT('Ctrl Pts',(-202.832854177236,62.6514176040611,11.8630277293477));
#18640=CARTESIAN_POINT('Ctrl Pts',(-201.851966480573,65.5497683586795,12.021936048152));
#18641=CARTESIAN_POINT('Ctrl Pts',(-203.757160729602,67.9440976267103,12.1808443669563));
#18642=CARTESIAN_POINT('Ctrl Pts',(-206.801776130772,67.6393110961385,12.3397526857606));
#18643=CARTESIAN_POINT('Ctrl Pts',(-208.194543313332,64.9148336516718,12.4986610045649));
#18644=CARTESIAN_POINT('Ctrl Pts',(-206.658588890975,62.2684357634442,12.6575693233692));
#18645=CARTESIAN_POINT('Ctrl Pts',(-203.602058711086,62.1263054372066,12.8164776421735));
#18646=CARTESIAN_POINT('Ctrl Pts',(-201.827145480354,64.6187461673567,12.9753859609778));
#18647=CARTESIAN_POINT('Ctrl Pts',(-202.961069810931,67.4607161502669,13.1342942797821));
#18648=CARTESIAN_POINT('Ctrl Pts',(-205.964262550072,68.0467290691411,13.2932025985864));
#18649=CARTESIAN_POINT('Ctrl Pts',(-208.08343016082,65.8395348308842,13.4521109173908));
#18650=CARTESIAN_POINT('Ctrl Pts',(-207.37574346268,62.8626644413404,13.611019236195));
#18651=CARTESIAN_POINT('Ctrl Pts',(-204.490001711787,61.8452794067929,13.7699275549994));
#18652=CARTESIAN_POINT('Ctrl Pts',(-202.071820690067,63.7201069454906,13.9288358738037));
#18653=CARTESIAN_POINT('Ctrl Pts',(-202.338161734746,66.768326145764,14.087744192608));
#18654=CARTESIAN_POINT('Ctrl Pts',(-205.044846344621,68.1953636703757,14.2466525114123));
#18655=CARTESIAN_POINT('Ctrl Pts',(-207.710416338458,66.692927556513,14.4055608302166));
#18656=CARTESIAN_POINT('Ctrl Pts',(-207.891106903343,63.6384342555754,14.5644691490209));
#18657=CARTESIAN_POINT('Ctrl Pts',(-205.421263021166,61.8322094680282,14.7233774678252));
#18658=CARTESIAN_POINT('Ctrl Pts',(-202.565209809467,62.9301791057216,14.8822857866295));
#18659=CARTESIAN_POINT('Ctrl Pts',(-201.941345237341,65.9257384937735,15.0411941054338));
#18660=CARTESIAN_POINT('Ctrl Pts',(-204.121620741519,68.0725889368547,15.2001024242381));
#18661=CARTESIAN_POINT('Ctrl Pts',(-207.107185405563,67.4025287969464,15.3590107430424));
#18662=CARTESIAN_POINT('Ctrl Pts',(-208.160904243891,64.5298476130291,15.5179190618467));
#18663=CARTESIAN_POINT('Ctrl Pts',(-206.316745100461,62.0882164301626,15.676827380651));
#18664=CARTESIAN_POINT('Ctrl Pts',(-203.26540114856,62.3160356393736,15.8357356994554));
#18665=CARTESIAN_POINT('Ctrl Pts',(-201.80433371747,65.0045662149023,15.9946440182597));
#18666=CARTESIAN_POINT('Ctrl Pts',(-203.27298513606,67.6887400042411,16.153552337064));
#18667=CARTESIAN_POINT('Ctrl Pts',(-206.325010933901,67.908258063909,16.3124606558683));
#18668=CARTESIAN_POINT('Ctrl Pts',(-208.162144747655,65.4607949079353,16.4713689746726));
#18669=CARTESIAN_POINT('Ctrl Pts',(-207.100541451971,62.5923678564539,16.6302772934769));
#18670=CARTESIAN_POINT('Ctrl Pts',(-204.112613754326,61.9281555284998,16.7891856122812));
#18671=CARTESIAN_POINT('Ctrl Pts',(-201.939478088485,64.086503084628,16.9480939310855));
#18672=CARTESIAN_POINT('Ctrl Pts',(-202.36110058667,66.0727092589846,17.0540328102884));
#18673=CARTESIAN_POINT('Ctrl Pts',(-202.945668449658,66.7564253212267,17.1070022498898));
#18674=CARTESIAN_POINT('Ctrl Pts',(-204.349800002025,62.567913197965,-0.321006749669432));
#18675=CARTESIAN_POINT('Ctrl Pts',(-203.540360643981,62.7843106836636,-0.268037310067997));
#18676=CARTESIAN_POINT('Ctrl Pts',(-202.168802483164,64.0864608745682,-0.162098430865125));
#18677=CARTESIAN_POINT('Ctrl Pts',(-202.69814130666,66.8897415984097,-0.00319011206081897));
#18678=CARTESIAN_POINT('Ctrl Pts',(-205.342093295844,67.9563291423292,0.155718206743488));
#18679=CARTESIAN_POINT('Ctrl Pts',(-207.670356669564,66.3146464051101,0.314626525547794));
#18680=CARTESIAN_POINT('Ctrl Pts',(-207.551468167857,63.4667172744462,0.4735348443521));
#18681=CARTESIAN_POINT('Ctrl Pts',(-205.092935872386,62.0249672107152,0.632443163156408));
#18682=CARTESIAN_POINT('Ctrl Pts',(-202.549437234532,63.310459551055,0.791351481960714));
#18683=CARTESIAN_POINT('Ctrl Pts',(-202.252472399597,66.1450175587076,0.950259800765021));
#18684=CARTESIAN_POINT('Ctrl Pts',(-204.474465902543,67.9297809531409,1.10916811956933));
#18685=CARTESIAN_POINT('Ctrl Pts',(-207.178236114389,67.0285807845878,1.26807643837363));
#18686=CARTESIAN_POINT('Ctrl Pts',(-207.885036955817,64.2675873735086,1.42698475717794));
#18687=CARTESIAN_POINT('Ctrl Pts',(-205.946861772035,62.1780680127346,1.58589307598225));
#18688=CARTESIAN_POINT('Ctrl Pts',(-203.140617402382,62.67566127779,1.74480139478655));
#18689=CARTESIAN_POINT('Ctrl Pts',(-202.039032708539,65.304183800853,1.90370971359086));
#18690=CARTESIAN_POINT('Ctrl Pts',(-203.652030465805,67.6538332883171,2.06261803239516));
#18691=CARTESIAN_POINT('Ctrl Pts',(-206.50083127026,67.5704784314428,2.22152635119948));
#18692=CARTESIAN_POINT('Ctrl Pts',(-207.97368691345,65.1305375068299,2.38043467000378));
#18693=CARTESIAN_POINT('Ctrl Pts',(-206.720299546718,62.5709213382542,2.53934298880809));
#18694=CARTESIAN_POINT('Ctrl Pts',(-203.88976082377,62.2382572969888,2.6982513076124));
#18695=CARTESIAN_POINT('Ctrl Pts',(-202.077076948865,64.4375281180749,2.8571596264167));
#18696=CARTESIAN_POINT('Ctrl Pts',(-202.944096267957,67.1524668643289,3.01606794522101));
#18697=CARTESIAN_POINT('Ctrl Pts',(-205.6959451455,67.8940480516819,3.17497626402531));
#18698=CARTESIAN_POINT('Ctrl Pts',(-207.809759294355,65.9823983291764,3.33388458282962));
#18699=CARTESIAN_POINT('Ctrl Pts',(-207.34761752514,63.1700967996395,3.49279290163393));
#18700=CARTESIAN_POINT('Ctrl Pts',(-204.733206248249,62.0354300712118,3.65170122043824));
#18701=CARTESIAN_POINT('Ctrl Pts',(-202.363388500804,63.6186479193701,3.81060953924254));
#18702=CARTESIAN_POINT('Ctrl Pts',(-202.410786707087,66.4682739158379,3.96951785804685));
#18703=CARTESIAN_POINT('Ctrl Pts',(-204.831946721149,67.9718027969204,4.12842617685115));
#18704=CARTESIAN_POINT('Ctrl Pts',(-207.407176102995,66.7508160889821,4.28733449565546));
#18705=CARTESIAN_POINT('Ctrl Pts',(-207.77553333811,63.9247007591889,4.44624281445977));
#18706=CARTESIAN_POINT('Ctrl Pts',(-205.599312630415,62.0844077549669,4.60515113326408));
#18707=CARTESIAN_POINT('Ctrl Pts',(-202.873648801545,62.9170971340231,4.76405945206838));
#18708=CARTESIAN_POINT('Ctrl Pts',(-202.097399985633,65.6593685804304,4.92296777087269));
#18709=CARTESIAN_POINT('Ctrl Pts',(-203.982222421131,67.7971382819264,5.08187608967699));
#18710=CARTESIAN_POINT('Ctrl Pts',(-206.800131965447,67.370522869588,5.2407844084813));
#18711=CARTESIAN_POINT('Ctrl Pts',(-207.967700643544,64.7706385852557,5.39969272728561));
#18712=CARTESIAN_POINT('Ctrl Pts',(-206.414514541016,62.3810302824357,5.55860104608992));
#18713=CARTESIAN_POINT('Ctrl Pts',(-203.564517317021,62.3924641449957,5.71750936489422));
#18714=CARTESIAN_POINT('Ctrl Pts',(-202.030554572688,64.7944577355345,5.87641768369853));
#18715=CARTESIAN_POINT('Ctrl Pts',(-203.218946207237,67.3848901768319,6.03532600250283));
#18716=CARTESIAN_POINT('Ctrl Pts',(-206.040188052521,67.7888819594342,6.19423432130714));
#18717=CARTESIAN_POINT('Ctrl Pts',(-207.907797117221,65.6360579323843,6.35314264011145));
#18718=CARTESIAN_POINT('Ctrl Pts',(-207.1095702847,62.9001031020125,6.51205095891576));
#18719=CARTESIAN_POINT('Ctrl Pts',(-204.377312993397,62.089310277602,6.67095927772006));
#18720=CARTESIAN_POINT('Ctrl Pts',(-202.215928190104,63.9470052585089,6.82986759652437));
#18721=CARTESIAN_POINT('Ctrl Pts',(-202.606949305129,66.7700740493103,6.98877591532868));
#18722=CARTESIAN_POINT('Ctrl Pts',(-205.191892550579,67.9703587354556,7.14768423413298));
#18723=CARTESIAN_POINT('Ctrl Pts',(-207.600910850401,66.4474517320208,7.30659255293729));
#18724=CARTESIAN_POINT('Ctrl Pts',(-207.625443152419,63.597537158538,7.4655008717416));
#18725=CARTESIAN_POINT('Ctrl Pts',(-205.242998516334,62.0333848430704,7.6244091905459));
#18726=CARTESIAN_POINT('Ctrl Pts',(-202.637775556419,63.1889921462316,7.78331750935021));
#18727=CARTESIAN_POINT('Ctrl Pts',(-202.198213564284,66.0049112084673,7.94222582815451));
#18728=CARTESIAN_POINT('Ctrl Pts',(-204.327298061427,67.8995389064651,8.10113414695883));
#18729=CARTESIAN_POINT('Ctrl Pts',(-207.073108177202,67.1359017425625,8.26004246576313));
#18730=CARTESIAN_POINT('Ctrl Pts',(-207.918315886821,64.4140937336109,8.41895078456743));
#18731=CARTESIAN_POINT('Ctrl Pts',(-206.088044208815,62.2294380411316,8.57785910337174));
#18732=CARTESIAN_POINT('Ctrl Pts',(-203.260265761013,62.5848025865447,8.73676742217605));
#18733=CARTESIAN_POINT('Ctrl Pts',(-202.027456218864,65.1543931264515,8.89567574098036));
#18734=CARTESIAN_POINT('Ctrl Pts',(-203.519841591753,67.5824377736476,9.05458405978466));
#18735=CARTESIAN_POINT('Ctrl Pts',(-206.369219649899,67.6429323333367,9.21349237858897));
#18736=CARTESIAN_POINT('Ctrl Pts',(-207.963312436502,65.2804160693309,9.37240069739327));
#18737=CARTESIAN_POINT('Ctrl Pts',(-206.840673501651,62.6608174871151,9.53130901619759));
#18738=CARTESIAN_POINT('Ctrl Pts',(-204.030525673313,62.1857552881527,9.69021733500189));
#18739=CARTESIAN_POINT('Ctrl Pts',(-202.109181072068,64.2907611867807,9.8491256538062));
#18740=CARTESIAN_POINT('Ctrl Pts',(-202.838106953866,67.0459893023525,10.0080339726105));
#18741=CARTESIAN_POINT('Ctrl Pts',(-205.549032217327,67.925477293127,10.1669422914148));
#18742=CARTESIAN_POINT('Ctrl Pts',(-207.756610880363,66.1229203990175,10.3258506102191));
#18743=CARTESIAN_POINT('Ctrl Pts',(-207.436959498352,63.2908826337379,10.4847589290234));
#18744=CARTESIAN_POINT('Ctrl Pts',(-204.883130885644,62.0257445673959,10.6436672478277));
#18745=CARTESIAN_POINT('Ctrl Pts',(-202.436446570756,63.4873706390274,10.802575566632));
#18746=CARTESIAN_POINT('Ctrl Pts',(-202.339999387492,66.3357584024529,10.9614838854363));
#18747=CARTESIAN_POINT('Ctrl Pts',(-204.682211035499,67.9595377920051,11.1203922042407));
#18748=CARTESIAN_POINT('Ctrl Pts',(-207.315768054299,66.870046011989,11.279300523045));
#18749=CARTESIAN_POINT('Ctrl Pts',(-207.826254803778,64.0661169492992,11.4382088418493));
#18750=CARTESIAN_POINT('Ctrl Pts',(-205.74566273762,62.1183614296738,11.5971171606536));
#18751=CARTESIAN_POINT('Ctrl Pts',(-202.98145540773,62.8124599438455,11.7560254794579));
#18752=CARTESIAN_POINT('Ctrl Pts',(-202.067827199178,65.5120707318156,11.9149337982622));
#18753=CARTESIAN_POINT('Ctrl Pts',(-203.84238224213,67.7422207961682,12.0738421170665));
#18754=CARTESIAN_POINT('Ctrl Pts',(-206.678228307043,67.4583334838238,12.2327504358708));
#18755=CARTESIAN_POINT('Ctrl Pts',(-207.975493417271,64.9206735098047,12.3916587546751));
#18756=CARTESIAN_POINT('Ctrl Pts',(-206.544859419016,62.4557391753607,12.5505670734794));
#18757=CARTESIAN_POINT('Ctrl Pts',(-203.697915571989,62.3233547283102,12.7094753922837));
#18758=CARTESIAN_POINT('Ctrl Pts',(-202.044708175418,64.644888749949,12.868383711088));
#18759=CARTESIAN_POINT('Ctrl Pts',(-203.100879292971,67.2919847968046,13.0272920298923));
#18760=CARTESIAN_POINT('Ctrl Pts',(-205.89814304858,67.8378147986296,13.1862003486966));
#18761=CARTESIAN_POINT('Ctrl Pts',(-207.871999295751,65.7819679114821,13.3451086675009));
#18762=CARTESIAN_POINT('Ctrl Pts',(-207.21283868803,63.0092215814544,13.5040169863053));
#18763=CARTESIAN_POINT('Ctrl Pts',(-204.524972304159,62.0615986581739,13.6629253051096));
#18764=CARTESIAN_POINT('Ctrl Pts',(-202.272606001323,63.8078692367045,13.8218336239139));
#18765=CARTESIAN_POINT('Ctrl Pts',(-202.520684035478,66.6470719881461,13.9807419427182));
#18766=CARTESIAN_POINT('Ctrl Pts',(-205.041771229913,67.9762575224163,14.1396502615225));
#18767=CARTESIAN_POINT('Ctrl Pts',(-207.524563038319,66.5768434816013,14.2985585803268));
#18768=CARTESIAN_POINT('Ctrl Pts',(-207.692863647714,63.7317968446979,14.4574668991311));
#18769=CARTESIAN_POINT('Ctrl Pts',(-205.392377007752,62.0494249253602,14.6163752179354));
#18770=CARTESIAN_POINT('Ctrl Pts',(-202.732163419374,63.0721067640084,14.7752835367397));
#18771=CARTESIAN_POINT('Ctrl Pts',(-202.151077252885,65.8622605875592,14.934191855544));
#18772=CARTESIAN_POINT('Ctrl Pts',(-204.181851224064,67.8619014547198,15.0931001743483));
#18773=CARTESIAN_POINT('Ctrl Pts',(-206.962695662023,67.2377873514137,15.2520084931526));
#18774=CARTESIAN_POINT('Ctrl Pts',(-207.944160979464,64.562085971191,15.4109168119569));
#18775=CARTESIAN_POINT('Ctrl Pts',(-206.226455863752,62.2878774852072,15.5698251307612));
#18776=CARTESIAN_POINT('Ctrl Pts',(-203.384342624961,62.5000751268878,15.7287334495655));
#18777=CARTESIAN_POINT('Ctrl Pts',(-202.02346061555,65.0042531094591,15.8876417683698));
#18778=CARTESIAN_POINT('Ctrl Pts',(-203.391406578293,67.504373050753,16.0465500871742));
#18779=CARTESIAN_POINT('Ctrl Pts',(-206.234154908835,67.7088387528733,16.2054584059785));
#18780=CARTESIAN_POINT('Ctrl Pts',(-207.945316421862,65.4291981922897,16.3643667247828));
#18781=CARTESIAN_POINT('Ctrl Pts',(-206.956507284456,62.7574592385606,16.5232750435871));
#18782=CARTESIAN_POINT('Ctrl Pts',(-204.173461846155,62.1387919626312,16.6821833623914));
#18783=CARTESIAN_POINT('Ctrl Pts',(-202.149338134461,64.1491415855772,16.8410916811957));
#18784=CARTESIAN_POINT('Ctrl Pts',(-202.542049969887,65.9991535645903,16.9470305603986));
#18785=CARTESIAN_POINT('Ctrl Pts',(-203.086534003335,66.6359872033749,17.));
#18786=CARTESIAN_POINT('Ctrl Pts',(-202.485823128102,65.0013539996937,0.887416697508052));
#18787=CARTESIAN_POINT('Ctrl Pts',(-202.484195200284,65.3337573103262,0.908364398593722));
#18788=CARTESIAN_POINT('Ctrl Pts',(-202.545417687543,65.6655864079193,0.929312099679392));
#18789=CARTESIAN_POINT('Ctrl Pts',(-202.672298789244,65.9700517898377,0.950259800765062));
#18790=CARTESIAN_POINT('Ctrl Pts',(-202.993136900579,66.7399386901854,1.0032292403665));
#18791=CARTESIAN_POINT('Ctrl Pts',(-203.733801401561,67.3348598216632,1.05619867996793));
#18792=CARTESIAN_POINT('Ctrl Pts',(-204.554762020693,67.4821203593099,1.10916811956937));
#18793=CARTESIAN_POINT('Ctrl Pts',(-205.375722639825,67.6293808969566,1.1621375591708));
#18794=CARTESIAN_POINT('Ctrl Pts',(-206.276979377107,67.3289808407722,1.21510699877224));
#18795=CARTESIAN_POINT('Ctrl Pts',(-206.845407885986,66.7186152441669,1.26807643837368));
#18796=CARTESIAN_POINT('Ctrl Pts',(-207.413836394865,66.1082496475615,1.32104587797511));
#18797=CARTESIAN_POINT('Ctrl Pts',(-207.649436675341,65.187918510535,1.37401531757655));
#18798=CARTESIAN_POINT('Ctrl Pts',(-207.444207618282,64.3794997152261,1.42698475717798));
#18799=CARTESIAN_POINT('Ctrl Pts',(-207.238978561223,63.5710809199172,1.47995419677942));
#18800=CARTESIAN_POINT('Ctrl Pts',(-206.592920166629,62.8745744663259,1.53292363638085));
#18801=CARTESIAN_POINT('Ctrl Pts',(-205.80218357439,62.6092534503727,1.58589307598229));
#18802=CARTESIAN_POINT('Ctrl Pts',(-205.011446982151,62.3439324344196,1.63886251558373));
#18803=CARTESIAN_POINT('Ctrl Pts',(-204.076032192267,62.5097968561048,1.69183195518516));
#18804=CARTESIAN_POINT('Ctrl Pts',(-203.424727348351,63.0308161541245,1.7448013947866));
#18805=CARTESIAN_POINT('Ctrl Pts',(-202.840201389118,63.4984148643111,1.79233982902708));
#18806=CARTESIAN_POINT('Ctrl Pts',(-202.48451199895,64.2520733360095,1.83987826326757));
#18807=CARTESIAN_POINT('Ctrl Pts',(-202.479332509853,65.0014637523716,1.88741669750805));
#18808=CARTESIAN_POINT('Ctrl Pts',(-204.206200717467,62.0307770462543,-5.55111512312578E-16));
#18809=CARTESIAN_POINT('Ctrl Pts',(-204.113162249417,62.0648109334671,-5.19915500288305E-16));
#18810=CARTESIAN_POINT('Ctrl Pts',(-204.02219118159,62.1036166453176,-4.84452877073069E-16));
#18811=CARTESIAN_POINT('Ctrl Pts',(-203.93349495337,62.1468647837849,-4.82253126321552E-16));
#18812=CARTESIAN_POINT('Ctrl Pts',(-203.842820762435,62.1910773736963,-4.80004320214958E-16));
#18813=CARTESIAN_POINT('Ctrl Pts',(-203.754523335469,62.239933353,-9.13199113811134E-16));
#18814=CARTESIAN_POINT('Ctrl Pts',(-203.668853233392,62.2931263628092,-1.02001740387436E-15));
#18815=CARTESIAN_POINT('Ctrl Pts',(-203.585825130324,62.3446789417594,-1.1235415013366E-15));
#18816=CARTESIAN_POINT('Ctrl Pts',(-203.505264469594,62.4003060362145,-6.67670990993899E-16));
#18817=CARTESIAN_POINT('Ctrl Pts',(-203.42743316137,62.4597595642908,-7.49400541621981E-16));
#18818=CARTESIAN_POINT('Ctrl Pts',(-203.359330766673,62.5117814013576,-8.20913898421552E-16));
#18819=CARTESIAN_POINT('Ctrl Pts',(-203.293318330331,62.5667335723465,-9.45964652035114E-16));
#18820=CARTESIAN_POINT('Ctrl Pts',(-203.229596673155,62.6244628960252,-9.78384040450919E-16));
#18821=CARTESIAN_POINT('Ctrl Pts',(-203.216348740433,62.6364650037874,-9.85124133155235E-16));
#18822=CARTESIAN_POINT('Ctrl Pts',(-203.203198172353,62.6485889403755,-3.4496231498821E-16));
#18823=CARTESIAN_POINT('Ctrl Pts',(-203.190163654011,62.6608172960224,-3.46944695195361E-16));
#18824=CARTESIAN_POINT('Ctrl Pts',(-203.11774011012,62.7287615674313,-3.57959371470727E-16));
#18825=CARTESIAN_POINT('Ctrl Pts',(-203.048782373238,62.8000276808216,-5.09072278378989E-16));
#18826=CARTESIAN_POINT('Ctrl Pts',(-202.983529572481,62.8743236281409,-5.13478148889135E-16));
#18827=CARTESIAN_POINT('Ctrl Pts',(-202.918635349275,62.9482113039592,-5.17859808235267E-16));
#18828=CARTESIAN_POINT('Ctrl Pts',(-202.857404970179,63.0250964056677,-2.66956613222884E-16));
#18829=CARTESIAN_POINT('Ctrl Pts',(-202.800117264857,63.1047184530433,-2.22044604925031E-16));
#18830=CARTESIAN_POINT('Ctrl Pts',(-202.744165764651,63.1824833587091,-1.78180145222485E-16));
#18831=CARTESIAN_POINT('Ctrl Pts',(-202.691974876248,63.2628597651003,-1.00656795420818E-15));
#18832=CARTESIAN_POINT('Ctrl Pts',(-202.643851527184,63.3456191713536,-1.0547118733939E-15));
#18833=CARTESIAN_POINT('Ctrl Pts',(-202.623072180899,63.3813541398117,-1.0755001017227E-15));
#18834=CARTESIAN_POINT('Ctrl Pts',(-202.60305183952,63.4175335255461,-2.58501556813931E-16));
#18835=CARTESIAN_POINT('Ctrl Pts',(-202.58381822777,63.454139265439,-1.94289029309402E-16));
#18836=CARTESIAN_POINT('Ctrl Pts',(-202.569903820985,63.480621403177,-1.47834975850494E-16));
#18837=CARTESIAN_POINT('Ctrl Pts',(-202.556401202133,63.5073266847522,-7.93899856949203E-16));
#18838=CARTESIAN_POINT('Ctrl Pts',(-202.5433215057,63.5342482737999,-8.32667268468867E-16));
#18839=CARTESIAN_POINT('Ctrl Pts',(-202.537160097315,63.5469301357491,-8.50929301967292E-16));
#18840=CARTESIAN_POINT('Ctrl Pts',(-202.531094723709,63.5596556012092,-3.63050352889582E-16));
#18841=CARTESIAN_POINT('Ctrl Pts',(-202.525129549917,63.5724168279603,-3.7470027081099E-16));
#18842=CARTESIAN_POINT('Ctrl Pts',(-202.485113190241,63.6580233597082,-4.52851775196109E-16));
#18843=CARTESIAN_POINT('Ctrl Pts',(-202.449555061626,63.7453341587585,2.75905776866127E-16));
#18844=CARTESIAN_POINT('Ctrl Pts',(-202.418706882959,63.8341116308705,2.22044604925031E-16));
#18845=CARTESIAN_POINT('Ctrl Pts',(-202.388542894157,63.9209200840876,1.6937803407733E-16));
#18846=CARTESIAN_POINT('Ctrl Pts',(-202.362882030333,64.0091315459226,-9.1941220868861E-16));
#18847=CARTESIAN_POINT('Ctrl Pts',(-202.342008814717,64.0985324360296,-8.32667268468867E-16));
#18848=CARTESIAN_POINT('Ctrl Pts',(-202.338628814105,64.1130091256228,-8.18620656943663E-16));
#18849=CARTESIAN_POINT('Ctrl Pts',(-202.335374462847,64.1275170099365,-5.95910370058754E-16));
#18850=CARTESIAN_POINT('Ctrl Pts',(-202.332247099787,64.1420551858173,-5.82867087928207E-16));
#18851=CARTESIAN_POINT('Ctrl Pts',(-202.312208792581,64.2352072851979,-4.99293390427251E-16));
#18852=CARTESIAN_POINT('Ctrl Pts',(-202.297379875413,64.3296040558921,-8.33690503982433E-17));
#18853=CARTESIAN_POINT('Ctrl Pts',(-202.287681750639,64.4248371114872,-5.55111512312578E-17));
#18854=CARTESIAN_POINT('Ctrl Pts',(-202.284325955759,64.4577901418682,-4.58716180684954E-17));
#18855=CARTESIAN_POINT('Ctrl Pts',(-202.28158492797,64.4908431751708,-8.28167483116791E-16));
#18856=CARTESIAN_POINT('Ctrl Pts',(-202.279456765112,64.5239787674251,-8.60422844084496E-16));
#18857=CARTESIAN_POINT('Ctrl Pts',(-202.278429684535,64.5399704586003,-8.75989723570996E-16));
#18858=CARTESIAN_POINT('Ctrl Pts',(-202.277545359971,64.555981373961,-8.02943466711267E-16));
#18859=CARTESIAN_POINT('Ctrl Pts',(-202.276803632431,64.5720095213841,-8.04911692853238E-16));
#18860=CARTESIAN_POINT('Ctrl Pts',(-202.276227016754,64.5844697315966,-8.06441783064374E-16));
#18861=CARTESIAN_POINT('Ctrl Pts',(-202.275736678019,64.5969392095638,-5.87596457671717E-16));
#18862=CARTESIAN_POINT('Ctrl Pts',(-202.275332691875,64.6094071262613,-5.82867087928207E-16));
#18863=CARTESIAN_POINT('Ctrl Pts',(-202.272313622363,64.702582369262,-5.47523558950325E-16));
#18864=CARTESIAN_POINT('Ctrl Pts',(-202.27410534735,64.7958212167759,-9.81423475480654E-16));
#18865=CARTESIAN_POINT('Ctrl Pts',(-202.280568163262,64.8887492259718,-9.15933995315754E-16));
#18866=CARTESIAN_POINT('Ctrl Pts',(-202.28704447601,64.9818713044648,-8.50307748018024E-16));
#18867=CARTESIAN_POINT('Ctrl Pts',(-202.298211793817,65.0746822257257,-8.07734983664408E-16));
#18868=CARTESIAN_POINT('Ctrl Pts',(-202.313980610279,65.1667932227156,-7.49400541621981E-16));
#18869=CARTESIAN_POINT('Ctrl Pts',(-202.329528117816,65.257611479329,-6.91884799745999E-16));
#18870=CARTESIAN_POINT('Ctrl Pts',(-202.349549338359,65.3477501671012,-2.84670909400231E-16));
#18871=CARTESIAN_POINT('Ctrl Pts',(-202.374001557502,65.4368115389553,-1.94289029309402E-16));
#18872=CARTESIAN_POINT('Ctrl Pts',(-202.383514216169,65.4714591276246,-1.59127722680513E-16));
#18873=CARTESIAN_POINT('Ctrl Pts',(-202.393697911918,65.5059433314471,-4.85030275451525E-16));
#18874=CARTESIAN_POINT('Ctrl Pts',(-202.404551700249,65.5402392680712,-4.71844785465692E-16));
#18875=CARTESIAN_POINT('Ctrl Pts',(-202.410350726718,65.5585631047066,-4.64799963593452E-16));
#18876=CARTESIAN_POINT('Ctrl Pts',(-202.41634105309,65.5768331827315,-6.36029965202052E-16));
#18877=CARTESIAN_POINT('Ctrl Pts',(-202.422522630952,65.5950455929995,-6.38378239159465E-16));
#18878=CARTESIAN_POINT('Ctrl Pts',(-202.428041241916,65.6113047438546,-6.40474663518505E-16));
#18879=CARTESIAN_POINT('Ctrl Pts',(-202.433712823702,65.6275191792443,-1.66152285628493E-16));
#18880=CARTESIAN_POINT('Ctrl Pts',(-202.43953101583,65.6436691493443,-1.66533453693773E-16));
#18881=CARTESIAN_POINT('Ctrl Pts',(-202.470364649952,65.7292562627001,-1.68553462041071E-16));
#18882=CARTESIAN_POINT('Ctrl Pts',(-202.505348644146,65.8131450789626,4.41371823884456E-16));
#18883=CARTESIAN_POINT('Ctrl Pts',(-202.544418722017,65.8949548979899,0.));
#18884=CARTESIAN_POINT('Ctrl Pts',(-202.575881626623,65.9608358655278,-3.55434141613069E-16));
#18885=CARTESIAN_POINT('Ctrl Pts',(-202.609995265414,66.0253683017606,-7.18594950445821E-16));
#18886=CARTESIAN_POINT('Ctrl Pts',(-202.646744272941,66.0883356853988,-5.55111512312578E-16));
#18887=CARTESIAN_POINT('Ctrl Pts',(-202.661986555904,66.1144524908179,-4.87303944389755E-16));
#18888=CARTESIAN_POINT('Ctrl Pts',(-202.677682386268,66.1402998412242,-7.97734533373392E-16));
#18889=CARTESIAN_POINT('Ctrl Pts',(-202.69383140079,66.1658612939494,-7.7715611723761E-16));
#18890=CARTESIAN_POINT('Ctrl Pts',(-202.702298041279,66.1792627080302,-7.66367220427743E-16));
#18891=CARTESIAN_POINT('Ctrl Pts',(-202.710887832138,66.1925831745098,-5.40710766792841E-17));
#18892=CARTESIAN_POINT('Ctrl Pts',(-202.719595914358,66.2058134485369,-1.11022302462516E-16));
#18893=CARTESIAN_POINT('Ctrl Pts',(-202.767005259998,66.2778429285551,-4.21081426798669E-16));
#18894=CARTESIAN_POINT('Ctrl Pts',(-202.817957067113,66.3472640345857,-9.3988901168733E-16));
#18895=CARTESIAN_POINT('Ctrl Pts',(-202.87241461149,66.4137214114329,-7.7715611723761E-16));
#18896=CARTESIAN_POINT('Ctrl Pts',(-202.926872155867,66.4801787882801,-6.14423222787889E-16));
#18897=CARTESIAN_POINT('Ctrl Pts',(-202.984835768426,66.5436731279146,-3.7164630165585E-17));
#18898=CARTESIAN_POINT('Ctrl Pts',(-203.04629821927,66.6038050748561,-2.22044604925031E-16));
#18899=CARTESIAN_POINT('Ctrl Pts',(-203.058349034853,66.6155950212913,-2.58104842041481E-16));
#18900=CARTESIAN_POINT('Ctrl Pts',(-203.070534438641,66.627255553132,-2.14870316912335E-16));
#18901=CARTESIAN_POINT('Ctrl Pts',(-203.082851846776,66.6387856087136,-2.22044604925031E-16));
#18902=CARTESIAN_POINT('Origin',(-205.,65.,9.));
#18903=CARTESIAN_POINT('Origin',(-205.,-95.,17.));
#18904=CARTESIAN_POINT('Ctrl Pts',(-203.086534003335,-93.3640127966251,
17.));
#18905=CARTESIAN_POINT('Ctrl Pts',(-203.024408000274,-93.4223959843149,
17.));
#18906=CARTESIAN_POINT('Ctrl Pts',(-202.965660700181,-93.4840340445169,
17.));
#18907=CARTESIAN_POINT('Ctrl Pts',(-202.910302663152,-93.5485502404793,
17.));
#18908=CARTESIAN_POINT('Ctrl Pts',(-202.85358729986,-93.6146483120265,17.));
#18909=CARTESIAN_POINT('Ctrl Pts',(-202.800428974214,-93.6837678789023,
17.));
#18910=CARTESIAN_POINT('Ctrl Pts',(-202.750867981151,-93.7555500875478,
17.));
#18911=CARTESIAN_POINT('Ctrl Pts',(-202.737959277062,-93.7742465508953,
17.));
#18912=CARTESIAN_POINT('Ctrl Pts',(-202.725294786098,-93.7931238635411,
17.));
#18913=CARTESIAN_POINT('Ctrl Pts',(-202.712875593634,-93.8121761152587,
17.));
#18914=CARTESIAN_POINT('Ctrl Pts',(-202.702666953263,-93.8278371646063,
17.));
#18915=CARTESIAN_POINT('Ctrl Pts',(-202.692623587495,-93.8436173779436,
17.));
#18916=CARTESIAN_POINT('Ctrl Pts',(-202.682755039166,-93.8594987232582,
17.));
#18917=CARTESIAN_POINT('Ctrl Pts',(-202.635325956578,-93.9358258195438,
17.));
#18918=CARTESIAN_POINT('Ctrl Pts',(-202.591881662897,-94.014561411206,17.));
#18919=CARTESIAN_POINT('Ctrl Pts',(-202.552455307866,-94.0953124442998,
17.));
#18920=CARTESIAN_POINT('Ctrl Pts',(-202.520329580588,-94.1611107070231,
17.));
#18921=CARTESIAN_POINT('Ctrl Pts',(-202.49087203172,-94.2282482025802,17.));
#18922=CARTESIAN_POINT('Ctrl Pts',(-202.464118359925,-94.2965306954245,
17.));
#18923=CARTESIAN_POINT('Ctrl Pts',(-202.455239584334,-94.3191916944583,
17.));
#18924=CARTESIAN_POINT('Ctrl Pts',(-202.446658750236,-94.3419789158481,
17.));
#18925=CARTESIAN_POINT('Ctrl Pts',(-202.4383775944,-94.3648855717116,17.));
#18926=CARTESIAN_POINT('Ctrl Pts',(-202.431690779773,-94.3833820913431,
17.));
#18927=CARTESIAN_POINT('Ctrl Pts',(-202.425198561125,-94.4019592233538,
17.));
#18928=CARTESIAN_POINT('Ctrl Pts',(-202.418909543929,-94.4205899139815,
17.));
#18929=CARTESIAN_POINT('Ctrl Pts',(-202.389394386736,-94.5080261135151,
17.));
#18930=CARTESIAN_POINT('Ctrl Pts',(-202.364312756292,-94.5967429324199,
17.));
#18931=CARTESIAN_POINT('Ctrl Pts',(-202.343695730977,-94.6863420431789,
17.));
#18932=CARTESIAN_POINT('Ctrl Pts',(-202.322620129767,-94.7779340695863,
17.));
#18933=CARTESIAN_POINT('Ctrl Pts',(-202.306209395933,-94.8704488625012,
17.));
#18934=CARTESIAN_POINT('Ctrl Pts',(-202.294539564163,-94.9634948472204,
17.));
#18935=CARTESIAN_POINT('Ctrl Pts',(-202.283037042173,-95.0552068364273,
17.));
#18936=CARTESIAN_POINT('Ctrl Pts',(-202.27614016437,-95.1474358567499,17.));
#18937=CARTESIAN_POINT('Ctrl Pts',(-202.273968836359,-95.2398261209644,
17.));
#18938=CARTESIAN_POINT('Ctrl Pts',(-202.272844366773,-95.2876724351408,
17.));
#18939=CARTESIAN_POINT('Ctrl Pts',(-202.272988049685,-95.3355622217538,
17.));
#18940=CARTESIAN_POINT('Ctrl Pts',(-202.274422018419,-95.3834468414973,
17.));
#18941=CARTESIAN_POINT('Ctrl Pts',(-202.275072129396,-95.4051560435378,
17.));
#18942=CARTESIAN_POINT('Ctrl Pts',(-202.275988023267,-95.4268712623304,
17.));
#18943=CARTESIAN_POINT('Ctrl Pts',(-202.277169537603,-95.4485498237118,
17.));
#18944=CARTESIAN_POINT('Ctrl Pts',(-202.282380920127,-95.544168871676,17.));
#18945=CARTESIAN_POINT('Ctrl Pts',(-202.29275597009,-95.63918004578,17.));
#18946=CARTESIAN_POINT('Ctrl Pts',(-202.308361643616,-95.7331861624806,
17.));
#18947=CARTESIAN_POINT('Ctrl Pts',(-202.312210372873,-95.7563703006822,
17.));
#18948=CARTESIAN_POINT('Ctrl Pts',(-202.316377475622,-95.7794934013305,
17.));
#18949=CARTESIAN_POINT('Ctrl Pts',(-202.320864419024,-95.8025496616774,
17.));
#18950=CARTESIAN_POINT('Ctrl Pts',(-202.338369892673,-95.8925019347234,
17.));
#18951=CARTESIAN_POINT('Ctrl Pts',(-202.360739472015,-95.9814367403613,
17.));
#18952=CARTESIAN_POINT('Ctrl Pts',(-202.387670003523,-96.0691240547554,
17.));
#18953=CARTESIAN_POINT('Ctrl Pts',(-202.415202635706,-96.1587718425676,
17.));
#18954=CARTESIAN_POINT('Ctrl Pts',(-202.447502661721,-96.2471164356113,
17.));
#18955=CARTESIAN_POINT('Ctrl Pts',(-202.484300312417,-96.3339075926369,
17.));
#18956=CARTESIAN_POINT('Ctrl Pts',(-202.498927651313,-96.3684077208491,
17.));
#18957=CARTESIAN_POINT('Ctrl Pts',(-202.514266241852,-96.4026622798363,
17.));
#18958=CARTESIAN_POINT('Ctrl Pts',(-202.530301312039,-96.4366549706656,
17.));
#18959=CARTESIAN_POINT('Ctrl Pts',(-202.538298082829,-96.453607297903,17.));
#18960=CARTESIAN_POINT('Ctrl Pts',(-202.546469923465,-96.4704979563681,
17.));
#18961=CARTESIAN_POINT('Ctrl Pts',(-202.554802687444,-96.4873005192782,
17.));
#18962=CARTESIAN_POINT('Ctrl Pts',(-202.597597092774,-96.5735930975321,
17.));
#18963=CARTESIAN_POINT('Ctrl Pts',(-202.644686646802,-96.6576840525218,
17.));
#18964=CARTESIAN_POINT('Ctrl Pts',(-202.695725951514,-96.7393268492994,
17.));
#18965=CARTESIAN_POINT('Ctrl Pts',(-202.747782191651,-96.8225963424571,
17.));
#18966=CARTESIAN_POINT('Ctrl Pts',(-202.803947462512,-96.9033199151229,
17.));
#18967=CARTESIAN_POINT('Ctrl Pts',(-202.863910401783,-96.9812287996324,
17.));
#18968=CARTESIAN_POINT('Ctrl Pts',(-202.924370848883,-97.0597840880771,
17.));
#18969=CARTESIAN_POINT('Ctrl Pts',(-202.988692707376,-97.1354786200808,
17.));
#18970=CARTESIAN_POINT('Ctrl Pts',(-203.056606164229,-97.2080175007534,
17.));
#18971=CARTESIAN_POINT('Ctrl Pts',(-203.094651211644,-97.2486537057484,
17.));
#18972=CARTESIAN_POINT('Ctrl Pts',(-203.133824229424,-97.288299178605,17.));
#18973=CARTESIAN_POINT('Ctrl Pts',(-203.174083617339,-97.3268979340229,
17.));
#18974=CARTESIAN_POINT('Ctrl Pts',(-203.185629855,-97.3379679086686,17.));
#18975=CARTESIAN_POINT('Ctrl Pts',(-203.197265472916,-97.3489517664843,
17.));
#18976=CARTESIAN_POINT('Ctrl Pts',(-203.208989546289,-97.3598481307381,
17.));
#18977=CARTESIAN_POINT('Ctrl Pts',(-203.219402554585,-97.3695259899387,
17.));
#18978=CARTESIAN_POINT('Ctrl Pts',(-203.22988211016,-97.3791317753717,17.));
#18979=CARTESIAN_POINT('Ctrl Pts',(-203.240421391601,-97.3886593080805,
17.));
#18980=CARTESIAN_POINT('Ctrl Pts',(-203.316131451988,-97.4571013627712,
17.));
#18981=CARTESIAN_POINT('Ctrl Pts',(-203.395010716132,-97.5215917702376,
17.));
#18982=CARTESIAN_POINT('Ctrl Pts',(-203.47672873235,-97.5818514569894,17.));
#18983=CARTESIAN_POINT('Ctrl Pts',(-203.558539296836,-97.6421793897639,
17.));
#18984=CARTESIAN_POINT('Ctrl Pts',(-203.64319562843,-97.6982678463519,17.));
#18985=CARTESIAN_POINT('Ctrl Pts',(-203.730411362481,-97.7498108582678,
17.));
#18986=CARTESIAN_POINT('Ctrl Pts',(-203.815808401538,-97.8002790524476,
17.));
#18987=CARTESIAN_POINT('Ctrl Pts',(-203.903659887931,-97.8463900605495,
17.));
#18988=CARTESIAN_POINT('Ctrl Pts',(-203.993730815686,-97.8878209215619,
17.));
#18989=CARTESIAN_POINT('Ctrl Pts',(-204.044096679879,-97.9109882317155,
17.));
#18990=CARTESIAN_POINT('Ctrl Pts',(-204.095157077275,-97.9326914441169,
17.));
#18991=CARTESIAN_POINT('Ctrl Pts',(-204.146874513566,-97.9528678786509,
17.));
#18992=CARTESIAN_POINT('Ctrl Pts',(-204.165970747425,-97.9603178595455,
17.));
#18993=CARTESIAN_POINT('Ctrl Pts',(-204.185156583856,-97.9675596309774,
17.));
#18994=CARTESIAN_POINT('Ctrl Pts',(-204.204429055805,-97.9745938792693,
17.));
#18995=CARTESIAN_POINT('Ctrl Pts',(-205.793799282533,-97.9692229537457,
17.));
#18996=CARTESIAN_POINT('Ctrl Pts',(-205.888625424821,-97.9345351273112,
17.));
#18997=CARTESIAN_POINT('Ctrl Pts',(-205.981405808652,-97.8948521769808,
17.));
#18998=CARTESIAN_POINT('Ctrl Pts',(-206.07190060029,-97.8504957325714,17.));
#18999=CARTESIAN_POINT('Ctrl Pts',(-206.163681990447,-97.8055086558944,
17.));
#19000=CARTESIAN_POINT('Ctrl Pts',(-206.253113003673,-97.7557135474638,
17.));
#19001=CARTESIAN_POINT('Ctrl Pts',(-206.339909395556,-97.7014052421032,
17.));
#19002=CARTESIAN_POINT('Ctrl Pts',(-206.36428919546,-97.6861508566487,17.));
#19003=CARTESIAN_POINT('Ctrl Pts',(-206.388460895741,-97.6705401887824,
17.));
#19004=CARTESIAN_POINT('Ctrl Pts',(-206.412417611516,-97.6545793244046,
17.));
#19005=CARTESIAN_POINT('Ctrl Pts',(-206.431857056321,-97.6416280357124,
17.));
#19006=CARTESIAN_POINT('Ctrl Pts',(-206.451157156149,-97.6284444656715,
17.));
#19007=CARTESIAN_POINT('Ctrl Pts',(-206.470294679557,-97.615045820576,17.));
#19008=CARTESIAN_POINT('Ctrl Pts',(-206.55300602175,-97.5571376003872,17.));
#19009=CARTESIAN_POINT('Ctrl Pts',(-206.632761459732,-97.4951644765478,
17.));
#19010=CARTESIAN_POINT('Ctrl Pts',(-206.709295581515,-97.4294253116699,
17.));
#19011=CARTESIAN_POINT('Ctrl Pts',(-206.76882353903,-97.3782936318028,17.));
#19012=CARTESIAN_POINT('Ctrl Pts',(-206.82640208509,-97.324882704478,17.));
#19013=CARTESIAN_POINT('Ctrl Pts',(-206.881888208557,-97.2693210301885,
17.));
#19014=CARTESIAN_POINT('Ctrl Pts',(-206.912065000132,-97.2391031493952,
17.));
#19015=CARTESIAN_POINT('Ctrl Pts',(-206.941622589496,-97.2082489492308,
17.));
#19016=CARTESIAN_POINT('Ctrl Pts',(-206.970535716259,-97.1767781813433,
17.));
#19017=CARTESIAN_POINT('Ctrl Pts',(-206.982341010226,-97.163928596816,17.));
#19018=CARTESIAN_POINT('Ctrl Pts',(-206.994033762366,-97.1509816881149,
17.));
#19019=CARTESIAN_POINT('Ctrl Pts',(-207.0056075954,-97.1379446989878,17.));
#19020=CARTESIAN_POINT('Ctrl Pts',(-207.071007089784,-97.0642774450467,
17.));
#19021=CARTESIAN_POINT('Ctrl Pts',(-207.132664401507,-96.9876805132482,
17.));
#19022=CARTESIAN_POINT('Ctrl Pts',(-207.190334415737,-96.9084322842349,
17.));
#19023=CARTESIAN_POINT('Ctrl Pts',(-207.247546870099,-96.8298128188818,
17.));
#19024=CARTESIAN_POINT('Ctrl Pts',(-207.300835489002,-96.7485831773063,
17.));
#19025=CARTESIAN_POINT('Ctrl Pts',(-207.349914644925,-96.6649933299702,
17.));
#19026=CARTESIAN_POINT('Ctrl Pts',(-207.397475414546,-96.5839895433924,
17.));
#19027=CARTESIAN_POINT('Ctrl Pts',(-207.441083337704,-96.5007686302,17.));
#19028=CARTESIAN_POINT('Ctrl Pts',(-207.480430575245,-96.4155483735031,
17.));
#19029=CARTESIAN_POINT('Ctrl Pts',(-207.501046319853,-96.3708977408989,
17.));
#19030=CARTESIAN_POINT('Ctrl Pts',(-207.520491610764,-96.3256981540745,
17.));
#19031=CARTESIAN_POINT('Ctrl Pts',(-207.538716406462,-96.2799807651805,
17.));
#19032=CARTESIAN_POINT('Ctrl Pts',(-207.545013455281,-96.2641844492984,
17.));
#19033=CARTESIAN_POINT('Ctrl Pts',(-207.551164759148,-96.2483263172452,
17.));
#19034=CARTESIAN_POINT('Ctrl Pts',(-207.557168136471,-96.2324076615222,
17.));
#19035=CARTESIAN_POINT('Ctrl Pts',(-207.562729489382,-96.2176610851248,
17.));
#19036=CARTESIAN_POINT('Ctrl Pts',(-207.568161126813,-96.2028697871422,
17.));
#19037=CARTESIAN_POINT('Ctrl Pts',(-207.573459223174,-96.1880421233524,
17.));
#19038=CARTESIAN_POINT('Ctrl Pts',(-207.604693505319,-96.1006274365002,
17.));
#19039=CARTESIAN_POINT('Ctrl Pts',(-207.631320267415,-96.011871227871,17.));
#19040=CARTESIAN_POINT('Ctrl Pts',(-207.653087285252,-95.9219972305274,
17.));
#19041=CARTESIAN_POINT('Ctrl Pts',(-207.658248202749,-95.9006882809563,
17.));
#19042=CARTESIAN_POINT('Ctrl Pts',(-207.663135701564,-95.8793164527878,
17.));
#19043=CARTESIAN_POINT('Ctrl Pts',(-207.667745988914,-95.8578846668755,
17.));
#19044=CARTESIAN_POINT('Ctrl Pts',(-207.687556304037,-95.7657926994287,
17.));
#19045=CARTESIAN_POINT('Ctrl Pts',(-207.702252299247,-95.6725932801944,
17.));
#19046=CARTESIAN_POINT('Ctrl Pts',(-207.711945419972,-95.5786784812294,
17.));
#19047=CARTESIAN_POINT('Ctrl Pts',(-207.722114123792,-95.4801558483222,
17.));
#19048=CARTESIAN_POINT('Ctrl Pts',(-207.726777009354,-95.3808446338519,
17.));
#19049=CARTESIAN_POINT('Ctrl Pts',(-207.726004467722,-95.2812134714913,
17.));
#19050=CARTESIAN_POINT('Ctrl Pts',(-207.725764520937,-95.2502686315798,
17.));
#19051=CARTESIAN_POINT('Ctrl Pts',(-207.724999819215,-95.2192931170245,
17.));
#19052=CARTESIAN_POINT('Ctrl Pts',(-207.723711405485,-95.1883015738151,
17.));
#19053=CARTESIAN_POINT('Ctrl Pts',(-207.723122799525,-95.1741432280866,
17.));
#19054=CARTESIAN_POINT('Ctrl Pts',(-207.722424806131,-95.1599814556,17.));
#19055=CARTESIAN_POINT('Ctrl Pts',(-207.721618537088,-95.1458321747028,
17.));
#19056=CARTESIAN_POINT('Ctrl Pts',(-207.716327423532,-95.052977993351,17.));
#19057=CARTESIAN_POINT('Ctrl Pts',(-207.706371932179,-94.9605047986718,
17.));
#19058=CARTESIAN_POINT('Ctrl Pts',(-207.69187986909,-94.8687837046641,17.));
#19059=CARTESIAN_POINT('Ctrl Pts',(-207.67741841215,-94.7772563187229,17.));
#19060=CARTESIAN_POINT('Ctrl Pts',(-207.65843910804,-94.686476913951,17.));
#19061=CARTESIAN_POINT('Ctrl Pts',(-207.635020232395,-94.5968312210243,
17.));
#19062=CARTESIAN_POINT('Ctrl Pts',(-207.611996283944,-94.5086972796644,
17.));
#19063=CARTESIAN_POINT('Ctrl Pts',(-207.584680760938,-94.4216583490485,
17.));
#19064=CARTESIAN_POINT('Ctrl Pts',(-207.553107666477,-94.3361100984335,
17.));
#19065=CARTESIAN_POINT('Ctrl Pts',(-207.536805014678,-94.2919375722512,
17.));
#19066=CARTESIAN_POINT('Ctrl Pts',(-207.519366617313,-94.248163031905,17.));
#19067=CARTESIAN_POINT('Ctrl Pts',(-207.500793443899,-94.2048450949011,
17.));
#19068=CARTESIAN_POINT('Ctrl Pts',(-207.494983237603,-94.1912940368956,
17.));
#19069=CARTESIAN_POINT('Ctrl Pts',(-207.489061191608,-94.1777859684221,
17.));
#19070=CARTESIAN_POINT('Ctrl Pts',(-207.483029722208,-94.1643281685061,
17.));
#19071=CARTESIAN_POINT('Ctrl Pts',(-207.446486020386,-94.0827895259774,
17.));
#19072=CARTESIAN_POINT('Ctrl Pts',(-207.406052561607,-94.0033669713649,
17.));
#19073=CARTESIAN_POINT('Ctrl Pts',(-207.361809047075,-93.9264057217905,
17.));
#19074=CARTESIAN_POINT('Ctrl Pts',(-207.318276162464,-93.85068060744,17.));
#19075=CARTESIAN_POINT('Ctrl Pts',(-207.271054166029,-93.7773376777461,
17.));
#19076=CARTESIAN_POINT('Ctrl Pts',(-207.220181837178,-93.7067387347045,
17.));
#19077=CARTESIAN_POINT('Ctrl Pts',(-207.170938074568,-93.6383998622723,
17.));
#19078=CARTESIAN_POINT('Ctrl Pts',(-207.11827349102,-93.5726316597938,17.));
#19079=CARTESIAN_POINT('Ctrl Pts',(-207.062195033272,-93.5098014324231,
17.));
#19080=CARTESIAN_POINT('Ctrl Pts',(-207.027351929298,-93.4707632663797,
17.));
#19081=CARTESIAN_POINT('Ctrl Pts',(-206.991190374561,-93.4328600994283,
17.));
#19082=CARTESIAN_POINT('Ctrl Pts',(-206.953707394001,-93.3961891492629,
17.));
#19083=CARTESIAN_POINT('Ctrl Pts',(-206.941658629391,-93.3844014088023,
17.));
#19084=CARTESIAN_POINT('Ctrl Pts',(-206.929473297568,-93.3727410508926,
17.));
#19085=CARTESIAN_POINT('Ctrl Pts',(-206.91715387718,-93.3612092940949,17.));
#19086=CARTESIAN_POINT('Origin',(-205.,-95.,-2.20842344717744));
#19087=CARTESIAN_POINT('Ctrl Pts',(-201.92372071423,-94.9977231567353,0.291576552822548));
#19088=CARTESIAN_POINT('Ctrl Pts',(-201.922485530331,-94.8497454287996,
0.299259877064297));
#19089=CARTESIAN_POINT('Ctrl Pts',(-201.999542171248,-93.6828631526875,
0.359912640907482));
#19090=CARTESIAN_POINT('Ctrl Pts',(-203.493268957345,-91.692897649157,0.473534844352101));
#19091=CARTESIAN_POINT('Ctrl Pts',(-206.963866039577,-91.9425114466253,
0.632443163156408));
#19092=CARTESIAN_POINT('Ctrl Pts',(-208.633932755097,-94.9948094985304,
0.791351481960715));
#19093=CARTESIAN_POINT('Ctrl Pts',(-206.972489195327,-98.0520533654047,
0.950259800765021));
#19094=CARTESIAN_POINT('Ctrl Pts',(-203.502670888945,-98.3111182651998,
1.10916811956933));
#19095=CARTESIAN_POINT('Ctrl Pts',(-202.001245999945,-96.3232598794757,
1.22294037025517));
#19096=CARTESIAN_POINT('Ctrl Pts',(-201.922516561303,-95.1532539549744,
1.28374318133958));
#19097=CARTESIAN_POINT('Ctrl Pts',(-201.923792845874,-95.0023469955484,
1.29157655282255));
#19098=CARTESIAN_POINT('Ctrl Pts',(-201.929615858992,-95.0031001153078,
0.208423447177458));
#19099=CARTESIAN_POINT('Ctrl Pts',(-201.934957634602,-94.2978296205795,
0.244887843987843));
#19100=CARTESIAN_POINT('Ctrl Pts',(-202.525017678651,-92.5576756090664,
0.334321680399663));
#19101=CARTESIAN_POINT('Ctrl Pts',(-205.417647323366,-91.3907175644162,
0.476724956412918));
#19102=CARTESIAN_POINT('Ctrl Pts',(-208.260129048284,-93.3950151579563,
0.635633275217225));
#19103=CARTESIAN_POINT('Ctrl Pts',(-208.114979996894,-96.8719144846003,
0.794541594021531));
#19104=CARTESIAN_POINT('Ctrl Pts',(-205.113462590801,-98.6320974631547,
0.953449912825839));
#19105=CARTESIAN_POINT('Ctrl Pts',(-202.417551547519,-97.2695714233959,
1.09141053054448));
#19106=CARTESIAN_POINT('Ctrl Pts',(-201.933583924064,-95.6186998810612,
1.17640170866169));
#19107=CARTESIAN_POINT('Ctrl Pts',(-201.930545885435,-94.9983467356882,
1.20842344717746));
#19108=CARTESIAN_POINT('Ctrl Pts',(-206.913465996665,-93.3640127966251,
0.));
#19109=CARTESIAN_POINT('Ctrl Pts',(-207.457950030113,-94.0008464354096,
0.0529694396014356));
#19110=CARTESIAN_POINT('Ctrl Pts',(-207.850593831989,-95.8509324154922,
0.158908318804306));
#19111=CARTESIAN_POINT('Ctrl Pts',(-205.826561617166,-97.8611954663596,
0.317816637608614));
#19112=CARTESIAN_POINT('Ctrl Pts',(-203.043475003269,-97.2425645771078,
0.47672495641292));
#19113=CARTESIAN_POINT('Ctrl Pts',(-202.054677556737,-94.5707911831857,
0.635633275217227));
#19114=CARTESIAN_POINT('Ctrl Pts',(-203.765838490358,-92.2911566070451,
0.794541594021533));
#19115=CARTESIAN_POINT('Ctrl Pts',(-206.608600212993,-92.4956149558742,
0.95344991282584));
#19116=CARTESIAN_POINT('Ctrl Pts',(-207.976549767678,-94.9957484667481,
1.11235823163015));
#19117=CARTESIAN_POINT('Ctrl Pts',(-206.615663429066,-97.4999330884679,
1.27126655043445));
#19118=CARTESIAN_POINT('Ctrl Pts',(-203.773539600754,-97.7121328233741,
1.43017486923876));
#19119=CARTESIAN_POINT('Ctrl Pts',(-202.055828366454,-95.437915374088,1.58908318804307));
#19120=CARTESIAN_POINT('Ctrl Pts',(-203.037297196393,-92.7622046523681,
1.74799150684737));
#19121=CARTESIAN_POINT('Ctrl Pts',(-205.818151752958,-92.1380880866711,
1.90689982565168));
#19122=CARTESIAN_POINT('Ctrl Pts',(-207.848933088516,-94.1377363167912,
2.06580814445599));
#19123=CARTESIAN_POINT('Ctrl Pts',(-207.267844815878,-96.9279002177238,
2.22471646326029));
#19124=CARTESIAN_POINT('Ctrl Pts',(-204.607621567184,-97.9505857971491,
2.3836247820646));
#19125=CARTESIAN_POINT('Ctrl Pts',(-202.307126575009,-96.2682077551517,
2.54253310086891));
#19126=CARTESIAN_POINT('Ctrl Pts',(-202.475427795301,-93.4231507955679,
2.70144141967322));
#19127=CARTESIAN_POINT('Ctrl Pts',(-204.958228618429,-92.0237316699425,
2.86034973847752));
#19128=CARTESIAN_POINT('Ctrl Pts',(-207.479324966578,-93.3529220322061,
3.01925805728183));
#19129=CARTESIAN_POINT('Ctrl Pts',(-207.727403901463,-96.1921350914307,
3.17816637608613));
#19130=CARTESIAN_POINT('Ctrl Pts',(-205.475029420604,-97.9384120109208,
3.33707469489044));
#19131=CARTESIAN_POINT('Ctrl Pts',(-202.787153277457,-96.9907856467029,
3.49598301369475));
#19132=CARTESIAN_POINT('Ctrl Pts',(-202.127990276418,-94.218029249343,3.65489133249906));
#19133=CARTESIAN_POINT('Ctrl Pts',(-204.101853690385,-92.1621748976358,
3.81379965130336));
#19134=CARTESIAN_POINT('Ctrl Pts',(-206.899127602474,-92.7080068813262,
3.97270797010767));
#19135=CARTESIAN_POINT('Ctrl Pts',(-207.955302554838,-95.3551125394054,
4.13161628891197));
#19136=CARTESIAN_POINT('Ctrl Pts',(-206.3020891557,-97.6766549902215,4.29052460771628));
#19137=CARTESIAN_POINT('Ctrl Pts',(-203.455134971813,-97.5442700624972,
4.44943292652059));
#19138=CARTESIAN_POINT('Ctrl Pts',(-202.024495779124,-95.0793267782196,
4.60834124532489));
#19139=CARTESIAN_POINT('Ctrl Pts',(-203.321765599542,-92.5416575903068,
4.7672495641292));
#19140=CARTESIAN_POINT('Ctrl Pts',(-206.15762196102,-92.2577692472075,4.92615788293351));
#19141=CARTESIAN_POINT('Ctrl Pts',(-207.932183447136,-94.4879274089262,
5.08506620173781));
#19142=CARTESIAN_POINT('Ctrl Pts',(-207.018551921327,-97.1875479988099,
5.24397452054212));
#19143=CARTESIAN_POINT('Ctrl Pts',(-204.254334554982,-97.8816490331574,
5.40288283934643));
#19144=CARTESIAN_POINT('Ctrl Pts',(-202.173734934482,-95.9338864415011,
5.56179115815073));
#19145=CARTESIAN_POINT('Ctrl Pts',(-202.684223537468,-93.1299471981326,
5.72069947695505));
#19146=CARTESIAN_POINT('Ctrl Pts',(-205.317790118349,-92.0404514623223,
5.87960779575934));
#19147=CARTESIAN_POINT('Ctrl Pts',(-207.660010270602,-93.6642367475931,
6.03851611456366));
#19148=CARTESIAN_POINT('Ctrl Pts',(-207.563562737152,-96.5126348531206,
6.19742443336797));
#19149=CARTESIAN_POINT('Ctrl Pts',(-205.116869538691,-97.9742662317143,
6.35633275217226));
#19150=CARTESIAN_POINT('Ctrl Pts',(-202.563031653386,-96.709123571831,6.51524107097658));
#19151=CARTESIAN_POINT('Ctrl Pts',(-202.243379110764,-93.8770755238139,
6.67414938978088));
#19152=CARTESIAN_POINT('Ctrl Pts',(-204.450965789212,-92.0745120848694,
6.83305770858519));
#19153=CARTESIAN_POINT('Ctrl Pts',(-207.161900895669,-92.9540032689432,
6.9919660273895));
#19154=CARTESIAN_POINT('Ctrl Pts',(-207.890829424096,-95.7092413883672,
7.1508743461938));
#19155=CARTESIAN_POINT('Ctrl Pts',(-205.969477846714,-97.8142549299807,
7.30978266499811));
#19156=CARTESIAN_POINT('Ctrl Pts',(-203.159319815119,-97.3391910061333,
7.46869098380242));
#19157=CARTESIAN_POINT('Ctrl Pts',(-202.03667680412,-94.7195829125171,7.62759930260672));
#19158=CARTESIAN_POINT('Ctrl Pts',(-203.630775378654,-92.3570580705415,
7.78650762141103));
#19159=CARTESIAN_POINT('Ctrl Pts',(-206.480163782497,-92.4175528498779,
7.94541594021533));
#19160=CARTESIAN_POINT('Ctrl Pts',(-207.972554574031,-94.8456063129684,
8.10432425901964));
#19161=CARTESIAN_POINT('Ctrl Pts',(-206.739740555722,-97.4152061827031,
8.26323257782395));
#19162=CARTESIAN_POINT('Ctrl Pts',(-203.911951840647,-97.7705720183959,
8.42214089662825));
#19163=CARTESIAN_POINT('Ctrl Pts',(-202.081673517178,-95.5859083937338,
8.58104921543256));
#19164=CARTESIAN_POINT('Ctrl Pts',(-202.926884295628,-92.8640905022736,
8.73995753423686));
#19165=CARTESIAN_POINT('Ctrl Pts',(-205.672704381061,-92.1004505657102,
8.89886585304118));
#19166=CARTESIAN_POINT('Ctrl Pts',(-207.801796608615,-93.995085142839,9.05777417184547));
#19167=CARTESIAN_POINT('Ctrl Pts',(-207.362233020492,-96.8110144292876,
9.2166824906498));
#19168=CARTESIAN_POINT('Ctrl Pts',(-204.757000601372,-97.9666259282991,
9.37559080945408));
#19169=CARTESIAN_POINT('Ctrl Pts',(-202.37454731496,-96.4024679336107,9.53449912825841));
#19170=CARTESIAN_POINT('Ctrl Pts',(-202.399079706051,-93.5525430124821,
9.69340744706271));
#19171=CARTESIAN_POINT('Ctrl Pts',(-204.808106752686,-92.0296304795825,
9.85231576586702));
#19172=CARTESIAN_POINT('Ctrl Pts',(-207.393059383707,-93.2299195237957,
10.0112240846713));
#19173=CARTESIAN_POINT('Ctrl Pts',(-207.784081918476,-96.0529985647693,
10.1701324034756));
#19174=CARTESIAN_POINT('Ctrl Pts',(-205.622689267493,-97.9107002907099,
10.3290407222799));
#19175=CARTESIAN_POINT('Ctrl Pts',(-202.890422055742,-97.0999045224228,
10.4879490410842));
#19176=CARTESIAN_POINT('Ctrl Pts',(-202.09219232497,-94.3639397581774,10.6468573598886));
#19177=CARTESIAN_POINT('Ctrl Pts',(-203.9598081707,-92.211107914521,10.8057656786928));
#19178=CARTESIAN_POINT('Ctrl Pts',(-206.781060259523,-92.6151011639616,
10.9646739974972));
#19179=CARTESIAN_POINT('Ctrl Pts',(-207.969456208958,-95.2055430107611,
11.1235823163015));
#19180=CARTESIAN_POINT('Ctrl Pts',(-206.435487895018,-97.6075453226064,
11.2824906351058));
#19181=CARTESIAN_POINT('Ctrl Pts',(-203.585480323077,-97.6189792266813,
11.4413989539101));
#19182=CARTESIAN_POINT('Ctrl Pts',(-202.032288581145,-95.229362247524,11.6003072727144));
#19183=CARTESIAN_POINT('Ctrl Pts',(-203.199861498522,-92.6294685233712,
11.7592155915187));
#19184=CARTESIAN_POINT('Ctrl Pts',(-206.017781274278,-92.2028515620513,
11.918123910323));
#19185=CARTESIAN_POINT('Ctrl Pts',(-207.902610553307,-94.3406290254934,
12.0770322291273));
#19186=CARTESIAN_POINT('Ctrl Pts',(-207.126358918942,-97.0829104287093,
12.2359405479316));
#19187=CARTESIAN_POINT('Ctrl Pts',(-204.400685193564,-97.9156028311452,
12.3948488667359));
#19188=CARTESIAN_POINT('Ctrl Pts',(-202.224456584312,-96.0753031450743,
12.5537571855402));
#19189=CARTESIAN_POINT('Ctrl Pts',(-202.592815156882,-93.2491775540462,
12.7126655043445));
#19190=CARTESIAN_POINT('Ctrl Pts',(-205.168053889028,-92.0281864128756,
12.8715738231488));
#19191=CARTESIAN_POINT('Ctrl Pts',(-207.58922269399,-93.5317207530604,13.0304821419532));
#19192=CARTESIAN_POINT('Ctrl Pts',(-207.636621072365,-96.3813570961325,
13.1893904607574));
#19193=CARTESIAN_POINT('Ctrl Pts',(-205.266794720449,-97.9645806927232,
13.3482987795618));
#19194=CARTESIAN_POINT('Ctrl Pts',(-202.652373950972,-96.829909844503,13.5072070983661));
#19195=CARTESIAN_POINT('Ctrl Pts',(-202.190230503823,-94.0175981038372,
13.6661154171704));
#19196=CARTESIAN_POINT('Ctrl Pts',(-204.30405232757,-92.1059414404975,13.8250237359747));
#19197=CARTESIAN_POINT('Ctrl Pts',(-207.055911196842,-92.8475253202271,
13.983932054779));
#19198=CARTESIAN_POINT('Ctrl Pts',(-207.922933663676,-95.5624739244494,
14.1428403735833));
#19199=CARTESIAN_POINT('Ctrl Pts',(-206.110243207721,-97.761752729989,14.3017486923876));
#19200=CARTESIAN_POINT('Ctrl Pts',(-203.279694206403,-97.4290874824383,
14.4606570111919));
#19201=CARTESIAN_POINT('Ctrl Pts',(-202.026302290869,-94.869462017148,14.6195653299962));
#19202=CARTESIAN_POINT('Ctrl Pts',(-203.499163277813,-92.4295122395567,
14.7784736488005));
#19203=CARTESIAN_POINT('Ctrl Pts',(-206.347974433471,-92.3461570680267,
14.9373819676048));
#19204=CARTESIAN_POINT('Ctrl Pts',(-207.960978032891,-94.6958151102762,
15.0962902864091));
#19205=CARTESIAN_POINT('Ctrl Pts',(-206.859389366482,-97.3243471311393,
15.2551986052135));
#19206=CARTESIAN_POINT('Ctrl Pts',(-204.053134757144,-97.8219422925345,
15.4141069240177));
#19207=CARTESIAN_POINT('Ctrl Pts',(-202.114952629401,-95.7324151709012,
15.5730152428221));
#19208=CARTESIAN_POINT('Ctrl Pts',(-202.821755867583,-92.9714120718513,
15.7319235616264));
#19209=CARTESIAN_POINT('Ctrl Pts',(-205.525536198956,-92.0702079824451,
15.8908318804307));
#19210=CARTESIAN_POINT('Ctrl Pts',(-207.747537243057,-93.8549791002543,
16.049740199235));
#19211=CARTESIAN_POINT('Ctrl Pts',(-207.450572215136,-96.6895450314807,
16.2086485180393));
#19212=CARTESIAN_POINT('Ctrl Pts',(-204.907062930782,-97.9750465199132,
16.3675568368436));
#19213=CARTESIAN_POINT('Ctrl Pts',(-202.44852376407,-96.5332828104831,16.5264651556479));
#19214=CARTESIAN_POINT('Ctrl Pts',(-202.329632350016,-93.68535893981,16.6853734744522));
#19215=CARTESIAN_POINT('Ctrl Pts',(-204.657905597619,-92.0436411981644,
16.8442817932565));
#19216=CARTESIAN_POINT('Ctrl Pts',(-207.301870908767,-93.1102820519823,
17.0031901120608));
#19217=CARTESIAN_POINT('Ctrl Pts',(-207.831183367532,-95.9134396039801,
17.1620984308651));
#19218=CARTESIAN_POINT('Ctrl Pts',(-206.459639356019,-97.2156893163364,
17.268037310068));
#19219=CARTESIAN_POINT('Ctrl Pts',(-205.650199997975,-97.4320868020351,
17.3210067496694));
#19220=CARTESIAN_POINT('Ctrl Pts',(-207.054331550342,-93.2435746787732,
-0.107002249889811));
#19221=CARTESIAN_POINT('Ctrl Pts',(-207.63889941333,-93.9272907410154,-0.0540328102883751));
#19222=CARTESIAN_POINT('Ctrl Pts',(-208.060448869472,-95.9135763642526,
0.051906068914496));
#19223=CARTESIAN_POINT('Ctrl Pts',(-205.887411436318,-98.0718309750383,
0.210814387718803));
#19224=CARTESIAN_POINT('Ctrl Pts',(-202.899439531812,-97.4076577124765,
0.36972270652311));
#19225=CARTESIAN_POINT('Ctrl Pts',(-201.83784878766,-94.5391936853839,0.528631025327416));
#19226=CARTESIAN_POINT('Ctrl Pts',(-203.674981979354,-92.0917369544157,
0.687539344131723));
#19227=CARTESIAN_POINT('Ctrl Pts',(-206.727022155188,-92.311247119458,0.84644766293603));
#19228=CARTESIAN_POINT('Ctrl Pts',(-208.195677430151,-94.9954354773421,
1.00535598174034));
#19229=CARTESIAN_POINT('Ctrl Pts',(-206.734605351153,-97.6839731807802,
1.16426430054464));
#19230=CARTESIAN_POINT('Ctrl Pts',(-203.683250030151,-97.911794637316,1.32317261934895));
#19231=CARTESIAN_POINT('Ctrl Pts',(-201.839084317695,-95.4701538312867,
1.48208093815326));
#19232=CARTESIAN_POINT('Ctrl Pts',(-202.892806927105,-92.5974626181698,
1.64098925695756));
#19233=CARTESIAN_POINT('Ctrl Pts',(-205.878382454666,-91.9273998345941,
1.79989757576187));
#19234=CARTESIAN_POINT('Ctrl Pts',(-208.058665865373,-94.0742581826815,
1.95880589456618));
#19235=CARTESIAN_POINT('Ctrl Pts',(-207.434799032048,-97.0698283899918,
2.11771421337048));
#19236=CARTESIAN_POINT('Ctrl Pts',(-204.57873544886,-98.1678020438509,2.27662253217479));
#19237=CARTESIAN_POINT('Ctrl Pts',(-202.108882599597,-96.361570682906,2.4355308509791));
#19238=CARTESIAN_POINT('Ctrl Pts',(-202.289573820351,-93.3070662993528,
2.5944391697834));
#19239=CARTESIAN_POINT('Ctrl Pts',(-204.955153492556,-91.8046247263461,
2.75334748858771));
#19240=CARTESIAN_POINT('Ctrl Pts',(-207.661847930024,-93.2316674343784,
2.91225580739202));
#19241=CARTESIAN_POINT('Ctrl Pts',(-207.928189941742,-96.2798977012732,
3.07116412619632));
#19242=CARTESIAN_POINT('Ctrl Pts',(-205.51000013995,-98.1547320477393,3.23007244500063));
#19243=CARTESIAN_POINT('Ctrl Pts',(-202.624247911321,-97.1373433189395,
3.38898076380494));
#19244=CARTESIAN_POINT('Ctrl Pts',(-201.916558643673,-94.1604621209265,
3.54788908260924));
#19245=CARTESIAN_POINT('Ctrl Pts',(-204.035733948823,-91.9532598685839,
3.70679740141355));
#19246=CARTESIAN_POINT('Ctrl Pts',(-207.038937592143,-92.5392749152246,
3.86570572021786));
#19247=CARTESIAN_POINT('Ctrl Pts',(-208.172866039841,-95.3812552169174,
4.02461403902216));
#19248=CARTESIAN_POINT('Ctrl Pts',(-206.397946364646,-97.8737049967838,
4.18352235782647));
#19249=CARTESIAN_POINT('Ctrl Pts',(-203.341405086918,-97.7315741544865,
4.34243067663077));
#19250=CARTESIAN_POINT('Ctrl Pts',(-201.805445087723,-95.0851666575561,
4.50133899543508));
#19251=CARTESIAN_POINT('Ctrl Pts',(-203.198217327227,-92.3606793208876,
4.66024731423939));
#19252=CARTESIAN_POINT('Ctrl Pts',(-206.242843782976,-92.0558916836784,
4.8191556330437));
#19253=CARTESIAN_POINT('Ctrl Pts',(-208.148044949501,-94.4502296451874,
4.978063951848));
#19254=CARTESIAN_POINT('Ctrl Pts',(-207.16715369137,-97.3485909233169,5.13697227065231));
#19255=CARTESIAN_POINT('Ctrl Pts',(-204.199440150821,-98.0937902926655,
5.29588058945661));
#19256=CARTESIAN_POINT('Ctrl Pts',(-201.965670932306,-96.0026373003525,
5.45478890826093));
#19257=CARTESIAN_POINT('Ctrl Pts',(-202.513740688985,-92.9922776373462,
5.61369722706523));
#19258=CARTESIAN_POINT('Ctrl Pts',(-205.341185193596,-91.8225753965231,
5.77260554586954));
#19259=CARTESIAN_POINT('Ctrl Pts',(-207.855834926075,-93.5659005187498,
5.93151386467385));
#19260=CARTESIAN_POINT('Ctrl Pts',(-207.752287117404,-96.6239920167532,
6.09042218347815));
#19261=CARTESIAN_POINT('Ctrl Pts',(-205.125473241242,-98.1932257848202,
6.24933050228246));
#19262=CARTESIAN_POINT('Ctrl Pts',(-202.383626899898,-96.8349458433886,
6.40823882108676));
#19263=CARTESIAN_POINT('Ctrl Pts',(-202.040442174065,-93.7944080615484,
6.56714713989107));
#19264=CARTESIAN_POINT('Ctrl Pts',(-204.410546984685,-91.8591434942289,
6.72605545869538));
#19265=CARTESIAN_POINT('Ctrl Pts',(-207.32105573155,-92.8033810666965,6.88496377749969));
#19266=CARTESIAN_POINT('Ctrl Pts',(-208.103646525691,-95.7614543260611,
7.04387209630399));
#19267=CARTESIAN_POINT('Ctrl Pts',(-206.040848873893,-98.0214347699103,
7.20278041510829));
#19268=CARTESIAN_POINT('Ctrl Pts',(-203.023812607864,-97.5113975866576,
7.36168873391261));
#19269=CARTESIAN_POINT('Ctrl Pts',(-201.818522855506,-94.6989391653287,
7.52059705271691));
#19270=CARTESIAN_POINT('Ctrl Pts',(-203.529975790509,-92.1624899523317,
7.67950537152122));
#19271=CARTESIAN_POINT('Ctrl Pts',(-206.589130490616,-92.2274382367739,
7.83841369032553));
#19272=CARTESIAN_POINT('Ctrl Pts',(-208.19138811831,-94.8342401573922,7.99732200912983));
#19273=CARTESIAN_POINT('Ctrl Pts',(-206.867816788622,-97.5930088490497,
8.15623032793414));
#19274=CARTESIAN_POINT('Ctrl Pts',(-203.831851903328,-97.9745360094224,
8.31513864673845));
#19275=CARTESIAN_POINT('Ctrl Pts',(-201.866832136913,-95.6290418021305,
8.47404696554275));
#19276=CARTESIAN_POINT('Ctrl Pts',(-202.774265648607,-92.7068491013155,
8.63295528434706));
#19277=CARTESIAN_POINT('Ctrl Pts',(-205.722227537085,-91.8869915143411,
8.79186360315137));
#19278=CARTESIAN_POINT('Ctrl Pts',(-208.008059291752,-93.9211053135663,
8.95077192195567));
#19279=CARTESIAN_POINT('Ctrl Pts',(-207.536135908197,-96.9443377027313,
9.10968024075998));
#19280=CARTESIAN_POINT('Ctrl Pts',(-204.739111469874,-98.1850230174926,
9.26858855956428));
#19281=CARTESIAN_POINT('Ctrl Pts',(-202.181266720073,-96.5057148281605,
9.4274968783686));
#19282=CARTESIAN_POINT('Ctrl Pts',(-202.20760513691,-93.4459841134342,9.58640519717289));
#19283=CARTESIAN_POINT('Ctrl Pts',(-204.793979954208,-91.8109577945972,
9.74531351597721));
#19284=CARTESIAN_POINT('Ctrl Pts',(-207.569231646844,-93.099609726408,9.90422183478151));
#19285=CARTESIAN_POINT('Ctrl Pts',(-207.989040481425,-96.1305182207789,
10.0631301535858));
#19286=CARTESIAN_POINT('Ctrl Pts',(-205.668530410522,-98.1249802459081,
10.2220384723901));
#19287=CARTESIAN_POINT('Ctrl Pts',(-202.735119131279,-97.2544953088468,
10.3809467911944));
#19288=CARTESIAN_POINT('Ctrl Pts',(-201.878125318374,-94.3171142706628,
10.5398551099987));
#19289=CARTESIAN_POINT('Ctrl Pts',(-203.883231321036,-92.0057952366625,
10.698763428803));
#19290=CARTESIAN_POINT('Ctrl Pts',(-206.912178366679,-92.4395296640824,
10.8576717476074));
#19291=CARTESIAN_POINT('Ctrl Pts',(-208.188061657773,-95.2206746776241,
11.0165800664117));
#19292=CARTESIAN_POINT('Ctrl Pts',(-206.541165653327,-97.7995076131551,
11.175488385216));
#19293=CARTESIAN_POINT('Ctrl Pts',(-203.481346203201,-97.8117832584635,
11.3343967040203));
#19294=CARTESIAN_POINT('Ctrl Pts',(-201.8138115803,-95.2462474391325,11.4933050228246));
#19295=CARTESIAN_POINT('Ctrl Pts',(-203.067338889211,-92.4549547198617,
11.6522133416289));
#19296=CARTESIAN_POINT('Ctrl Pts',(-206.09270830354,-91.9969310679766,11.8111216604332));
#19297=CARTESIAN_POINT('Ctrl Pts',(-208.116294958158,-94.2920874482903,
11.9700299792375));
#19298=CARTESIAN_POINT('Ctrl Pts',(-207.282897225321,-97.2362501438185,
12.1289382980418));
#19299=CARTESIAN_POINT('Ctrl Pts',(-204.356564831779,-98.1302437016009,
12.2878466168461));
#19300=CARTESIAN_POINT('Ctrl Pts',(-202.020126608923,-96.1544648198391,
12.4467549356504));
#19301=CARTESIAN_POINT('Ctrl Pts',(-202.415603005571,-93.1202854944699,
12.6056632544547));
#19302=CARTESIAN_POINT('Ctrl Pts',(-205.180425681454,-91.8094074185768,
12.764571573259));
#19303=CARTESIAN_POINT('Ctrl Pts',(-207.779836109132,-93.4236289607667,
12.9234798920633));
#19304=CARTESIAN_POINT('Ctrl Pts',(-207.83072386167,-96.4830498528951,13.0823882108676));
#19305=CARTESIAN_POINT('Ctrl Pts',(-205.286435616122,-98.1828272157492,
13.241296529672));
#19306=CARTESIAN_POINT('Ctrl Pts',(-202.479546399398,-96.9646241607618,
13.4002048484762));
#19307=CARTESIAN_POINT('Ctrl Pts',(-201.983380872592,-93.9452756338911,
13.5591131672806));
#19308=CARTESIAN_POINT('Ctrl Pts',(-204.252818046752,-91.8928866163885,
13.7180214860849));
#19309=CARTESIAN_POINT('Ctrl Pts',(-207.207263282303,-92.6890644235765,
13.8769298048892));
#19310=CARTESIAN_POINT('Ctrl Pts',(-208.138114215414,-95.6038821339156,
14.0358381236935));
#19311=CARTESIAN_POINT('Ctrl Pts',(-206.191977100272,-97.9650674625775,
14.1947464424978));
#19312=CARTESIAN_POINT('Ctrl Pts',(-203.153048721962,-97.6079120624099,
14.3536547613021));
#19313=CARTESIAN_POINT('Ctrl Pts',(-201.807384591263,-94.8598520709758,
14.5125630801064));
#19314=CARTESIAN_POINT('Ctrl Pts',(-203.388674669069,-92.2402780528891,
14.6714713989107));
#19315=CARTESIAN_POINT('Ctrl Pts',(-206.447209625131,-92.1507864397344,
14.830379717715));
#19316=CARTESIAN_POINT('Ctrl Pts',(-208.17895933528,-94.6734216248493,14.9892880365193));
#19317=CARTESIAN_POINT('Ctrl Pts',(-206.996273906404,-97.4954609351664,
15.1481963553236));
#19318=CARTESIAN_POINT('Ctrl Pts',(-203.9834284248,-98.0296880607766,15.3071046741279));
#19319=CARTESIAN_POINT('Ctrl Pts',(-201.902561191062,-95.7863341162865,
15.4660129929323));
#19320=CARTESIAN_POINT('Ctrl Pts',(-202.66139787518,-92.8220714709839,15.6249213117365));
#19321=CARTESIAN_POINT('Ctrl Pts',(-205.564225126678,-91.8545225323609,
15.7838296305409));
#19322=CARTESIAN_POINT('Ctrl Pts',(-207.949805459824,-93.7706849433184,
15.9427379493452));
#19323=CARTESIAN_POINT('Ctrl Pts',(-207.630978458316,-96.813925969912,16.1016462681495));
#19324=CARTESIAN_POINT('Ctrl Pts',(-204.900221088943,-98.1940635162815,
16.2605545869538));
#19325=CARTESIAN_POINT('Ctrl Pts',(-202.260689167953,-96.6461600355912,
16.4194629057581));
#19326=CARTESIAN_POINT('Ctrl Pts',(-202.133045204913,-93.5885776846673,
16.5783712245624));
#19327=CARTESIAN_POINT('Ctrl Pts',(-204.632721289413,-91.8259999543616,
16.7372795433667));
#19328=CARTESIAN_POINT('Ctrl Pts',(-207.471330058092,-92.9711647823235,
16.896187862171));
#19329=CARTESIAN_POINT('Ctrl Pts',(-208.039609445301,-95.9806852073979,
17.0550961809753));
#19330=CARTESIAN_POINT('Ctrl Pts',(-206.56709509676,-97.3788039485619,17.1610350601782));
#19331=CARTESIAN_POINT('Ctrl Pts',(-205.698066426161,-97.6111321859386,
17.2140044997796));
#19332=CARTESIAN_POINT('Ctrl Pts',(-207.195197104019,-93.1231365609213,
-0.214004499779621));
#19333=CARTESIAN_POINT('Ctrl Pts',(-207.819848796546,-93.8537350466211,
-0.161035060178185));
#19334=CARTESIAN_POINT('Ctrl Pts',(-208.270303906954,-95.9762203130131,
-0.0550961809753145));
#19335=CARTESIAN_POINT('Ctrl Pts',(-205.948261255469,-98.2824664837171,
0.103812137828992));
#19336=CARTESIAN_POINT('Ctrl Pts',(-202.755404060354,-97.5727508478452,
0.262720456633299));
#19337=CARTESIAN_POINT('Ctrl Pts',(-201.621020018583,-94.5075961875819,
0.421628775437606));
#19338=CARTESIAN_POINT('Ctrl Pts',(-203.584125468349,-91.8923173017865,
0.580537094241912));
#19339=CARTESIAN_POINT('Ctrl Pts',(-206.845444097382,-92.1268792830416,
0.739445413046219));
#19340=CARTESIAN_POINT('Ctrl Pts',(-208.414805092624,-94.9951224879363,
0.898353731850525));
#19341=CARTESIAN_POINT('Ctrl Pts',(-206.85354727324,-97.8680132730923,1.05726205065483));
#19342=CARTESIAN_POINT('Ctrl Pts',(-203.592960459548,-98.111456451258,1.21617036945914));
#19343=CARTESIAN_POINT('Ctrl Pts',(-201.622340268936,-95.5023922884853,
1.37507868826345));
#19344=CARTESIAN_POINT('Ctrl Pts',(-202.748316657816,-92.4327205839714,
1.53398700706775));
#19345=CARTESIAN_POINT('Ctrl Pts',(-205.938613156373,-91.7167115825171,
1.69289532587206));
#19346=CARTESIAN_POINT('Ctrl Pts',(-208.26839864223,-94.0107800485717,1.85180364467637));
#19347=CARTESIAN_POINT('Ctrl Pts',(-207.601753248218,-97.2117565622599,
2.01071196348067));
#19348=CARTESIAN_POINT('Ctrl Pts',(-204.549849330536,-98.3850182905525,
2.16962028228498));
#19349=CARTESIAN_POINT('Ctrl Pts',(-201.910638624185,-96.4549336106603,
2.32852860108929));
#19350=CARTESIAN_POINT('Ctrl Pts',(-202.103719845401,-93.1909818031377,
2.48743691989359));
#19351=CARTESIAN_POINT('Ctrl Pts',(-204.952078366683,-91.5855177827496,
2.6463452386979));
#19352=CARTESIAN_POINT('Ctrl Pts',(-207.844370893469,-93.1104128365508,
2.80525355750221));
#19353=CARTESIAN_POINT('Ctrl Pts',(-208.128975982022,-96.3676603111157,
2.96416187630651));
#19354=CARTESIAN_POINT('Ctrl Pts',(-205.544970859296,-98.3710520845579,
3.12307019511082));
#19355=CARTESIAN_POINT('Ctrl Pts',(-202.461342545186,-97.283900991176,3.28197851391513));
#19356=CARTESIAN_POINT('Ctrl Pts',(-201.705127010927,-94.1028949925101,
3.44088683271943));
#19357=CARTESIAN_POINT('Ctrl Pts',(-203.969614207261,-91.744344839532,3.59979515152374));
#19358=CARTESIAN_POINT('Ctrl Pts',(-207.178747581812,-92.370542949123,3.75870347032805));
#19359=CARTESIAN_POINT('Ctrl Pts',(-208.390429524845,-95.4073978944294,
3.91761178913235));
#19360=CARTESIAN_POINT('Ctrl Pts',(-206.493803573593,-98.0707550033463,
4.07652010793666));
#19361=CARTESIAN_POINT('Ctrl Pts',(-203.227675202022,-97.9188782464756,
4.23542842674096));
#19362=CARTESIAN_POINT('Ctrl Pts',(-201.586394396321,-95.0910065368929,
4.39433674554527));
#19363=CARTESIAN_POINT('Ctrl Pts',(-203.074669054913,-92.1797010514681,
4.55324506434958));
#19364=CARTESIAN_POINT('Ctrl Pts',(-206.328065604933,-91.8540141201495,
4.71215338315389));
#19365=CARTESIAN_POINT('Ctrl Pts',(-208.363906451865,-94.4125318814486,
4.87106170195819));
#19366=CARTESIAN_POINT('Ctrl Pts',(-207.315755461415,-97.5096338478239,
5.0299700207625));
#19367=CARTESIAN_POINT('Ctrl Pts',(-204.144545746659,-98.3059315521737,
5.1888783395668));
#19368=CARTESIAN_POINT('Ctrl Pts',(-201.757606930131,-96.0713881592039,
5.34778665837112));
#19369=CARTESIAN_POINT('Ctrl Pts',(-202.343257840502,-92.8546080765599,
5.50669497717542));
#19370=CARTESIAN_POINT('Ctrl Pts',(-205.364580268843,-91.6046993307239,
5.66560329597973));
#19371=CARTESIAN_POINT('Ctrl Pts',(-208.051659581547,-93.4675642899066,
5.82451161478403));
#19372=CARTESIAN_POINT('Ctrl Pts',(-207.941011497657,-96.7353491803859,
5.98341993358834));
#19373=CARTESIAN_POINT('Ctrl Pts',(-205.134076943793,-98.4121853379263,
6.14232825239264));
#19374=CARTESIAN_POINT('Ctrl Pts',(-202.204222146409,-96.9607681149461,
6.30123657119695));
#19375=CARTESIAN_POINT('Ctrl Pts',(-201.837505237367,-93.711740599283,6.46014489000126));
#19376=CARTESIAN_POINT('Ctrl Pts',(-204.370128180156,-91.6437749035884,
6.61905320880557));
#19377=CARTESIAN_POINT('Ctrl Pts',(-207.480210567431,-92.6527588644499,
6.77796152760988));
#19378=CARTESIAN_POINT('Ctrl Pts',(-208.316463627286,-95.8136672637549,
6.93686984641418));
#19379=CARTESIAN_POINT('Ctrl Pts',(-206.112219901073,-98.22861460984,7.09577816521849));
#19380=CARTESIAN_POINT('Ctrl Pts',(-202.888305400608,-97.683604167182,7.25468648402279));
#19381=CARTESIAN_POINT('Ctrl Pts',(-201.600368906892,-94.6782954181403,
7.4135948028271));
#19382=CARTESIAN_POINT('Ctrl Pts',(-203.429176202363,-91.967921834122,7.57250312163141));
#19383=CARTESIAN_POINT('Ctrl Pts',(-206.698097198735,-92.0373236236699,
7.73141144043571));
#19384=CARTESIAN_POINT('Ctrl Pts',(-208.410221662588,-94.8228740018159,
7.89031975924003));
#19385=CARTESIAN_POINT('Ctrl Pts',(-206.995893021523,-97.7708115153964,
8.04922807804432));
#19386=CARTESIAN_POINT('Ctrl Pts',(-203.751751966009,-98.178500000449,8.20813639684863));
#19387=CARTESIAN_POINT('Ctrl Pts',(-201.651990756648,-95.6721752105271,
8.36704471565293));
#19388=CARTESIAN_POINT('Ctrl Pts',(-202.621647001585,-92.5496077003575,
8.52595303445725));
#19389=CARTESIAN_POINT('Ctrl Pts',(-205.771750693109,-91.6735324629718,
8.68486135326155));
#19390=CARTESIAN_POINT('Ctrl Pts',(-208.214321974889,-93.8471254842938,
8.84376967206586));
#19391=CARTESIAN_POINT('Ctrl Pts',(-207.710038795902,-97.077660976175,9.00267799087017));
#19392=CARTESIAN_POINT('Ctrl Pts',(-204.721222338376,-98.4034201066862,
9.16158630967447));
#19393=CARTESIAN_POINT('Ctrl Pts',(-201.987986125186,-96.6089617227103,
9.32049462847878));
#19394=CARTESIAN_POINT('Ctrl Pts',(-202.016130567769,-93.3394252143862,
9.47940294728308));
#19395=CARTESIAN_POINT('Ctrl Pts',(-204.77985315573,-91.5922851096117,9.6383112660874));
#19396=CARTESIAN_POINT('Ctrl Pts',(-207.745403909981,-92.9692999290205,
9.7972195848917));
#19397=CARTESIAN_POINT('Ctrl Pts',(-208.193999044374,-96.2080378767884,
9.956127903696));
#19398=CARTESIAN_POINT('Ctrl Pts',(-205.714371553552,-98.3392602011063,
10.1150362225003));
#19399=CARTESIAN_POINT('Ctrl Pts',(-202.579816206816,-97.4090860952708,
10.2739445413046));
#19400=CARTESIAN_POINT('Ctrl Pts',(-201.664058311778,-94.2702887831483,
10.4328528601089));
#19401=CARTESIAN_POINT('Ctrl Pts',(-203.806654471371,-91.8004825588039,
10.5917611789132));
#19402=CARTESIAN_POINT('Ctrl Pts',(-207.043296473835,-92.2639581642033,
10.7506694977175));
#19403=CARTESIAN_POINT('Ctrl Pts',(-208.406667106589,-95.235806344487,10.9095778165218));
#19404=CARTESIAN_POINT('Ctrl Pts',(-206.646843411636,-97.991469903704,11.0684861353262));
#19405=CARTESIAN_POINT('Ctrl Pts',(-203.377212083324,-98.0045872902456,
11.2273944541305));
#19406=CARTESIAN_POINT('Ctrl Pts',(-201.595334579455,-95.2631326307411,
11.3863027729348));
#19407=CARTESIAN_POINT('Ctrl Pts',(-202.9348162799,-92.2804409163521,11.5452110917391));
#19408=CARTESIAN_POINT('Ctrl Pts',(-206.167635332802,-91.7910105739019,
11.7041194105434));
#19409=CARTESIAN_POINT('Ctrl Pts',(-208.329979363009,-94.2435458710873,
11.8630277293477));
#19410=CARTESIAN_POINT('Ctrl Pts',(-207.439435531701,-97.3895898589279,
12.021936048152));
#19411=CARTESIAN_POINT('Ctrl Pts',(-204.312444469995,-98.3448845720566,
12.1808443669563));
#19412=CARTESIAN_POINT('Ctrl Pts',(-201.815796633535,-96.233626494604,12.3397526857606));
#19413=CARTESIAN_POINT('Ctrl Pts',(-202.23839085426,-92.9913934348935,12.4986610045649));
#19414=CARTESIAN_POINT('Ctrl Pts',(-205.192797473881,-91.5906284242781,
12.6575693233692));
#19415=CARTESIAN_POINT('Ctrl Pts',(-207.970449524274,-93.3155371684729,
12.8164776421735));
#19416=CARTESIAN_POINT('Ctrl Pts',(-208.024826650977,-96.5847426096578,
12.9753859609778));
#19417=CARTESIAN_POINT('Ctrl Pts',(-205.306076511795,-98.4010737387753,
13.1342942797821));
#19418=CARTESIAN_POINT('Ctrl Pts',(-202.306718847825,-97.0993384770204,
13.2932025985864));
#19419=CARTESIAN_POINT('Ctrl Pts',(-201.77653124136,-93.8729531639453,13.4521109173908));
#19420=CARTESIAN_POINT('Ctrl Pts',(-204.201583765935,-91.6798317922794,
13.6110192361951));
#19421=CARTESIAN_POINT('Ctrl Pts',(-207.358615367764,-92.5306035269258,
13.7699275549994));
#19422=CARTESIAN_POINT('Ctrl Pts',(-208.353294767152,-95.6452903433819,
13.9288358738037));
#19423=CARTESIAN_POINT('Ctrl Pts',(-206.273710992823,-98.1683821951658,
14.087744192608));
#19424=CARTESIAN_POINT('Ctrl Pts',(-203.026403237521,-97.7867366423815,
14.2466525114123));
#19425=CARTESIAN_POINT('Ctrl Pts',(-201.588466891657,-94.8502421248036,
14.4055608302166));
#19426=CARTESIAN_POINT('Ctrl Pts',(-203.278186060326,-92.0510438662215,
14.5644691490209));
#19427=CARTESIAN_POINT('Ctrl Pts',(-206.546444816791,-91.9554158114422,
14.7233774678252));
#19428=CARTESIAN_POINT('Ctrl Pts',(-208.396940637668,-94.6510281394225,
14.8822857866295));
#19429=CARTESIAN_POINT('Ctrl Pts',(-207.133158446327,-97.6665747391933,
15.0411941054338));
#19430=CARTESIAN_POINT('Ctrl Pts',(-203.913722092456,-98.2374338290189,
15.2001024242381));
#19431=CARTESIAN_POINT('Ctrl Pts',(-201.690169752724,-95.8402530616716,
15.3590107430424));
#19432=CARTESIAN_POINT('Ctrl Pts',(-202.501039882777,-92.6727308701165,
15.5179190618467));
#19433=CARTESIAN_POINT('Ctrl Pts',(-205.6029140544,-91.6388370822767,15.6768273806511));
#19434=CARTESIAN_POINT('Ctrl Pts',(-208.152073676592,-93.6863907863824,
15.8357356994554));
#19435=CARTESIAN_POINT('Ctrl Pts',(-207.811384701495,-96.9383069083435,
15.9946440182597));
#19436=CARTESIAN_POINT('Ctrl Pts',(-204.893379247105,-98.4130805126498,
16.153552337064));
#19437=CARTESIAN_POINT('Ctrl Pts',(-202.072854571835,-96.7590372606993,
16.3124606558683));
#19438=CARTESIAN_POINT('Ctrl Pts',(-201.93645805981,-93.4917964295245,16.4713689746726));
#19439=CARTESIAN_POINT('Ctrl Pts',(-204.607536981208,-91.6083587105588,
16.6302772934769));
#19440=CARTESIAN_POINT('Ctrl Pts',(-207.640789207417,-92.8320475126647,
16.7891856122812));
#19441=CARTESIAN_POINT('Ctrl Pts',(-208.24803552307,-96.0479308108158,16.9480939310855));
#19442=CARTESIAN_POINT('Ctrl Pts',(-206.674550837501,-97.5419185807874,
17.0540328102884));
#19443=CARTESIAN_POINT('Ctrl Pts',(-205.745932854347,-97.7901775698422,
17.1070022498898));
#19444=CARTESIAN_POINT('Ctrl Pts',(-207.336062657696,-93.0026984430694,
-0.321006749669432));
#19445=CARTESIAN_POINT('Ctrl Pts',(-208.000798179763,-93.7801793522269,
-0.268037310067996));
#19446=CARTESIAN_POINT('Ctrl Pts',(-208.480158944437,-96.0388642617737,
-0.162098430865125));
#19447=CARTESIAN_POINT('Ctrl Pts',(-206.009111074621,-98.4931019923957,
-0.00319011206081841));
#19448=CARTESIAN_POINT('Ctrl Pts',(-202.611368588897,-97.7378439832139,
0.155718206743489));
#19449=CARTESIAN_POINT('Ctrl Pts',(-201.404191249506,-94.47599868978,0.314626525547795));
#19450=CARTESIAN_POINT('Ctrl Pts',(-203.493268957345,-91.692897649157,0.473534844352101));
#19451=CARTESIAN_POINT('Ctrl Pts',(-206.963866039577,-91.9425114466253,
0.632443163156408));
#19452=CARTESIAN_POINT('Ctrl Pts',(-208.633932755097,-94.9948094985304,
0.791351481960715));
#19453=CARTESIAN_POINT('Ctrl Pts',(-206.972489195327,-98.0520533654047,
0.950259800765021));
#19454=CARTESIAN_POINT('Ctrl Pts',(-203.502670888945,-98.3111182651998,
1.10916811956933));
#19455=CARTESIAN_POINT('Ctrl Pts',(-201.405596220178,-95.534630745684,1.26807643837364));
#19456=CARTESIAN_POINT('Ctrl Pts',(-202.603826388527,-92.2679785497729,
1.42698475717794));
#19457=CARTESIAN_POINT('Ctrl Pts',(-205.99884385808,-91.5060233304403,1.58589307598225));
#19458=CARTESIAN_POINT('Ctrl Pts',(-208.478131419088,-93.947301914462,1.74480139478656));
#19459=CARTESIAN_POINT('Ctrl Pts',(-207.768707464389,-97.3536847345279,
1.90370971359086));
#19460=CARTESIAN_POINT('Ctrl Pts',(-204.520963212211,-98.6022345372543,
2.06261803239517));
#19461=CARTESIAN_POINT('Ctrl Pts',(-201.712394648774,-96.5482965384147,
2.22152635119948));
#19462=CARTESIAN_POINT('Ctrl Pts',(-201.91786587045,-93.0748973069226,2.38043467000378));
#19463=CARTESIAN_POINT('Ctrl Pts',(-204.94900324081,-91.3664108391532,2.53934298880809));
#19464=CARTESIAN_POINT('Ctrl Pts',(-208.026893856913,-92.9891582387231,
2.6982513076124));
#19465=CARTESIAN_POINT('Ctrl Pts',(-208.329762022302,-96.4554229209582,
2.8571596264167));
#19466=CARTESIAN_POINT('Ctrl Pts',(-205.579941578641,-98.5873721213763,
3.01606794522101));
#19467=CARTESIAN_POINT('Ctrl Pts',(-202.298437179052,-97.4304586634127,
3.17497626402532));
#19468=CARTESIAN_POINT('Ctrl Pts',(-201.493695378181,-94.0453278640936,
3.33388458282962));
#19469=CARTESIAN_POINT('Ctrl Pts',(-203.9034944657,-91.5354298104801,3.49279290163393));
#19470=CARTESIAN_POINT('Ctrl Pts',(-207.318557571481,-92.2018109830213,
3.65170122043824));
#19471=CARTESIAN_POINT('Ctrl Pts',(-208.607993009848,-95.4335405719414,
3.81060953924254));
#19472=CARTESIAN_POINT('Ctrl Pts',(-206.589660782539,-98.2678050099089,
3.96951785804685));
#19473=CARTESIAN_POINT('Ctrl Pts',(-203.113945317127,-98.1061823384649,
4.12842617685115));
#19474=CARTESIAN_POINT('Ctrl Pts',(-201.36734370492,-95.0968464162294,4.28733449565546));
#19475=CARTESIAN_POINT('Ctrl Pts',(-202.951120782599,-91.9987227820489,
4.44624281445977));
#19476=CARTESIAN_POINT('Ctrl Pts',(-206.413287426889,-91.6521365566204,
4.60515113326408));
#19477=CARTESIAN_POINT('Ctrl Pts',(-208.57976795423,-94.3748341177099,4.76405945206838));
#19478=CARTESIAN_POINT('Ctrl Pts',(-207.464357231459,-97.6706767723307,
4.92296777087269));
#19479=CARTESIAN_POINT('Ctrl Pts',(-204.089651342497,-98.5180728116819,
5.081876089677));
#19480=CARTESIAN_POINT('Ctrl Pts',(-201.549542927956,-96.1401390180551,
5.2407844084813));
#19481=CARTESIAN_POINT('Ctrl Pts',(-202.172774992019,-92.7169385157737,
5.39969272728561));
#19482=CARTESIAN_POINT('Ctrl Pts',(-205.38797534409,-91.3868232649246,5.55860104608991));
#19483=CARTESIAN_POINT('Ctrl Pts',(-208.247484237019,-93.3692280610634,
5.71750936489423));
#19484=CARTESIAN_POINT('Ctrl Pts',(-208.129735877909,-96.8467063440184,
5.87641768369853));
#19485=CARTESIAN_POINT('Ctrl Pts',(-205.142680646343,-98.6311448910324,
6.03532600250284));
#19486=CARTESIAN_POINT('Ctrl Pts',(-202.024817392921,-97.0865903865035,
6.19423432130714));
#19487=CARTESIAN_POINT('Ctrl Pts',(-201.634568300669,-93.6290731370177,
6.35314264011145));
#19488=CARTESIAN_POINT('Ctrl Pts',(-204.329709375628,-91.4284063129477,
6.51205095891576));
#19489=CARTESIAN_POINT('Ctrl Pts',(-207.639365403312,-92.5021366622034,
6.67095927772007));
#19490=CARTESIAN_POINT('Ctrl Pts',(-208.529280728881,-95.8658802014486,
6.82986759652437));
#19491=CARTESIAN_POINT('Ctrl Pts',(-206.183590928253,-98.4357944497699,
6.98877591532868));
#19492=CARTESIAN_POINT('Ctrl Pts',(-202.752798193353,-97.8558107477063,
7.14768423413298));
#19493=CARTESIAN_POINT('Ctrl Pts',(-201.382214958278,-94.6576516709519,
7.30659255293729));
#19494=CARTESIAN_POINT('Ctrl Pts',(-203.328376614218,-91.7733537159122,
7.46550087174159));
#19495=CARTESIAN_POINT('Ctrl Pts',(-206.807063906854,-91.847209010566,7.62440919054591));
#19496=CARTESIAN_POINT('Ctrl Pts',(-208.629055206866,-94.8115078462396,
7.7833175093502));
#19497=CARTESIAN_POINT('Ctrl Pts',(-207.123969254423,-97.9486141817431,
7.94222582815452));
#19498=CARTESIAN_POINT('Ctrl Pts',(-203.67165202869,-98.3824639914755,8.10113414695881));
#19499=CARTESIAN_POINT('Ctrl Pts',(-201.437149376383,-95.715308618924,8.26004246576313));
#19500=CARTESIAN_POINT('Ctrl Pts',(-202.469028354564,-92.3923662993994,
8.41895078456744));
#19501=CARTESIAN_POINT('Ctrl Pts',(-205.821273849133,-91.4600734116028,
8.57785910337174));
#19502=CARTESIAN_POINT('Ctrl Pts',(-208.420584658025,-93.7731456550212,
8.73676742217605));
#19503=CARTESIAN_POINT('Ctrl Pts',(-207.883941683608,-97.2109842496187,
8.89567574098036));
#19504=CARTESIAN_POINT('Ctrl Pts',(-204.703333206878,-98.6218171958797,
9.05458405978466));
#19505=CARTESIAN_POINT('Ctrl Pts',(-201.7947055303,-96.7122086172601,9.21349237858897));
#19506=CARTESIAN_POINT('Ctrl Pts',(-201.824655998628,-93.2328663153382,
9.37240069739327));
#19507=CARTESIAN_POINT('Ctrl Pts',(-204.765726357252,-91.3736124246263,
9.53130901619759));
#19508=CARTESIAN_POINT('Ctrl Pts',(-207.921576173118,-92.8389901316329,
9.69021733500189));
#19509=CARTESIAN_POINT('Ctrl Pts',(-208.398957607323,-96.2855575327979,
9.84912565380619));
#19510=CARTESIAN_POINT('Ctrl Pts',(-205.76021269658,-98.5535401563045,10.0080339726105));
#19511=CARTESIAN_POINT('Ctrl Pts',(-202.424513282353,-97.5636768816949,
10.1669422914148));
#19512=CARTESIAN_POINT('Ctrl Pts',(-201.449991305182,-94.2234632956337,
10.3258506102191));
#19513=CARTESIAN_POINT('Ctrl Pts',(-203.730077621707,-91.5951698809454,
10.4847589290234));
#19514=CARTESIAN_POINT('Ctrl Pts',(-207.174414580991,-92.0883866643241,
10.6436672478277));
#19515=CARTESIAN_POINT('Ctrl Pts',(-208.625272555405,-95.2509380113502,
10.802575566632));
#19516=CARTESIAN_POINT('Ctrl Pts',(-206.752521169945,-98.1834321942526,
10.9614838854363));
#19517=CARTESIAN_POINT('Ctrl Pts',(-203.273077963447,-98.1973913220278,
11.1203922042406));
#19518=CARTESIAN_POINT('Ctrl Pts',(-201.37685757861,-95.2800178223495,11.279300523045));
#19519=CARTESIAN_POINT('Ctrl Pts',(-202.802293670589,-92.1059271128426,
11.4382088418493));
#19520=CARTESIAN_POINT('Ctrl Pts',(-206.242562362063,-91.5850900798271,
11.5971171606536));
#19521=CARTESIAN_POINT('Ctrl Pts',(-208.54366376786,-94.1950042938844,11.7560254794579));
#19522=CARTESIAN_POINT('Ctrl Pts',(-207.595973838081,-97.542929574037,11.9149337982622));
#19523=CARTESIAN_POINT('Ctrl Pts',(-204.26832410821,-98.5595254425124,12.0738421170665));
#19524=CARTESIAN_POINT('Ctrl Pts',(-201.611466658146,-96.3127881693687,
12.2327504358708));
#19525=CARTESIAN_POINT('Ctrl Pts',(-202.061178702949,-92.8625013753173,
12.3916587546751));
#19526=CARTESIAN_POINT('Ctrl Pts',(-205.205169266307,-91.3718494299793,
12.5505670734794));
#19527=CARTESIAN_POINT('Ctrl Pts',(-208.161062939416,-93.2074453761791,
12.7094753922837));
#19528=CARTESIAN_POINT('Ctrl Pts',(-208.218929440283,-96.6864353664204,
12.868383711088));
#19529=CARTESIAN_POINT('Ctrl Pts',(-205.325717407468,-98.6193202618013,
13.0272920298923));
#19530=CARTESIAN_POINT('Ctrl Pts',(-202.133891296251,-97.2340527932792,
13.1862003486966));
#19531=CARTESIAN_POINT('Ctrl Pts',(-201.569681610129,-93.8006306939993,
13.3451086675009));
#19532=CARTESIAN_POINT('Ctrl Pts',(-204.150349485118,-91.4667769681704,
13.5040169863052));
#19533=CARTESIAN_POINT('Ctrl Pts',(-207.509967453225,-92.3721426302753,
13.6629253051096));
#19534=CARTESIAN_POINT('Ctrl Pts',(-208.568475318891,-95.6866985528482,
13.8218336239139));
#19535=CARTESIAN_POINT('Ctrl Pts',(-206.355444885374,-98.3716969277542,
13.9807419427182));
#19536=CARTESIAN_POINT('Ctrl Pts',(-202.89975775308,-97.9655612223532,14.1396502615225));
#19537=CARTESIAN_POINT('Ctrl Pts',(-201.36954919205,-94.8406321786314,14.2985585803268));
#19538=CARTESIAN_POINT('Ctrl Pts',(-203.167697451582,-91.8618096795541,
14.4574668991311));
#19539=CARTESIAN_POINT('Ctrl Pts',(-206.64568000845,-91.7600451831499,14.6163752179354));
#19540=CARTESIAN_POINT('Ctrl Pts',(-208.614921940056,-94.6286346539956,
14.7752835367397));
#19541=CARTESIAN_POINT('Ctrl Pts',(-207.270042986249,-97.8376885432202,
14.934191855544));
#19542=CARTESIAN_POINT('Ctrl Pts',(-203.844015760112,-98.4451795972611,
15.0931001743483));
#19543=CARTESIAN_POINT('Ctrl Pts',(-201.477778314385,-95.8941720070566,
15.2520084931526));
#19544=CARTESIAN_POINT('Ctrl Pts',(-202.340681890374,-92.5233902692492,
15.4109168119569));
#19545=CARTESIAN_POINT('Ctrl Pts',(-205.641602982121,-91.4231516321926,
15.5698251307612));
#19546=CARTESIAN_POINT('Ctrl Pts',(-208.35434189336,-93.6020966294465,15.7287334495655));
#19547=CARTESIAN_POINT('Ctrl Pts',(-207.991790944675,-97.0626878467749,
15.8876417683698));
#19548=CARTESIAN_POINT('Ctrl Pts',(-204.886537405266,-98.6320975090182,
16.0465500871742));
#19549=CARTESIAN_POINT('Ctrl Pts',(-201.885019975718,-96.8719144858073,
16.2054584059785));
#19550=CARTESIAN_POINT('Ctrl Pts',(-201.739870914707,-93.3950151743818,
16.3643667247828));
#19551=CARTESIAN_POINT('Ctrl Pts',(-204.582352673002,-91.390717466756,16.5232750435871));
#19552=CARTESIAN_POINT('Ctrl Pts',(-207.810248356741,-92.6929302430059,
16.6821833623914));
#19553=CARTESIAN_POINT('Ctrl Pts',(-208.456461600838,-96.1151764142335,
16.8410916811957));
#19554=CARTESIAN_POINT('Ctrl Pts',(-206.782006578242,-97.7050332130129,
16.9470305603986));
#19555=CARTESIAN_POINT('Ctrl Pts',(-205.793799282533,-97.9692229537457,
17.));
#19556=CARTESIAN_POINT('Ctrl Pts',(-206.913465996665,-93.3640127966251,
0.));
#19557=CARTESIAN_POINT('Ctrl Pts',(-206.975062216132,-93.4218981178264,
-1.31381266890706E-17));
#19558=CARTESIAN_POINT('Ctrl Pts',(-207.033286091207,-93.482935106556,-1.69718597115089E-16));
#19559=CARTESIAN_POINT('Ctrl Pts',(-207.088141399968,-93.5467387008732,
-1.73472347597681E-16));
#19560=CARTESIAN_POINT('Ctrl Pts',(-207.144450725543,-93.6122334988504,
-1.77325596496041E-16));
#19561=CARTESIAN_POINT('Ctrl Pts',(-207.197210975624,-93.68064394337,-2.67124571148989E-16));
#19562=CARTESIAN_POINT('Ctrl Pts',(-207.246400666372,-93.7516020865845,
-2.15105711021124E-16));
#19563=CARTESIAN_POINT('Ctrl Pts',(-207.297350695962,-93.8250995906632,
-1.61225265293368E-16));
#19564=CARTESIAN_POINT('Ctrl Pts',(-207.34447062712,-93.9013309190617,2.27940104476882E-16));
#19565=CARTESIAN_POINT('Ctrl Pts',(-207.38770149442,-93.979931379362,2.35922392732846E-16));
#19566=CARTESIAN_POINT('Ctrl Pts',(-207.406614998863,-94.0143190807433,
2.3941464384483E-16));
#19567=CARTESIAN_POINT('Ctrl Pts',(-207.424783615686,-94.0491607575792,
3.42879087734196E-16));
#19568=CARTESIAN_POINT('Ctrl Pts',(-207.44219995004,-94.0844279691951,3.67761376907083E-16));
#19569=CARTESIAN_POINT('Ctrl Pts',(-207.451657071589,-94.1035781703914,
3.81272534213045E-16));
#19570=CARTESIAN_POINT('Ctrl Pts',(-207.460892353772,-94.122853861087,-1.08199995754127E-16));
#19571=CARTESIAN_POINT('Ctrl Pts',(-207.469904412035,-94.1422506144636,
-1.38777878078145E-16));
#19572=CARTESIAN_POINT('Ctrl Pts',(-207.478555202027,-94.1608698061163,
-1.68129978415293E-16));
#19573=CARTESIAN_POINT('Ctrl Pts',(-207.487002799098,-94.1796065572533,
2.27509235892531E-16));
#19574=CARTESIAN_POINT('Ctrl Pts',(-207.495231872231,-94.1984241373372,
1.94289029309402E-16));
#19575=CARTESIAN_POINT('Ctrl Pts',(-207.531772015166,-94.2819811862123,
4.6778966234489E-17));
#19576=CARTESIAN_POINT('Ctrl Pts',(-207.564052792852,-94.3672219361847,
1.51760739280742E-16));
#19577=CARTESIAN_POINT('Ctrl Pts',(-207.592050671291,-94.4537471119226,
4.16333634234434E-17));
#19578=CARTESIAN_POINT('Ctrl Pts',(-207.620513098777,-94.5417079388662,
-7.03212782969341E-17));
#19579=CARTESIAN_POINT('Ctrl Pts',(-207.64454981266,-94.6309969241772,-2.46766243899794E-16));
#19580=CARTESIAN_POINT('Ctrl Pts',(-207.664096969712,-94.7212317285697,
-3.05311331771918E-16));
#19581=CARTESIAN_POINT('Ctrl Pts',(-207.683346860096,-94.8100942720475,
-3.62966085405676E-16));
#19582=CARTESIAN_POINT('Ctrl Pts',(-207.698242981348,-94.8998749945991,
-1.93681199868498E-16));
#19583=CARTESIAN_POINT('Ctrl Pts',(-207.708681347609,-94.9902317459613,
-1.2490009027033E-16));
#19584=CARTESIAN_POINT('Ctrl Pts',(-207.712775191561,-95.025668942816,-9.79246879459923E-17));
#19585=CARTESIAN_POINT('Ctrl Pts',(-207.716182873916,-95.0611949208303,
-3.69133290614202E-16));
#19586=CARTESIAN_POINT('Ctrl Pts',(-207.718896131003,-95.0967895639108,
-4.02455846426619E-16));
#19587=CARTESIAN_POINT('Ctrl Pts',(-207.720491590831,-95.1177200623165,
-4.22050303371335E-16));
#19588=CARTESIAN_POINT('Ctrl Pts',(-207.721846915935,-95.1386743071217,
-2.20645000857552E-16));
#19589=CARTESIAN_POINT('Ctrl Pts',(-207.722960233087,-95.1596482300522,
-2.22044604925031E-16));
#19590=CARTESIAN_POINT('Ctrl Pts',(-207.723721698985,-95.1739935826248,
-2.2300188000784E-16));
#19591=CARTESIAN_POINT('Ctrl Pts',(-207.724369888774,-95.1883485234433,
-1.87428557882604E-16));
#19592=CARTESIAN_POINT('Ctrl Pts',(-207.724903817588,-95.2026963903353,
-1.94289029309402E-16));
#19593=CARTESIAN_POINT('Ctrl Pts',(-207.728446146415,-95.2978867251433,
-2.39804545795279E-16));
#19594=CARTESIAN_POINT('Ctrl Pts',(-207.726972459038,-95.3929268374015,
-1.01495799011983E-16));
#19595=CARTESIAN_POINT('Ctrl Pts',(-207.720424921853,-95.4874173617819,
-1.11022302462516E-16));
#19596=CARTESIAN_POINT('Ctrl Pts',(-207.713899316081,-95.5815913838534,
-1.2051689625484E-16));
#19597=CARTESIAN_POINT('Ctrl Pts',(-207.702334152436,-95.6752204482728,
-2.71226026961406E-16));
#19598=CARTESIAN_POINT('Ctrl Pts',(-207.685624183999,-95.7679271110661,
-2.77555756156289E-16));
#19599=CARTESIAN_POINT('Ctrl Pts',(-207.683541364687,-95.7794825624354,
-2.7834472725813E-16));
#19600=CARTESIAN_POINT('Ctrl Pts',(-207.681378547894,-95.7910236950498,
-6.25097225611804E-16));
#19601=CARTESIAN_POINT('Ctrl Pts',(-207.679135472956,-95.8025497860598,
-6.38378239159465E-16));
#19602=CARTESIAN_POINT('Ctrl Pts',(-207.661514670061,-95.8930946779994,
-7.71497736738381E-16));
#19603=CARTESIAN_POINT('Ctrl Pts',(-207.638945415372,-95.9827116524882,
-6.42240409036171E-16));
#19604=CARTESIAN_POINT('Ctrl Pts',(-207.611702718408,-96.0711633770076,
-6.93889390390723E-16));
#19605=CARTESIAN_POINT('Ctrl Pts',(-207.600775956761,-96.1066404412793,
-7.14605258182346E-16));
#19606=CARTESIAN_POINT('Ctrl Pts',(-207.589096771976,-96.1419299956307,
-4.97532461527305E-16));
#19607=CARTESIAN_POINT('Ctrl Pts',(-207.576680614638,-96.1770163619212,
-4.71844785465692E-16));
#19608=CARTESIAN_POINT('Ctrl Pts',(-207.570899237935,-96.1933537435407,
-4.59883747287457E-16));
#19609=CARTESIAN_POINT('Ctrl Pts',(-207.564958057168,-96.2096470667711,
2.78109615914965E-16));
#19610=CARTESIAN_POINT('Ctrl Pts',(-207.558858540981,-96.2258947231297,
3.05311331771918E-16));
#19611=CARTESIAN_POINT('Ctrl Pts',(-207.553795015448,-96.2393827474737,
3.27892890464571E-16));
#19612=CARTESIAN_POINT('Ctrl Pts',(-207.54862569686,-96.2528304121624,-4.55940524341242E-16));
#19613=CARTESIAN_POINT('Ctrl Pts',(-207.543352629307,-96.2662349571962,
-4.44089209850063E-16));
#19614=CARTESIAN_POINT('Ctrl Pts',(-207.509118978743,-96.3532595412822,
-3.67148462374673E-16));
#19615=CARTESIAN_POINT('Ctrl Pts',(-207.470506912078,-96.4384928583734,
9.67505829131724E-18));
#19616=CARTESIAN_POINT('Ctrl Pts',(-207.427848909633,-96.5217037647646,
-2.77555756156289E-17));
#19617=CARTESIAN_POINT('Ctrl Pts',(-207.38361239696,-96.6079937948706,-6.65712870024757E-17));
#19618=CARTESIAN_POINT('Ctrl Pts',(-207.33502484806,-96.6921096962562,-3.77517922847587E-16));
#19619=CARTESIAN_POINT('Ctrl Pts',(-207.28240107588,-96.7737901161264,-4.16333634234434E-16));
#19620=CARTESIAN_POINT('Ctrl Pts',(-207.229201427051,-96.8563643876647,
-4.55574116801746E-16));
#19621=CARTESIAN_POINT('Ctrl Pts',(-207.17187631397,-96.9364503981286,-2.0948851905607E-17));
#19622=CARTESIAN_POINT('Ctrl Pts',(-207.11069939243,-97.0137627199881,1.66533453693773E-16));
#19623=CARTESIAN_POINT('Ctrl Pts',(-207.08660648421,-97.0442101277357,2.40368387980402E-16));
#19624=CARTESIAN_POINT('Ctrl Pts',(-207.061915647846,-97.0742271107383,
-6.23795172114093E-17));
#19625=CARTESIAN_POINT('Ctrl Pts',(-207.036641661937,-97.1037951533782,
-5.55111512312578E-17));
#19626=CARTESIAN_POINT('Ctrl Pts',(-207.02229432359,-97.1205801082148,-5.16121710321849E-17));
#19627=CARTESIAN_POINT('Ctrl Pts',(-207.007759045441,-97.1372203785107,
-1.09560184887863E-16));
#19628=CARTESIAN_POINT('Ctrl Pts',(-206.993038388462,-97.1537124668965,
-1.11022302462516E-16));
#19629=CARTESIAN_POINT('Ctrl Pts',(-206.979026737747,-97.1694102297314,
-1.12413998552589E-16));
#19630=CARTESIAN_POINT('Ctrl Pts',(-206.964844314787,-97.1849766172826,
3.77293975944909E-17));
#19631=CARTESIAN_POINT('Ctrl Pts',(-206.9505123113,-97.2003885037202,2.77555756156289E-17));
#19632=CARTESIAN_POINT('Ctrl Pts',(-206.881794715978,-97.2742838091652,
-2.00658656184701E-17));
#19633=CARTESIAN_POINT('Ctrl Pts',(-206.80956588058,-97.3447172801099,-2.86357592693776E-16));
#19634=CARTESIAN_POINT('Ctrl Pts',(-206.734139318221,-97.4114022177255,
-3.33066907387547E-16));
#19635=CARTESIAN_POINT('Ctrl Pts',(-206.669026235039,-97.4689689654876,
-3.7338940648942E-16));
#19636=CARTESIAN_POINT('Ctrl Pts',(-206.601529082945,-97.5237422921457,
-1.64613334688922E-16));
#19637=CARTESIAN_POINT('Ctrl Pts',(-206.531822997772,-97.5755222055268,
-1.66533453693773E-16));
#19638=CARTESIAN_POINT('Ctrl Pts',(-206.504657943773,-97.5957012779787,
-1.67281740393871E-16));
#19639=CARTESIAN_POINT('Ctrl Pts',(-206.477157172808,-97.6154255432419,
-5.71199676364673E-16));
#19640=CARTESIAN_POINT('Ctrl Pts',(-206.449330183025,-97.6346823604932,
-5.55111512312578E-16));
#19641=CARTESIAN_POINT('Ctrl Pts',(-206.434059995963,-97.645249626444,-5.46283059200145E-16));
#19642=CARTESIAN_POINT('Ctrl Pts',(-206.418692843289,-97.6556751456101,
-2.60925414246822E-16));
#19643=CARTESIAN_POINT('Ctrl Pts',(-206.403240459967,-97.665950341847,-2.77555756156289E-16));
#19644=CARTESIAN_POINT('Ctrl Pts',(-206.316661269863,-97.723521924807,-3.70735009069288E-16));
#19645=CARTESIAN_POINT('Ctrl Pts',(-206.227325531817,-97.7764359916984,
-7.1156062831465E-16));
#19646=CARTESIAN_POINT('Ctrl Pts',(-206.135543110803,-97.8243696354571,
-5.55111512312578E-16));
#19647=CARTESIAN_POINT('Ctrl Pts',(-206.043760689789,-97.8723032792159,
-3.98662396310506E-16));
#19648=CARTESIAN_POINT('Ctrl Pts',(-205.949530933876,-97.9152574183469,
-6.03815084515193E-17));
#19649=CARTESIAN_POINT('Ctrl Pts',(-205.853125489076,-97.9528679072037,
1.11022302462516E-16));
#19650=CARTESIAN_POINT('Ctrl Pts',(-205.834025108086,-97.9603195056885,
1.44525943527419E-16));
#19651=CARTESIAN_POINT('Ctrl Pts',(-205.814839220958,-97.9675611910345,
-1.08059395429565E-16));
#19652=CARTESIAN_POINT('Ctrl Pts',(-205.795570948431,-97.974593906276,-1.11022302462516E-16));
#19653=CARTESIAN_POINT('Ctrl Pts',(-202.480282573446,-95.0019224211138,
1.61258330249195));
#19654=CARTESIAN_POINT('Ctrl Pts',(-202.479237170353,-95.125530122547,1.60474993100899));
#19655=CARTESIAN_POINT('Ctrl Pts',(-202.487545208479,-95.2489966935751,
1.59691655952602));
#19656=CARTESIAN_POINT('Ctrl Pts',(-202.505691710494,-95.3709998286824,
1.58908318804305));
#19657=CARTESIAN_POINT('Ctrl Pts',(-202.628398777888,-96.1959878571834,
1.53611374844161));
#19658=CARTESIAN_POINT('Ctrl Pts',(-203.200969189321,-96.9540603402788,
1.48314430884018));
#19659=CARTESIAN_POINT('Ctrl Pts',(-203.960941699756,-97.2977299593421,
1.43017486923874));
#19660=CARTESIAN_POINT('Ctrl Pts',(-204.720914210191,-97.6413995784054,
1.3772054296373));
#19661=CARTESIAN_POINT('Ctrl Pts',(-205.668288819629,-97.5706663334367,
1.32423599003587));
#19662=CARTESIAN_POINT('Ctrl Pts',(-206.368790514116,-97.1179356073323,
1.27126655043443));
#19663=CARTESIAN_POINT('Ctrl Pts',(-207.069292208603,-96.665204881228,1.218297110833));
#19664=CARTESIAN_POINT('Ctrl Pts',(-207.52292098814,-95.830476673988,1.16532767123156));
#19665=CARTESIAN_POINT('Ctrl Pts',(-207.521743785462,-94.9964236518891,
1.11235823163013));
#19666=CARTESIAN_POINT('Ctrl Pts',(-207.520566582783,-94.1623706297901,
1.05938879202869));
#19667=CARTESIAN_POINT('Ctrl Pts',(-207.064583397888,-93.3289927928321,
1.00641935242726));
#19668=CARTESIAN_POINT('Ctrl Pts',(-206.362798185001,-92.8782274828816,
0.95344991282582));
#19669=CARTESIAN_POINT('Ctrl Pts',(-205.661012972115,-92.4274621729311,
0.900480473224384));
#19670=CARTESIAN_POINT('Ctrl Pts',(-204.713425731236,-92.3593093899881,
0.847511033622949));
#19671=CARTESIAN_POINT('Ctrl Pts',(-203.95443862186,-92.70517209454,0.794541594021513));
#19672=CARTESIAN_POINT('Ctrl Pts',(-203.195451512484,-93.0510347990919,
0.741572154420077));
#19673=CARTESIAN_POINT('Ctrl Pts',(-202.625064534611,-93.8109129911388,
0.688602714818642));
#19674=CARTESIAN_POINT('Ctrl Pts',(-202.504670620096,-94.636147652816,0.635633275217206));
#19675=CARTESIAN_POINT('Ctrl Pts',(-202.487207239533,-94.7558496079226,
0.627949950975456));
#19676=CARTESIAN_POINT('Ctrl Pts',(-202.479211752923,-94.8769266689453,
0.620266626733705));
#19677=CARTESIAN_POINT('Ctrl Pts',(-202.480223490507,-94.9981350405341,
0.612583302491955));
#19678=CARTESIAN_POINT('Ctrl Pts',(-204.206200717467,-97.9692229537457,
-1.94289029309402E-15));
#19679=CARTESIAN_POINT('Ctrl Pts',(-203.217993421758,-97.7050332130129,
0.0529694396014337));
#19680=CARTESIAN_POINT('Ctrl Pts',(-201.543538352679,-96.1151767441382,
0.158908318804305));
#19681=CARTESIAN_POINT('Ctrl Pts',(-202.189751683364,-92.692930169225,0.317816637608612));
#19682=CARTESIAN_POINT('Ctrl Pts',(-205.417647323366,-91.3907175644162,
0.476724956412918));
#19683=CARTESIAN_POINT('Ctrl Pts',(-208.260129048284,-93.3950151579563,
0.635633275217225));
#19684=CARTESIAN_POINT('Ctrl Pts',(-208.114979996894,-96.8719144846003,
0.794541594021531));
#19685=CARTESIAN_POINT('Ctrl Pts',(-205.113462590801,-98.6320974631547,
0.953449912825839));
#19686=CARTESIAN_POINT('Ctrl Pts',(-202.00820908717,-97.0626878310035,1.11235823163014));
#19687=CARTESIAN_POINT('Ctrl Pts',(-201.645658139265,-93.6020966408935,
1.27126655043445));
#19688=CARTESIAN_POINT('Ctrl Pts',(-204.358397024947,-91.4231516694834,
1.43017486923876));
#19689=CARTESIAN_POINT('Ctrl Pts',(-207.659318082557,-92.523390293429,1.58908318804306));
#19690=CARTESIAN_POINT('Ctrl Pts',(-208.522221650421,-95.8941719984357,
1.74799150684737));
#19691=CARTESIAN_POINT('Ctrl Pts',(-206.155984228169,-98.445179562461,1.90689982565168));
#19692=CARTESIAN_POINT('Ctrl Pts',(-202.729957036615,-97.8376885148057,
2.06580814445599));
#19693=CARTESIAN_POINT('Ctrl Pts',(-201.385078096233,-94.628634657678,2.22471646326029));
#19694=CARTESIAN_POINT('Ctrl Pts',(-203.3543200081,-91.7600452157265,2.3836247820646));
#19695=CARTESIAN_POINT('Ctrl Pts',(-206.83230253,-91.8618097110707,2.5425331008689));
#19696=CARTESIAN_POINT('Ctrl Pts',(-208.630450771479,-94.8406321802388,
2.70144141967321));
#19697=CARTESIAN_POINT('Ctrl Pts',(-207.100242225817,-97.9655611925551,
2.86034973847752));
#19698=CARTESIAN_POINT('Ctrl Pts',(-203.644555128245,-98.3716968938806,
3.01925805728183));
#19699=CARTESIAN_POINT('Ctrl Pts',(-201.431524716961,-95.6866985459482,
3.17816637608613));
#19700=CARTESIAN_POINT('Ctrl Pts',(-202.490032571993,-92.3721426566775,
3.33707469489044));
#19701=CARTESIAN_POINT('Ctrl Pts',(-205.849650506345,-91.4667770036684,
3.49598301369474));
#19702=CARTESIAN_POINT('Ctrl Pts',(-208.430318355407,-93.8006307060494,
3.65489133249905));
#19703=CARTESIAN_POINT('Ctrl Pts',(-207.866108674953,-97.2340527708336,
3.81379965130336));
#19704=CARTESIAN_POINT('Ctrl Pts',(-204.674282595805,-98.6193202254382,
3.97270797010767));
#19705=CARTESIAN_POINT('Ctrl Pts',(-201.781070592057,-96.6864353494769,
4.13161628891197));
#19706=CARTESIAN_POINT('Ctrl Pts',(-201.838937092343,-93.2074453941888,
4.29052460771628));
#19707=CARTESIAN_POINT('Ctrl Pts',(-204.794830735755,-91.3718494664313,
4.44943292652058));
#19708=CARTESIAN_POINT('Ctrl Pts',(-207.938821267524,-92.8625013967925,
4.60834124532489));
#19709=CARTESIAN_POINT('Ctrl Pts',(-208.38853330781,-96.3127881561792,4.7672495641292));
#19710=CARTESIAN_POINT('Ctrl Pts',(-205.731675884439,-98.55952540675,4.92615788293351));
#19711=CARTESIAN_POINT('Ctrl Pts',(-202.404026188001,-97.5429295484884,
5.08506620173781));
#19712=CARTESIAN_POINT('Ctrl Pts',(-201.456336267743,-94.1950043019721,
5.24397452054212));
#19713=CARTESIAN_POINT('Ctrl Pts',(-203.75743765042,-91.5850901141365,5.40288283934643));
#19714=CARTESIAN_POINT('Ctrl Pts',(-207.19770630733,-92.1059271419192,5.56179115815073));
#19715=CARTESIAN_POINT('Ctrl Pts',(-208.623142384989,-95.2800178195362,
5.72069947695504));
#19716=CARTESIAN_POINT('Ctrl Pts',(-206.726922019203,-98.1973912899037,
5.87960779575934));
#19717=CARTESIAN_POINT('Ctrl Pts',(-203.247478847662,-98.1834321622689,
6.03851611456366));
#19718=CARTESIAN_POINT('Ctrl Pts',(-201.374727481018,-95.250938008829,6.19742443336796));
#19719=CARTESIAN_POINT('Ctrl Pts',(-202.825585440856,-92.088386693577,6.35633275217227));
#19720=CARTESIAN_POINT('Ctrl Pts',(-206.269922365534,-91.5951699151535,
6.51524107097657));
#19721=CARTESIAN_POINT('Ctrl Pts',(-208.550008659151,-94.2234633034355,
6.67414938978088));
#19722=CARTESIAN_POINT('Ctrl Pts',(-207.575486691771,-97.5636768559377,
6.83305770858518));
#19723=CARTESIAN_POINT('Ctrl Pts',(-204.239787311058,-98.5535401206023,
6.9919660273895));
#19724=CARTESIAN_POINT('Ctrl Pts',(-201.601042426826,-96.285557519882,7.1508743461938));
#19725=CARTESIAN_POINT('Ctrl Pts',(-202.078423856235,-92.8389901533445,
7.30978266499811));
#19726=CARTESIAN_POINT('Ctrl Pts',(-205.234273640395,-91.3736124610605,
7.46869098380241));
#19727=CARTESIAN_POINT('Ctrl Pts',(-208.175343969469,-93.2328663330924,
7.62759930260672));
#19728=CARTESIAN_POINT('Ctrl Pts',(-208.205294437497,-96.7122086000577,
7.78650762141102));
#19729=CARTESIAN_POINT('Ctrl Pts',(-205.296666790141,-98.6218171594914,
7.94541594021533));
#19730=CARTESIAN_POINT('Ctrl Pts',(-202.116058345367,-97.2109842274052,
8.10432425901964));
#19731=CARTESIAN_POINT('Ctrl Pts',(-201.579415376341,-93.7731456673473,
8.26323257782395));
#19732=CARTESIAN_POINT('Ctrl Pts',(-204.178726159118,-91.4600734471682,
8.42214089662825));
#19733=CARTESIAN_POINT('Ctrl Pts',(-207.530971620008,-92.3923663255981,
8.58104921543255));
#19734=CARTESIAN_POINT('Ctrl Pts',(-208.562850587821,-95.7153086117373,
8.73995753423687));
#19735=CARTESIAN_POINT('Ctrl Pts',(-206.328347957964,-98.382463957492,8.89886585304117));
#19736=CARTESIAN_POINT('Ctrl Pts',(-202.876030766917,-97.9486141521186,
9.05777417184548));
#19737=CARTESIAN_POINT('Ctrl Pts',(-201.370944829595,-94.8115078481334,
9.21668249064979));
#19738=CARTESIAN_POINT('Ctrl Pts',(-203.192936111301,-91.8472090422419,
9.3755908094541));
#19739=CARTESIAN_POINT('Ctrl Pts',(-206.671623368988,-91.7733537483301,
9.53449912825839));
#19740=CARTESIAN_POINT('Ctrl Pts',(-208.617785005374,-94.6576516743914,
9.69340744706271));
#19741=CARTESIAN_POINT('Ctrl Pts',(-207.247201784069,-97.8558107190141,
9.85231576586701));
#19742=CARTESIAN_POINT('Ctrl Pts',(-203.816409083639,-98.4357944152506,
10.0112240846713));
#19743=CARTESIAN_POINT('Ctrl Pts',(-201.470719306577,-95.8658801927493,
10.1701324034756));
#19744=CARTESIAN_POINT('Ctrl Pts',(-202.360634623205,-92.5021366872992,
10.3290407222799));
#19745=CARTESIAN_POINT('Ctrl Pts',(-205.670290617637,-91.4284063488314,
10.4879490410842));
#19746=CARTESIAN_POINT('Ctrl Pts',(-208.365431665519,-93.6290731507911,
10.6468573598885));
#19747=CARTESIAN_POINT('Ctrl Pts',(-207.975182577187,-97.0865903655397,
10.8057656786929));
#19748=CARTESIAN_POINT('Ctrl Pts',(-204.85731935509,-98.6311448545504,10.9646739974972));
#19749=CARTESIAN_POINT('Ctrl Pts',(-201.870264153535,-96.8467063254648,
11.1235823163015));
#19750=CARTESIAN_POINT('Ctrl Pts',(-201.752515795608,-93.3692280774477,
11.2824906351058));
#19751=CARTESIAN_POINT('Ctrl Pts',(-204.612024659808,-91.3868233012261,
11.4413989539101));
#19752=CARTESIAN_POINT('Ctrl Pts',(-207.827224979576,-92.7169385387114,
11.6003072727144));
#19753=CARTESIAN_POINT('Ctrl Pts',(-208.450457037378,-96.1401390066001,
11.7592155915187));
#19754=CARTESIAN_POINT('Ctrl Pts',(-205.910348648356,-98.5180727763361,
11.918123910323));
#19755=CARTESIAN_POINT('Ctrl Pts',(-202.5356427933,-97.6706767454985,12.0770322291273));
#19756=CARTESIAN_POINT('Ctrl Pts',(-201.420232081736,-94.374834123991,12.2359405479316));
#19757=CARTESIAN_POINT('Ctrl Pts',(-203.58671258731,-91.6521365902563,12.3948488667359));
#19758=CARTESIAN_POINT('Ctrl Pts',(-207.048879196816,-91.9987228122024,
12.5537571855402));
#19759=CARTESIAN_POINT('Ctrl Pts',(-208.632656258583,-95.0968464152565,
12.7126655043445));
#19760=CARTESIAN_POINT('Ctrl Pts',(-206.886054663924,-98.1061823072572,
12.8715738231488));
#19761=CARTESIAN_POINT('Ctrl Pts',(-203.410339233432,-98.2678049770775,
13.0304821419532));
#19762=CARTESIAN_POINT('Ctrl Pts',(-201.392007026401,-95.4335405675857,
13.1893904607575));
#19763=CARTESIAN_POINT('Ctrl Pts',(-202.681442451813,-92.2018110111346,
13.3482987795618));
#19764=CARTESIAN_POINT('Ctrl Pts',(-206.096505523284,-91.5354298452884,
13.5072070983661));
#19765=CARTESIAN_POINT('Ctrl Pts',(-208.506304586591,-94.045327873685,13.6661154171704));
#19766=CARTESIAN_POINT('Ctrl Pts',(-207.701562793806,-97.4304586389942,
13.8250237359747));
#19767=CARTESIAN_POINT('Ctrl Pts',(-204.420058427186,-98.5873720853337,
13.983932054779));
#19768=CARTESIAN_POINT('Ctrl Pts',(-201.670238011152,-96.4554229063367,
14.1428403735833));
#19769=CARTESIAN_POINT('Ctrl Pts',(-201.973106173498,-92.989158258924,14.3017486923876));
#19770=CARTESIAN_POINT('Ctrl Pts',(-205.050996758677,-91.3664108756636,
14.4606570111919));
#19771=CARTESIAN_POINT('Ctrl Pts',(-208.082134098584,-93.0748973262563,
14.6195653299962));
#19772=CARTESIAN_POINT('Ctrl Pts',(-208.287605318196,-96.548296522874,14.7784736488005));
#19773=CARTESIAN_POINT('Ctrl Pts',(-205.479036782975,-98.6022345010335,
14.9373819676048));
#19774=CARTESIAN_POINT('Ctrl Pts',(-202.231292563431,-97.3536847109377,
15.0962902864091));
#19775=CARTESIAN_POINT('Ctrl Pts',(-201.521868615849,-93.9473019249279,
15.2551986052134));
#19776=CARTESIAN_POINT('Ctrl Pts',(-204.001156151974,-91.5060233657571,
15.4141069240177));
#19777=CARTESIAN_POINT('Ctrl Pts',(-207.396173587353,-92.2679785768132,
15.5730152428221));
#19778=CARTESIAN_POINT('Ctrl Pts',(-208.594403743819,-95.5346307410897,
15.7319235616264));
#19779=CARTESIAN_POINT('Ctrl Pts',(-206.497329095757,-98.3111182304646,
15.8908318804307));
#19780=CARTESIAN_POINT('Ctrl Pts',(-203.027510825076,-98.0520533374907,
16.049740199235));
#19781=CARTESIAN_POINT('Ctrl Pts',(-201.36606728008,-94.9948094934893,16.2086485180393));
#19782=CARTESIAN_POINT('Ctrl Pts',(-203.036133983161,-91.9425114866494,
16.3675568368436));
#19783=CARTESIAN_POINT('Ctrl Pts',(-206.506731020769,-91.6928976656653,
16.5264651556479));
#19784=CARTESIAN_POINT('Ctrl Pts',(-208.595808729299,-94.4759987242795,
16.6853734744522));
#19785=CARTESIAN_POINT('Ctrl Pts',(-207.388631352792,-97.7378439047888,
16.8442817932565));
#19786=CARTESIAN_POINT('Ctrl Pts',(-203.990889000222,-98.4931020304819,
17.0031901120608));
#19787=CARTESIAN_POINT('Ctrl Pts',(-201.519840830385,-96.0388640162284,
17.1620984308651));
#19788=CARTESIAN_POINT('Ctrl Pts',(-201.999201820237,-93.780179352227,17.268037310068));
#19789=CARTESIAN_POINT('Ctrl Pts',(-202.663937342304,-93.0026984430694,
17.3210067496694));
#19790=CARTESIAN_POINT('Ctrl Pts',(-204.254067145653,-97.7901775698422,
-0.107002249889813));
#19791=CARTESIAN_POINT('Ctrl Pts',(-203.325449162499,-97.5419185807874,
-0.054032810288377));
#19792=CARTESIAN_POINT('Ctrl Pts',(-201.75196443325,-96.047931120827,0.0519060689144942));
#19793=CARTESIAN_POINT('Ctrl Pts',(-202.35921083027,-92.8320474433327,0.210814387718801));
#19794=CARTESIAN_POINT('Ctrl Pts',(-205.39246301538,-91.6083588023301,0.369722706523108));
#19795=CARTESIAN_POINT('Ctrl Pts',(-208.063541905413,-93.4917964140895,
0.528631025327414));
#19796=CARTESIAN_POINT('Ctrl Pts',(-207.927145402428,-96.7590372595651,
0.687539344131721));
#19797=CARTESIAN_POINT('Ctrl Pts',(-205.106620749199,-98.4130804695519,
0.846447662936027));
#19798=CARTESIAN_POINT('Ctrl Pts',(-202.18861532843,-96.9383068935231,1.00535598174034));
#19799=CARTESIAN_POINT('Ctrl Pts',(-201.847926354066,-93.686390797139,1.16426430054464));
#19800=CARTESIAN_POINT('Ctrl Pts',(-204.397085952243,-91.638837117319,1.32317261934895));
#19801=CARTESIAN_POINT('Ctrl Pts',(-207.498960091786,-92.6727308928383,
1.48208093815325));
#19802=CARTESIAN_POINT('Ctrl Pts',(-208.309830214205,-95.8402530535703,
1.64098925695756));
#19803=CARTESIAN_POINT('Ctrl Pts',(-206.086277896531,-98.2374337963173,
1.79989757576187));
#19804=CARTESIAN_POINT('Ctrl Pts',(-202.866841575158,-97.6665747124921,
1.95880589456617));
#19805=CARTESIAN_POINT('Ctrl Pts',(-201.603059396433,-94.6510281428828,
2.11771421337048));
#19806=CARTESIAN_POINT('Ctrl Pts',(-203.453555198761,-91.9554158420543,
2.27662253217479));
#19807=CARTESIAN_POINT('Ctrl Pts',(-206.721813922367,-92.0510438958378,
2.4355308509791));
#19808=CARTESIAN_POINT('Ctrl Pts',(-208.411533074072,-94.8502421263141,
2.5944391697834));
#19809=CARTESIAN_POINT('Ctrl Pts',(-206.973596742648,-97.7867366143803,
2.75334748858771));
#19810=CARTESIAN_POINT('Ctrl Pts',(-203.726289019975,-98.1683821633347,
2.91225580739202));
#19811=CARTESIAN_POINT('Ctrl Pts',(-201.646705266537,-95.645290336898,3.07116412619632));
#19812=CARTESIAN_POINT('Ctrl Pts',(-202.641384655933,-92.5306035517361,
3.23007244500063));
#19813=CARTESIAN_POINT('Ctrl Pts',(-205.798416226043,-91.6798318256369,
3.38898076380493));
#19814=CARTESIAN_POINT('Ctrl Pts',(-208.223468726254,-93.8729531752686,
3.54788908260924));
#19815=CARTESIAN_POINT('Ctrl Pts',(-207.693281125116,-97.0993384559284,
3.70679740141355));
#19816=CARTESIAN_POINT('Ctrl Pts',(-204.69392349128,-98.4010737046049,3.86570572021786));
#19817=CARTESIAN_POINT('Ctrl Pts',(-201.975173379413,-96.584742593736,4.02461403902216));
#19818=CARTESIAN_POINT('Ctrl Pts',(-202.02955050557,-93.3155371853966,4.18352235782647));
#19819=CARTESIAN_POINT('Ctrl Pts',(-204.807202528057,-91.5906284585319,
4.34243067663077));
#19820=CARTESIAN_POINT('Ctrl Pts',(-207.761609117994,-92.9913934550739,
4.50133899543508));
#19821=CARTESIAN_POINT('Ctrl Pts',(-208.184203334474,-96.2336264822096,
4.66024731423938));
#19822=CARTESIAN_POINT('Ctrl Pts',(-205.687555523098,-98.3448845384508,
4.8191556330437));
#19823=CARTESIAN_POINT('Ctrl Pts',(-202.560564492808,-97.3895898349197,
4.978063951848));
#19824=CARTESIAN_POINT('Ctrl Pts',(-201.670020670447,-94.2435458786875,
5.13697227065231));
#19825=CARTESIAN_POINT('Ctrl Pts',(-203.832364678929,-91.7910106061423,
5.29588058945662));
#19826=CARTESIAN_POINT('Ctrl Pts',(-207.065183699351,-92.2804409436754,
5.45478890826092));
#19827=CARTESIAN_POINT('Ctrl Pts',(-208.404665386339,-95.2631326280973,
5.61369722706523));
#19828=CARTESIAN_POINT('Ctrl Pts',(-206.622787900372,-98.0045872600586,
5.77260554586953));
#19829=CARTESIAN_POINT('Ctrl Pts',(-203.35315660491,-97.9914698736489,5.93151386467385));
#19830=CARTESIAN_POINT('Ctrl Pts',(-201.593332927638,-95.235806342118,6.09042218347814));
#19831=CARTESIAN_POINT('Ctrl Pts',(-202.956703546694,-92.2639581916921,
6.24933050228246));
#19832=CARTESIAN_POINT('Ctrl Pts',(-206.193345516639,-91.8004825909493,
6.40823882108676));
#19833=CARTESIAN_POINT('Ctrl Pts',(-208.335941654706,-94.2702887904795,
6.56714713989107));
#19834=CARTESIAN_POINT('Ctrl Pts',(-207.420183768868,-97.4090860710669,
6.72605545869537));
#19835=CARTESIAN_POINT('Ctrl Pts',(-204.285628453626,-98.3392601675569,
6.88496377749969));
#19836=CARTESIAN_POINT('Ctrl Pts',(-201.806000987716,-96.2080378646515,
7.04387209630398));
#19837=CARTESIAN_POINT('Ctrl Pts',(-202.254596117602,-92.9692999494227,
7.20278041510831));
#19838=CARTESIAN_POINT('Ctrl Pts',(-205.220146842058,-91.5922851438489,
7.36168873391259));
#19839=CARTESIAN_POINT('Ctrl Pts',(-207.983869402252,-93.3394252310698,
7.52059705271691));
#19840=CARTESIAN_POINT('Ctrl Pts',(-208.012013844552,-96.6089617065452,
7.67950537152121));
#19841=CARTESIAN_POINT('Ctrl Pts',(-205.278777658823,-98.4034200724921,
7.83841369032552));
#19842=CARTESIAN_POINT('Ctrl Pts',(-202.289961231325,-97.0776609553009,
7.99732200912983));
#19843=CARTESIAN_POINT('Ctrl Pts',(-201.785678057406,-93.8471254958766,
8.15623032793413));
#19844=CARTESIAN_POINT('Ctrl Pts',(-204.228249314645,-91.6735324963928,
8.31513864673845));
#19845=CARTESIAN_POINT('Ctrl Pts',(-207.37835297452,-92.5496077249763,8.47404696554274));
#19846=CARTESIAN_POINT('Ctrl Pts',(-208.348009209715,-95.6721752037739,
8.63295528434706));
#19847=CARTESIAN_POINT('Ctrl Pts',(-206.24824802145,-98.1784999685146,8.79186360315136));
#19848=CARTESIAN_POINT('Ctrl Pts',(-203.00410699853,-97.7708114875583,8.95077192195567));
#19849=CARTESIAN_POINT('Ctrl Pts',(-201.589778371674,-94.8228740035955,
9.10968024075998));
#19850=CARTESIAN_POINT('Ctrl Pts',(-203.301902818326,-92.0373236534358,
9.26858855956428));
#19851=CARTESIAN_POINT('Ctrl Pts',(-206.570823781855,-91.967921864585,9.42749687836858));
#19852=CARTESIAN_POINT('Ctrl Pts',(-208.399631058952,-94.6782954213725,
9.5864051971729));
#19853=CARTESIAN_POINT('Ctrl Pts',(-207.111694578176,-97.6836041402198,
9.7453135159772));
#19854=CARTESIAN_POINT('Ctrl Pts',(-203.887780110101,-98.2286145774026,
9.90422183478151));
#19855=CARTESIAN_POINT('Ctrl Pts',(-201.683536406035,-95.81366725558,10.0631301535858));
#19856=CARTESIAN_POINT('Ctrl Pts',(-202.519789457487,-92.6527588880325,
10.2220384723901));
#19857=CARTESIAN_POINT('Ctrl Pts',(-205.629871813515,-91.6437749373083,
10.3809467911944));
#19858=CARTESIAN_POINT('Ctrl Pts',(-208.162494730859,-93.7117406122259,
10.5398551099987));
#19859=CARTESIAN_POINT('Ctrl Pts',(-207.795777825502,-96.9607680952463,
10.698763428803));
#19860=CARTESIAN_POINT('Ctrl Pts',(-204.865923057554,-98.4121853036442,
10.8576717476073));
#19861=CARTESIAN_POINT('Ctrl Pts',(-202.058988531892,-96.735349162951,11.0165800664117));
#19862=CARTESIAN_POINT('Ctrl Pts',(-201.948340449113,-93.4675643053029,
11.175488385216));
#19863=CARTESIAN_POINT('Ctrl Pts',(-204.63541973482,-91.6046993648363,11.3343967040203));
#19864=CARTESIAN_POINT('Ctrl Pts',(-207.656742132806,-92.8546080981145,
11.4933050228246));
#19865=CARTESIAN_POINT('Ctrl Pts',(-208.242393037293,-96.0713881484396,
11.6522133416289));
#19866=CARTESIAN_POINT('Ctrl Pts',(-205.855454244746,-98.3059315189592,
11.8111216604332));
#19867=CARTESIAN_POINT('Ctrl Pts',(-202.684244561852,-97.5096338226097,
11.9700299792375));
#19868=CARTESIAN_POINT('Ctrl Pts',(-201.636093581931,-94.412531887351,12.1289382980418));
#19869=CARTESIAN_POINT('Ctrl Pts',(-203.671934408411,-91.854014151757,12.2878466168461));
#19870=CARTESIAN_POINT('Ctrl Pts',(-206.925330925743,-92.1797010798036,
12.4467549356504));
#19871=CARTESIAN_POINT('Ctrl Pts',(-208.413605569382,-95.0910065359784,
12.6056632544547));
#19872=CARTESIAN_POINT('Ctrl Pts',(-206.772324780171,-97.9188782171498,
12.764571573259));
#19873=CARTESIAN_POINT('Ctrl Pts',(-203.506196441416,-98.0707549724947,
12.9234798920633));
#19874=CARTESIAN_POINT('Ctrl Pts',(-201.609570509219,-95.4073978903364,
13.0823882108676));
#19875=CARTESIAN_POINT('Ctrl Pts',(-202.821252440078,-92.3705429755409,
13.241296529672));
#19876=CARTESIAN_POINT('Ctrl Pts',(-206.030385782386,-91.7443448722414,
13.4002048484763));
#19877=CARTESIAN_POINT('Ctrl Pts',(-208.29487295597,-94.1028950015231,13.5591131672806));
#19878=CARTESIAN_POINT('Ctrl Pts',(-207.538657429308,-97.28390096823,13.7180214860849));
#19879=CARTESIAN_POINT('Ctrl Pts',(-204.45502914618,-98.3710520506886,13.8769298048892));
#19880=CARTESIAN_POINT('Ctrl Pts',(-201.871024049414,-96.3676602973758,
14.0358381236935));
#19881=CARTESIAN_POINT('Ctrl Pts',(-202.155629135109,-93.1104128555335,
14.1947464424978));
#19882=CARTESIAN_POINT('Ctrl Pts',(-205.047921632835,-91.5855178170584,
14.3536547613021));
#19883=CARTESIAN_POINT('Ctrl Pts',(-207.896280125501,-93.1909818213055,
14.5125630801064));
#19884=CARTESIAN_POINT('Ctrl Pts',(-208.089361344776,-96.4549335960568,
14.6714713989107));
#19885=CARTESIAN_POINT('Ctrl Pts',(-205.450150664941,-98.3850182565158,
14.830379717715));
#19886=CARTESIAN_POINT('Ctrl Pts',(-202.398246777924,-97.2117565400922,
14.9892880365193));
#19887=CARTESIAN_POINT('Ctrl Pts',(-201.7316013906,-94.0107800584065,15.1481963553236));
#19888=CARTESIAN_POINT('Ctrl Pts',(-204.061386853075,-91.7167116157045,
15.3071046741279));
#19889=CARTESIAN_POINT('Ctrl Pts',(-207.251683319518,-92.4327206093809,
15.4660129929323));
#19890=CARTESIAN_POINT('Ctrl Pts',(-208.377659697231,-95.5023922841682,
15.6249213117365));
#19891=CARTESIAN_POINT('Ctrl Pts',(-206.407039526077,-98.1114564186172,
15.7838296305409));
#19892=CARTESIAN_POINT('Ctrl Pts',(-203.146452745933,-97.8680132468618,
15.9427379493452));
#19893=CARTESIAN_POINT('Ctrl Pts',(-201.585194940432,-94.9951224831991,
16.1016462681495));
#19894=CARTESIAN_POINT('Ctrl Pts',(-203.154555923984,-92.1268793206523,
16.2605545869538));
#19895=CARTESIAN_POINT('Ctrl Pts',(-206.415874511084,-91.8923173172992,
16.4194629057581));
#19896=CARTESIAN_POINT('Ctrl Pts',(-208.3789799615,-94.507596220001,16.5783712245624));
#19897=CARTESIAN_POINT('Ctrl Pts',(-207.24459588485,-97.5727507741492,16.7372795433667));
#19898=CARTESIAN_POINT('Ctrl Pts',(-204.051738814861,-98.2824665195066,
16.896187862171));
#19899=CARTESIAN_POINT('Ctrl Pts',(-201.729695881446,-95.9762200822744,
17.0550961809753));
#19900=CARTESIAN_POINT('Ctrl Pts',(-202.180151203454,-93.8537350466212,
17.1610350601782));
#19901=CARTESIAN_POINT('Ctrl Pts',(-202.804802895981,-93.1231365609213,
17.2140044997796));
#19902=CARTESIAN_POINT('Ctrl Pts',(-204.301933573839,-97.6111321859386,
-0.214004499779623));
#19903=CARTESIAN_POINT('Ctrl Pts',(-203.43290490324,-97.3788039485619,-0.161035060178188));
#19904=CARTESIAN_POINT('Ctrl Pts',(-201.960390513822,-95.9806854975158,
-0.0550961809753165));
#19905=CARTESIAN_POINT('Ctrl Pts',(-202.528669977177,-92.9711647174406,
0.10381213782899));
#19906=CARTESIAN_POINT('Ctrl Pts',(-205.367278707393,-91.8260000402438,
0.262720456633297));
#19907=CARTESIAN_POINT('Ctrl Pts',(-207.866954762541,-93.5885776702228,
0.421628775437603));
#19908=CARTESIAN_POINT('Ctrl Pts',(-207.739310807963,-96.6461600345297,
0.580537094241911));
#19909=CARTESIAN_POINT('Ctrl Pts',(-205.099778907598,-98.1940634759493,
0.739445413046217));
#19910=CARTESIAN_POINT('Ctrl Pts',(-202.369021569689,-96.8139259560427,
0.898353731850524));
#19911=CARTESIAN_POINT('Ctrl Pts',(-202.050194568866,-93.7706849533848,
1.05726205065483));
#19912=CARTESIAN_POINT('Ctrl Pts',(-204.435774879538,-91.8545225651544,
1.21617036945914));
#19913=CARTESIAN_POINT('Ctrl Pts',(-207.338602101016,-92.8220714922477,
1.37507868826344));
#19914=CARTESIAN_POINT('Ctrl Pts',(-208.097438777988,-95.786334108705,1.53398700706775));
#19915=CARTESIAN_POINT('Ctrl Pts',(-206.016571564894,-98.0296880301736,
1.69289532587206));
#19916=CARTESIAN_POINT('Ctrl Pts',(-203.003726113702,-97.4954609101786,
1.85180364467636));
#19917=CARTESIAN_POINT('Ctrl Pts',(-201.821040696633,-94.6734216280877,
2.01071196348067));
#19918=CARTESIAN_POINT('Ctrl Pts',(-203.552790389423,-92.1507864683822,
2.16962028228498));
#19919=CARTESIAN_POINT('Ctrl Pts',(-206.611325314735,-92.2402780806049,
2.32852860108928));
#19920=CARTESIAN_POINT('Ctrl Pts',(-208.192615376664,-94.8598520723894,
2.48743691989359));
#19921=CARTESIAN_POINT('Ctrl Pts',(-206.84695125948,-97.6079120362055,2.6463452386979));
#19922=CARTESIAN_POINT('Ctrl Pts',(-203.808022911705,-97.9650674327889,
2.8052535575022));
#19923=CARTESIAN_POINT('Ctrl Pts',(-201.861885816114,-95.6038821278479,
2.96416187630651));
#19924=CARTESIAN_POINT('Ctrl Pts',(-202.792736739874,-92.6890644467946,
3.12307019511082));
#19925=CARTESIAN_POINT('Ctrl Pts',(-205.747181945741,-91.8928866476054,
3.28197851391513));
#19926=CARTESIAN_POINT('Ctrl Pts',(-208.0166190971,-93.9452756444879,3.44088683271943));
#19927=CARTESIAN_POINT('Ctrl Pts',(-207.520453575278,-96.9646241410233,
3.59979515152374));
#19928=CARTESIAN_POINT('Ctrl Pts',(-204.713564386756,-98.1828271837715,
3.75870347032805));
#19929=CARTESIAN_POINT('Ctrl Pts',(-202.169276166769,-96.4830498379951,
3.91761178913235));
#19930=CARTESIAN_POINT('Ctrl Pts',(-202.220163918797,-93.4236289766044,
4.07652010793666));
#19931=CARTESIAN_POINT('Ctrl Pts',(-204.819574320358,-91.8094074506325,
4.23542842674097));
#19932=CARTESIAN_POINT('Ctrl Pts',(-207.584396968464,-93.1202855133552,
4.39433674554527));
#19933=CARTESIAN_POINT('Ctrl Pts',(-207.979873361138,-96.1544648082402,
4.55324506434958));
#19934=CARTESIAN_POINT('Ctrl Pts',(-205.643435161757,-98.1302436701516,
4.71215338315388));
#19935=CARTESIAN_POINT('Ctrl Pts',(-202.717102797615,-97.236250121351,4.8710617019582));
#19936=CARTESIAN_POINT('Ctrl Pts',(-201.883705073152,-94.2920874554028,
5.02997002076249));
#19937=CARTESIAN_POINT('Ctrl Pts',(-203.907291707438,-91.9969310981482,
5.18887833956681));
#19938=CARTESIAN_POINT('Ctrl Pts',(-206.932661091371,-92.4549547454316,
5.34778665837111));
#19939=CARTESIAN_POINT('Ctrl Pts',(-208.186188387689,-95.2462474366585,
5.50669497717542));
#19940=CARTESIAN_POINT('Ctrl Pts',(-206.518653781542,-97.8117832302136,
5.66560329597972));
#19941=CARTESIAN_POINT('Ctrl Pts',(-203.458834362157,-97.7995075850287,
5.82451161478403));
#19942=CARTESIAN_POINT('Ctrl Pts',(-201.811938374257,-95.220674675407,5.98341993358834));
#19943=CARTESIAN_POINT('Ctrl Pts',(-203.087821652533,-92.4395296898073,
6.14232825239265));
#19944=CARTESIAN_POINT('Ctrl Pts',(-206.116768667744,-92.0057952667451,
6.30123657119695));
#19945=CARTESIAN_POINT('Ctrl Pts',(-208.12187465026,-94.3171142775237,6.46014489000126));
#19946=CARTESIAN_POINT('Ctrl Pts',(-207.264880845966,-97.2544952861959,
6.61905320880556));
#19947=CARTESIAN_POINT('Ctrl Pts',(-204.331469596194,-98.1249802145116,
6.77796152760988));
#19948=CARTESIAN_POINT('Ctrl Pts',(-202.010959548606,-96.1305182094207,
6.93686984641417));
#19949=CARTESIAN_POINT('Ctrl Pts',(-202.430768378969,-93.0996097455012,
7.0957781652185));
#19950=CARTESIAN_POINT('Ctrl Pts',(-205.206020043722,-91.8109578266372,
7.25468648402278));
#19951=CARTESIAN_POINT('Ctrl Pts',(-207.792394835035,-93.4459841290473,
7.4135948028271));
#19952=CARTESIAN_POINT('Ctrl Pts',(-207.818733251607,-96.5057148130326,
7.5725031216314));
#19953=CARTESIAN_POINT('Ctrl Pts',(-205.260888527505,-98.1850229854928,
7.73141144043571));
#19954=CARTESIAN_POINT('Ctrl Pts',(-202.463864117283,-96.9443376831967,
7.89031975924002));
#19955=CARTESIAN_POINT('Ctrl Pts',(-201.99194073847,-93.921105324406,8.04922807804432));
#19956=CARTESIAN_POINT('Ctrl Pts',(-204.277772470171,-91.8869915456173,
8.20813639684863));
#19957=CARTESIAN_POINT('Ctrl Pts',(-207.225734329031,-92.7068491243547,
8.36704471565294));
#19958=CARTESIAN_POINT('Ctrl Pts',(-208.133167831608,-95.6290417958106,
8.52595303445724));
#19959=CARTESIAN_POINT('Ctrl Pts',(-206.168148084936,-97.9745359795373,
8.68486135326155));
#19960=CARTESIAN_POINT('Ctrl Pts',(-203.132183230144,-97.5930088229981,
8.84376967206586));
#19961=CARTESIAN_POINT('Ctrl Pts',(-201.808611913754,-94.8342401590575,
9.00267799087016));
#19962=CARTESIAN_POINT('Ctrl Pts',(-203.41086952535,-92.2274382646298,9.16158630967448));
#19963=CARTESIAN_POINT('Ctrl Pts',(-206.470024194722,-92.1624899808399,
9.32049462847878));
#19964=CARTESIAN_POINT('Ctrl Pts',(-208.18147711253,-94.6989391683534,9.47940294728308));
#19965=CARTESIAN_POINT('Ctrl Pts',(-206.976187372282,-97.5113975614257,
9.63831126608739));
#19966=CARTESIAN_POINT('Ctrl Pts',(-203.959151136564,-98.0214347395542,
9.7972195848917));
#19967=CARTESIAN_POINT('Ctrl Pts',(-201.896353505491,-95.7614543184109,
9.956127903696));
#19968=CARTESIAN_POINT('Ctrl Pts',(-202.678944291769,-92.8033810887658,
10.1150362225003));
#19969=CARTESIAN_POINT('Ctrl Pts',(-205.589453009393,-91.859143525785,10.2739445413046));
#19970=CARTESIAN_POINT('Ctrl Pts',(-207.9595577962,-93.7944080736608,10.4328528601089));
#19971=CARTESIAN_POINT('Ctrl Pts',(-207.616373073816,-96.8349458249529,
10.5917611789132));
#19972=CARTESIAN_POINT('Ctrl Pts',(-204.874526760019,-98.1932257527382,
10.7506694977175));
#19973=CARTESIAN_POINT('Ctrl Pts',(-202.247712910248,-96.6239920004371,
10.9095778165219));
#19974=CARTESIAN_POINT('Ctrl Pts',(-202.144165102618,-93.5659005331583,
11.0684861353261));
#19975=CARTESIAN_POINT('Ctrl Pts',(-204.658814809832,-91.8225754284465,
11.2273944541305));
#19976=CARTESIAN_POINT('Ctrl Pts',(-207.486259286036,-92.9922776575177,
11.3863027729348));
#19977=CARTESIAN_POINT('Ctrl Pts',(-208.034329037208,-96.0026372902789,
11.5452110917391));
#19978=CARTESIAN_POINT('Ctrl Pts',(-205.800559841136,-98.0937902615824,
11.7041194105434));
#19979=CARTESIAN_POINT('Ctrl Pts',(-202.832846330403,-97.3485908997207,
11.8630277293477));
#19980=CARTESIAN_POINT('Ctrl Pts',(-201.851955082127,-94.4502296507111,
12.021936048152));
#19981=CARTESIAN_POINT('Ctrl Pts',(-203.757156229511,-92.0558917132578,
12.1808443669563));
#19982=CARTESIAN_POINT('Ctrl Pts',(-206.80178265467,-92.3606793474046,12.3397526857606));
#19983=CARTESIAN_POINT('Ctrl Pts',(-208.194554880182,-95.0851666567005,
12.4986610045649));
#19984=CARTESIAN_POINT('Ctrl Pts',(-206.658594896419,-97.7315741270424,
12.6575693233692));
#19985=CARTESIAN_POINT('Ctrl Pts',(-203.602053649399,-97.8737049679119,
12.8164776421735));
#19986=CARTESIAN_POINT('Ctrl Pts',(-201.827133992036,-95.3812552130871,
12.9753859609778));
#19987=CARTESIAN_POINT('Ctrl Pts',(-202.961062428342,-92.5392749399473,
13.1342942797821));
#19988=CARTESIAN_POINT('Ctrl Pts',(-205.964266041489,-91.9532598991944,
13.2932025985864));
#19989=CARTESIAN_POINT('Ctrl Pts',(-208.083441325348,-94.1604621293612,
13.4521109173908));
#19990=CARTESIAN_POINT('Ctrl Pts',(-207.375752064809,-97.1373432974659,
13.6110192361951));
#19991=CARTESIAN_POINT('Ctrl Pts',(-204.489999865174,-98.1547320160434,
13.7699275549994));
#19992=CARTESIAN_POINT('Ctrl Pts',(-202.071810087677,-96.2798976884151,
13.9288358738037));
#19993=CARTESIAN_POINT('Ctrl Pts',(-202.33815209672,-93.231667452143,14.087744192608));
#19994=CARTESIAN_POINT('Ctrl Pts',(-205.044846506994,-91.8046247584532,
14.2466525114123));
#19995=CARTESIAN_POINT('Ctrl Pts',(-207.710426152417,-93.3070663163548,
14.4055608302166));
#19996=CARTESIAN_POINT('Ctrl Pts',(-207.891117371357,-96.3615706692395,
14.5644691490209));
#19997=CARTESIAN_POINT('Ctrl Pts',(-205.421264546907,-98.1678020119983,
14.7233774678252));
#19998=CARTESIAN_POINT('Ctrl Pts',(-202.565200992417,-97.0698283692467,
14.8822857866295));
#19999=CARTESIAN_POINT('Ctrl Pts',(-201.94133416535,-94.0742581918852,15.0411941054338));
#20000=CARTESIAN_POINT('Ctrl Pts',(-204.121617554176,-91.9273998656518,
15.2001024242381));
#20001=CARTESIAN_POINT('Ctrl Pts',(-207.107193051684,-92.5974626419489,
15.3590107430424));
#20002=CARTESIAN_POINT('Ctrl Pts',(-208.160915650643,-95.4701538272465,
15.5179190618468));
#20003=CARTESIAN_POINT('Ctrl Pts',(-206.316749956396,-97.9117946067699,
15.676827380651));
#20004=CARTESIAN_POINT('Ctrl Pts',(-203.265394666789,-97.6839731562328,
15.8357356994554));
#20005=CARTESIAN_POINT('Ctrl Pts',(-201.804322600784,-94.995435472909,15.9946440182597));
#20006=CARTESIAN_POINT('Ctrl Pts',(-203.272977864808,-92.3112471546551,
16.153552337064));
#20007=CARTESIAN_POINT('Ctrl Pts',(-206.325018001399,-92.091736968933,16.3124606558683));
#20008=CARTESIAN_POINT('Ctrl Pts',(-208.162151193701,-94.5391937157227,
16.4713689746726));
#20009=CARTESIAN_POINT('Ctrl Pts',(-207.100560416909,-97.4076576435095,
16.6302772934769));
#20010=CARTESIAN_POINT('Ctrl Pts',(-204.112588629499,-98.0718310085313,
16.7891856122812));
#20011=CARTESIAN_POINT('Ctrl Pts',(-201.939550932507,-95.9135761483203,
16.9480939310855));
#20012=CARTESIAN_POINT('Ctrl Pts',(-202.36110058667,-93.9272907410154,17.0540328102884));
#20013=CARTESIAN_POINT('Ctrl Pts',(-202.945668449658,-93.2435746787732,
17.1070022498898));
#20014=CARTESIAN_POINT('Ctrl Pts',(-204.349800002025,-97.4320868020351,
-0.321006749669434));
#20015=CARTESIAN_POINT('Ctrl Pts',(-203.540360643981,-97.2156893163364,
-0.268037310067998));
#20016=CARTESIAN_POINT('Ctrl Pts',(-202.168816594393,-95.9134398742047,
-0.162098430865127));
#20017=CARTESIAN_POINT('Ctrl Pts',(-202.698129124083,-93.1102819915483,
-0.00319011206082018));
#20018=CARTESIAN_POINT('Ctrl Pts',(-205.342094399406,-92.0436412781577,
0.155718206743486));
#20019=CARTESIAN_POINT('Ctrl Pts',(-207.67036761967,-93.685358926356,0.314626525547793));
#20020=CARTESIAN_POINT('Ctrl Pts',(-207.551476213497,-96.5332828094945,
0.4735348443521));
#20021=CARTESIAN_POINT('Ctrl Pts',(-205.092937065996,-97.9750464823464,
0.632443163156407));
#20022=CARTESIAN_POINT('Ctrl Pts',(-202.549427810949,-96.6895450185623,
0.791351481960713));
#20023=CARTESIAN_POINT('Ctrl Pts',(-202.252462783667,-93.8549791096304,
0.95025980076502));
#20024=CARTESIAN_POINT('Ctrl Pts',(-204.474463806834,-92.0702080129899,
1.10916811956933));
#20025=CARTESIAN_POINT('Ctrl Pts',(-207.178244110245,-92.971412091657,1.26807643837363));
#20026=CARTESIAN_POINT('Ctrl Pts',(-207.885047341772,-95.7324151638398,
1.42698475717794));
#20027=CARTESIAN_POINT('Ctrl Pts',(-205.946865233257,-97.8219422640298,
1.58589307598225));
#20028=CARTESIAN_POINT('Ctrl Pts',(-203.140610652246,-97.3243471078651,
1.74480139478655));
#20029=CARTESIAN_POINT('Ctrl Pts',(-202.039021996833,-94.6958151132924,
1.90370971359086));
#20030=CARTESIAN_POINT('Ctrl Pts',(-203.652025580085,-92.3461570947101,
2.06261803239517));
#20031=CARTESIAN_POINT('Ctrl Pts',(-206.500836707101,-92.4295122653719,
2.22152635119947));
#20032=CARTESIAN_POINT('Ctrl Pts',(-207.973697679257,-94.8694620184648,
2.38043467000378));
#20033=CARTESIAN_POINT('Ctrl Pts',(-206.720305776311,-97.4290874580306,
2.53934298880809));
#20034=CARTESIAN_POINT('Ctrl Pts',(-203.889756803435,-97.7617527022432,
2.69825130761239));
#20035=CARTESIAN_POINT('Ctrl Pts',(-202.07706636569,-95.5624739187976,2.8571596264167));
#20036=CARTESIAN_POINT('Ctrl Pts',(-202.944088823814,-92.8475253418532,
3.01606794522101));
#20037=CARTESIAN_POINT('Ctrl Pts',(-205.695947665438,-92.1059414695739,
3.17497626402532));
#20038=CARTESIAN_POINT('Ctrl Pts',(-207.809769467947,-94.0175981137072,
3.33388458282962));
#20039=CARTESIAN_POINT('Ctrl Pts',(-207.347626025441,-96.829909826118,3.49279290163393));
#20040=CARTESIAN_POINT('Ctrl Pts',(-204.733205282231,-97.9645806629382,
3.65170122043823));
#20041=CARTESIAN_POINT('Ctrl Pts',(-202.363378954125,-96.3813570822541,
3.81060953924254));
#20042=CARTESIAN_POINT('Ctrl Pts',(-202.410777332023,-93.5317207678121,
3.96951785804685));
#20043=CARTESIAN_POINT('Ctrl Pts',(-204.831946112661,-92.0281864427333,
4.12842617685115));
#20044=CARTESIAN_POINT('Ctrl Pts',(-207.407184818934,-93.2491775716366,
4.28733449565546));
#20045=CARTESIAN_POINT('Ctrl Pts',(-207.775543387802,-96.0753031342707,
4.44624281445976));
#20046=CARTESIAN_POINT('Ctrl Pts',(-205.599314800415,-97.9156028018523,
4.60515113326408));
#20047=CARTESIAN_POINT('Ctrl Pts',(-202.873641102421,-97.0829104077825,
4.76405945206838));
#20048=CARTESIAN_POINT('Ctrl Pts',(-202.097389475856,-94.340629032118,4.92296777087269));
#20049=CARTESIAN_POINT('Ctrl Pts',(-203.982218735947,-92.2028515901542,
5.08187608967699));
#20050=CARTESIAN_POINT('Ctrl Pts',(-206.800138483392,-92.6294685471878,
5.2407844084813));
#20051=CARTESIAN_POINT('Ctrl Pts',(-207.967711389038,-95.2293622452196,
5.39969272728561));
#20052=CARTESIAN_POINT('Ctrl Pts',(-206.414519662711,-97.6189792003685,
5.55860104608991));
#20053=CARTESIAN_POINT('Ctrl Pts',(-203.564512119404,-97.6075452964086,
5.71750936489422));
#20054=CARTESIAN_POINT('Ctrl Pts',(-202.030543820876,-95.2055430086959,
5.87641768369853));
#20055=CARTESIAN_POINT('Ctrl Pts',(-203.218939758371,-92.6151011879226,
6.03532600250283));
#20056=CARTESIAN_POINT('Ctrl Pts',(-206.040191818849,-92.2111079425408,
6.19423432130715));
#20057=CARTESIAN_POINT('Ctrl Pts',(-207.907807645815,-94.3639397645677,
6.35314264011144));
#20058=CARTESIAN_POINT('Ctrl Pts',(-207.109577923063,-97.0999045013251,
6.51205095891576));
#20059=CARTESIAN_POINT('Ctrl Pts',(-204.377310738763,-97.9107002614662,
6.67095927772006));
#20060=CARTESIAN_POINT('Ctrl Pts',(-202.215918109496,-96.05299855419,6.82986759652437));
#20061=CARTESIAN_POINT('Ctrl Pts',(-202.606940640336,-93.2299195415795,
6.98877591532867));
#20062=CARTESIAN_POINT('Ctrl Pts',(-205.191893245386,-92.0296305094257,
7.14768423413299));
#20063=CARTESIAN_POINT('Ctrl Pts',(-207.600920267818,-93.5525430270246,
7.30659255293729));
#20064=CARTESIAN_POINT('Ctrl Pts',(-207.625452658662,-96.4024679195202,
7.4655008717416));
#20065=CARTESIAN_POINT('Ctrl Pts',(-205.242999396187,-97.9666258984934,
7.6244091905459));
#20066=CARTESIAN_POINT('Ctrl Pts',(-202.637767003241,-96.8110144110925,
7.78331750935021));
#20067=CARTESIAN_POINT('Ctrl Pts',(-202.198203419534,-93.9950851529353,
7.94222582815451));
#20068=CARTESIAN_POINT('Ctrl Pts',(-204.327295625697,-92.1004505948418,
8.10113414695882));
#20069=CARTESIAN_POINT('Ctrl Pts',(-207.073115683543,-92.8640905237329,
8.26004246576312));
#20070=CARTESIAN_POINT('Ctrl Pts',(-207.918326453502,-95.5859083878473,
8.41895078456744));
#20071=CARTESIAN_POINT('Ctrl Pts',(-206.088048148422,-97.7705719905599,
8.57785910337173));
#20072=CARTESIAN_POINT('Ctrl Pts',(-203.260259461758,-97.4152061584378,
8.73676742217605));
#20073=CARTESIAN_POINT('Ctrl Pts',(-202.027445455834,-94.8456063145195,
8.89567574098035));
#20074=CARTESIAN_POINT('Ctrl Pts',(-203.519836232374,-92.4175528758237,
9.05458405978466));
#20075=CARTESIAN_POINT('Ctrl Pts',(-206.369224607589,-92.3570580970949,
9.21349237858896));
#20076=CARTESIAN_POINT('Ctrl Pts',(-207.963323166107,-94.7195829153344,
9.37240069739328));
#20077=CARTESIAN_POINT('Ctrl Pts',(-206.840680166388,-97.3391909826315,
9.53130901619757));
#20078=CARTESIAN_POINT('Ctrl Pts',(-204.030522163026,-97.814254901706,9.6902173350019));
#20079=CARTESIAN_POINT('Ctrl Pts',(-202.109170604948,-95.7092413812417,
9.84912565380619));
#20080=CARTESIAN_POINT('Ctrl Pts',(-202.838099126052,-92.9540032894992,
10.0080339726105));
#20081=CARTESIAN_POINT('Ctrl Pts',(-205.549034205271,-92.0745121142617,
10.1669422914148));
#20082=CARTESIAN_POINT('Ctrl Pts',(-207.75662086154,-93.8770755350957,10.3258506102191));
#20083=CARTESIAN_POINT('Ctrl Pts',(-207.436968322131,-96.7091235546594,
10.4847589290234));
#20084=CARTESIAN_POINT('Ctrl Pts',(-204.883130462482,-97.974266201832,10.6436672478277));
#20085=CARTESIAN_POINT('Ctrl Pts',(-202.436437288604,-96.5126348379233,
10.802575566632));
#20086=CARTESIAN_POINT('Ctrl Pts',(-202.339989756123,-93.6642367610134,
10.9614838854363));
#20087=CARTESIAN_POINT('Ctrl Pts',(-204.682209884844,-92.0404514920568,
11.1203922042406));
#20088=CARTESIAN_POINT('Ctrl Pts',(-207.315776439265,-93.1299472169208,
11.279300523045));
#20089=CARTESIAN_POINT('Ctrl Pts',(-207.826265037123,-95.9338864321184,
11.4382088418493));
#20090=CARTESIAN_POINT('Ctrl Pts',(-205.745665437526,-97.8816490042056,
11.5971171606536));
#20091=CARTESIAN_POINT('Ctrl Pts',(-202.981448098954,-97.1875479768318,
11.7560254794579));
#20092=CARTESIAN_POINT('Ctrl Pts',(-202.067816582323,-94.4879274140711,
11.9149337982622));
#20093=CARTESIAN_POINT('Ctrl Pts',(-203.842378050611,-92.2577692747585,
12.0738421170665));
#20094=CARTESIAN_POINT('Ctrl Pts',(-206.678234383597,-92.5416576150057,
12.2327504358708));
#20095=CARTESIAN_POINT('Ctrl Pts',(-207.975504190982,-95.0793267774225,
12.3916587546751));
#20096=CARTESIAN_POINT('Ctrl Pts',(-206.544865012666,-97.544270036935,12.5505670734794));
#20097=CARTESIAN_POINT('Ctrl Pts',(-203.697910857383,-97.6766549633293,
12.7094753922837));
#20098=CARTESIAN_POINT('Ctrl Pts',(-202.044697474854,-95.3551125358376,
12.868383711088));
#20099=CARTESIAN_POINT('Ctrl Pts',(-203.100872416607,-92.7080069043539,
13.0272920298923));
#20100=CARTESIAN_POINT('Ctrl Pts',(-205.898146300591,-92.1621749261473,
13.1862003486966));
#20101=CARTESIAN_POINT('Ctrl Pts',(-207.872009694727,-94.2180292571993,
13.3451086675009));
#20102=CARTESIAN_POINT('Ctrl Pts',(-207.212846700311,-96.9907856267017,
13.5040169863053));
#20103=CARTESIAN_POINT('Ctrl Pts',(-204.524970584168,-97.9384119813983,
13.6629253051096));
#20104=CARTESIAN_POINT('Ctrl Pts',(-202.272596125939,-96.1921350794542,
13.8218336239139));
#20105=CARTESIAN_POINT('Ctrl Pts',(-202.520675058331,-93.3529220487526,
13.9807419427182));
#20106=CARTESIAN_POINT('Ctrl Pts',(-205.041771381152,-92.0237316998481,
14.1396502615225));
#20107=CARTESIAN_POINT('Ctrl Pts',(-207.524572179335,-93.423150811404,14.2985585803268));
#20108=CARTESIAN_POINT('Ctrl Pts',(-207.692873397937,-96.2682077424223,
14.4574668991311));
#20109=CARTESIAN_POINT('Ctrl Pts',(-205.392378428873,-97.9505857674807,
14.6163752179354));
#20110=CARTESIAN_POINT('Ctrl Pts',(-202.73215520691,-96.9279001984011,14.7752835367397));
#20111=CARTESIAN_POINT('Ctrl Pts',(-202.151066940101,-94.1377363253639,
14.934191855544));
#20112=CARTESIAN_POINT('Ctrl Pts',(-204.181848255277,-92.1380881155991,
15.0931001743483));
#20113=CARTESIAN_POINT('Ctrl Pts',(-206.962702783849,-92.7622046745167,
15.2520084931526));
#20114=CARTESIAN_POINT('Ctrl Pts',(-207.944171604055,-95.4379153703248,
15.4109168119569));
#20115=CARTESIAN_POINT('Ctrl Pts',(-206.226460386715,-97.7121327949226,
15.5698251307612));
#20116=CARTESIAN_POINT('Ctrl Pts',(-203.384336587646,-97.4999330656037,
15.7287334495655));
#20117=CARTESIAN_POINT('Ctrl Pts',(-202.023450261136,-94.9957484626189,
15.8876417683698));
#20118=CARTESIAN_POINT('Ctrl Pts',(-203.391399805631,-92.4956149886579,
16.0465500871742));
#20119=CARTESIAN_POINT('Ctrl Pts',(-206.234161491715,-92.2911566205669,
16.2054584059785));
#20120=CARTESIAN_POINT('Ctrl Pts',(-207.945322425902,-94.5707912114442,
16.3643667247828));
#20121=CARTESIAN_POINT('Ctrl Pts',(-206.956524948968,-97.24256451287,16.5232750435871));
#20122=CARTESIAN_POINT('Ctrl Pts',(-204.173438444138,-97.8611954975559,
16.6821833623914));
#20123=CARTESIAN_POINT('Ctrl Pts',(-202.149405983567,-95.8509322143663,
16.8410916811957));
#20124=CARTESIAN_POINT('Ctrl Pts',(-202.542049969887,-94.0008464354096,
16.9470305603986));
#20125=CARTESIAN_POINT('Ctrl Pts',(-203.086534003335,-93.3640127966251,
17.));
#20126=CARTESIAN_POINT('Ctrl Pts',(-202.485813979692,-94.9986458132734,
0.887416697508031));
#20127=CARTESIAN_POINT('Ctrl Pts',(-202.484186104837,-94.6662414532709,
0.908364398593701));
#20128=CARTESIAN_POINT('Ctrl Pts',(-202.545408874051,-94.3344113220432,
0.92931209967937));
#20129=CARTESIAN_POINT('Ctrl Pts',(-202.672290458742,-94.029944911679,0.95025980076504));
#20130=CARTESIAN_POINT('Ctrl Pts',(-202.993129791389,-93.2600554107502,
1.00322924036648));
#20131=CARTESIAN_POINT('Ctrl Pts',(-203.733796799112,-92.6651317118701,
1.05619867996791));
#20132=CARTESIAN_POINT('Ctrl Pts',(-204.554760353541,-92.5178705422078,
1.10916811956935));
#20133=CARTESIAN_POINT('Ctrl Pts',(-205.375723907971,-92.3706093725456,
1.16213755917078));
#20134=CARTESIAN_POINT('Ctrl Pts',(-206.276984009108,-92.6710107321013,
1.21510699877222));
#20135=CARTESIAN_POINT('Ctrl Pts',(-206.845414598264,-93.2813785905763,
1.26807643837365));
#20136=CARTESIAN_POINT('Ctrl Pts',(-207.41384518742,-93.8917464490512,1.32104587797509));
#20137=CARTESIAN_POINT('Ctrl Pts',(-207.649446264596,-94.8120808064455,
1.37401531757652));
#20138=CARTESIAN_POINT('Ctrl Pts',(-207.444216451765,-95.620502501841,1.42698475717796));
#20139=CARTESIAN_POINT('Ctrl Pts',(-207.238986638933,-96.4289241972365,
1.4799541967794));
#20140=CARTESIAN_POINT('Ctrl Pts',(-206.592925936095,-97.1254332306331,
1.53292363638083));
#20141=CARTESIAN_POINT('Ctrl Pts',(-205.802186487841,-97.390755221304,1.58589307598227));
#20142=CARTESIAN_POINT('Ctrl Pts',(-205.011447039586,-97.6560772119749,
1.6388625155837));
#20143=CARTESIAN_POINT('Ctrl Pts',(-204.076028845916,-97.49021215992,1.69183195518514));
#20144=CARTESIAN_POINT('Ctrl Pts',(-203.424721639845,-96.9691909681305,
1.74480139478657));
#20145=CARTESIAN_POINT('Ctrl Pts',(-202.840193560653,-96.501590558344,1.79233982902706));
#20146=CARTESIAN_POINT('Ctrl Pts',(-202.484502889507,-95.7479293694392,
1.83987826326755));
#20147=CARTESIAN_POINT('Ctrl Pts',(-202.479323384637,-94.9985362448309,
1.88741669750803));
#20148=CARTESIAN_POINT('Ctrl Pts',(-204.206200717467,-97.9692229537457,
-1.94289029309402E-15));
#20149=CARTESIAN_POINT('Ctrl Pts',(-204.113164566746,-97.9351899142219,
-1.95608846886529E-15));
#20150=CARTESIAN_POINT('Ctrl Pts',(-204.022195793433,-97.8963847243652,
-1.87178471689281E-15));
#20151=CARTESIAN_POINT('Ctrl Pts',(-203.933501803929,-97.8531368677882,
-1.96197225132977E-15));
#20152=CARTESIAN_POINT('Ctrl Pts',(-203.842828758516,-97.808924008661,-2.05417216759616E-15));
#20153=CARTESIAN_POINT('Ctrl Pts',(-203.754532478722,-97.7600673920919,
-2.02940294614423E-15));
#20154=CARTESIAN_POINT('Ctrl Pts',(-203.668863497467,-97.706873479352,-1.98105420956551E-15));
#20155=CARTESIAN_POINT('Ctrl Pts',(-203.585835066753,-97.6553191473921,
-1.93419571228578E-15));
#20156=CARTESIAN_POINT('Ctrl Pts',(-203.505274137607,-97.5996899115334,
-2.24355396026084E-15));
#20157=CARTESIAN_POINT('Ctrl Pts',(-203.427442606602,-97.5402339590788,
-2.26207941267376E-15));
#20158=CARTESIAN_POINT('Ctrl Pts',(-203.359340016973,-97.4882100006811,
-2.27828918353506E-15));
#20159=CARTESIAN_POINT('Ctrl Pts',(-203.29332742065,-97.4332554915952,-1.79029168246463E-15));
#20160=CARTESIAN_POINT('Ctrl Pts',(-203.2296056295,-97.3755236839992,-1.74166236988071E-15));
#20161=CARTESIAN_POINT('Ctrl Pts',(-203.216356113094,-97.3635196502445,
-1.73155099568283E-15));
#20162=CARTESIAN_POINT('Ctrl Pts',(-203.203203983489,-97.3513937509761,
-1.77457247924768E-15));
#20163=CARTESIAN_POINT('Ctrl Pts',(-203.190167931591,-97.3391634026804,
-1.77635683940025E-15));
#20164=CARTESIAN_POINT('Ctrl Pts',(-203.117744760303,-97.2712164033532,
-1.78627004180089E-15));
#20165=CARTESIAN_POINT('Ctrl Pts',(-203.048787400483,-97.1999474448534,
-1.60673788718679E-15));
#20166=CARTESIAN_POINT('Ctrl Pts',(-202.983534963279,-97.1256486442048,
-1.63757896132211E-15));
#20167=CARTESIAN_POINT('Ctrl Pts',(-202.918640645489,-97.0517576113602,
-1.66825077300687E-15));
#20168=CARTESIAN_POINT('Ctrl Pts',(-202.857410209928,-96.97486910218,-1.76356714015849E-15));
#20169=CARTESIAN_POINT('Ctrl Pts',(-202.800122474302,-96.8952437100093,
-1.72084568816899E-15));
#20170=CARTESIAN_POINT('Ctrl Pts',(-202.744171289059,-96.8174760164764,
-1.67912094817054E-15));
#20171=CARTESIAN_POINT('Ctrl Pts',(-202.691980694321,-96.7370969139694,
-2.11654729638491E-15));
#20172=CARTESIAN_POINT('Ctrl Pts',(-202.643857601275,-96.6543350073822,
-2.27595720048157E-15));
#20173=CARTESIAN_POINT('Ctrl Pts',(-202.62307823217,-96.6185987299325,-2.34478979262376E-15));
#20174=CARTESIAN_POINT('Ctrl Pts',(-202.603057870683,-96.5824180660604,
-2.21214957918682E-15));
#20175=CARTESIAN_POINT('Ctrl Pts',(-202.583824240712,-96.5458110879139,
-2.23432383705813E-15));
#20176=CARTESIAN_POINT('Ctrl Pts',(-202.569909304535,-96.5193270718798,
-2.25036622653533E-15));
#20177=CARTESIAN_POINT('Ctrl Pts',(-202.55640618783,-96.4926199163307,-1.6439290738235E-15));
#20178=CARTESIAN_POINT('Ctrl Pts',(-202.543326026024,-96.4656964618893,
-1.63757896132211E-15));
#20179=CARTESIAN_POINT('Ctrl Pts',(-202.537164434797,-96.4530137960989,
-1.63458765295335E-15));
#20180=CARTESIAN_POINT('Ctrl Pts',(-202.531098886162,-96.4402875329931,
-2.24077876564333E-15));
#20181=CARTESIAN_POINT('Ctrl Pts',(-202.525133543247,-96.4275255114806,
-2.23432383705813E-15));
#20182=CARTESIAN_POINT('Ctrl Pts',(-202.485117270381,-96.3419162611141,
-2.19102336175286E-15));
#20183=CARTESIAN_POINT('Ctrl Pts',(-202.4495592445,-96.254603019968,-1.8759278374734E-15));
#20184=CARTESIAN_POINT('Ctrl Pts',(-202.418711175416,-96.1658234873367,
-1.80411241501588E-15));
#20185=CARTESIAN_POINT('Ctrl Pts',(-202.388547336981,-96.0790131436709,
-1.73388990629946E-15));
#20186=CARTESIAN_POINT('Ctrl Pts',(-202.362886617194,-95.990800160075,-1.72432441326592E-15));
#20187=CARTESIAN_POINT('Ctrl Pts',(-202.342013530391,-95.9013982186672,
-1.63757896132211E-15));
#20188=CARTESIAN_POINT('Ctrl Pts',(-202.338634312827,-95.886924623388,-1.62353543448175E-15));
#20189=CARTESIAN_POINT('Ctrl Pts',(-202.335380687559,-95.8724198597991,
-2.0203055504241E-15));
#20190=CARTESIAN_POINT('Ctrl Pts',(-202.332253992484,-95.8578848308905,
-2.02615701994091E-15));
#20191=CARTESIAN_POINT('Ctrl Pts',(-202.312215595091,-95.7647325795669,
-2.03483094975162E-15));
#20192=CARTESIAN_POINT('Ctrl Pts',(-202.297386480098,-95.670336192193,-1.24180755483495E-15));
#20193=CARTESIAN_POINT('Ctrl Pts',(-202.287688067001,-95.5751039661889,
-1.16573417585641E-15));
#20194=CARTESIAN_POINT('Ctrl Pts',(-202.284332121912,-95.5421507275438,
-1.13941047938093E-15));
#20195=CARTESIAN_POINT('Ctrl Pts',(-202.281590951551,-95.5090975364209,
-1.59096596101214E-15));
#20196=CARTESIAN_POINT('Ctrl Pts',(-202.27946265438,-95.4759618339203,-1.58206781009085E-15));
#20197=CARTESIAN_POINT('Ctrl Pts',(-202.278435478218,-95.459969610567,-1.57777331182387E-15));
#20198=CARTESIAN_POINT('Ctrl Pts',(-202.277551068544,-95.4439581729582,
-1.39634750300735E-15));
#20199=CARTESIAN_POINT('Ctrl Pts',(-202.276809266428,-95.4279295130754,
-1.36002320516582E-15));
#20200=CARTESIAN_POINT('Ctrl Pts',(-202.276232614801,-95.4154693803712,
-1.33178593674769E-15));
#20201=CARTESIAN_POINT('Ctrl Pts',(-202.27574223997,-95.402999988249,-2.11721333807556E-15));
#20202=CARTESIAN_POINT('Ctrl Pts',(-202.275338217547,-95.3905321636395,
-2.1094237467878E-15));
#20203=CARTESIAN_POINT('Ctrl Pts',(-202.272318895462,-95.2973581810847,
-2.05121092574771E-15));
#20204=CARTESIAN_POINT('Ctrl Pts',(-202.274110299127,-95.2041209575845,
-1.64901362259784E-15));
#20205=CARTESIAN_POINT('Ctrl Pts',(-202.280572742583,-95.111194847899,-1.63757896132211E-15));
#20206=CARTESIAN_POINT('Ctrl Pts',(-202.287048682582,-95.0180746659159,
-1.62612041923403E-15));
#20207=CARTESIAN_POINT('Ctrl Pts',(-202.29821557696,-94.9252659180417,-1.50579107067496E-15));
#20208=CARTESIAN_POINT('Ctrl Pts',(-202.313983936443,-94.8331572852858,
-1.4432899320127E-15));
#20209=CARTESIAN_POINT('Ctrl Pts',(-202.329531074206,-94.7423408877986,
-1.38166565117914E-15));
#20210=CARTESIAN_POINT('Ctrl Pts',(-202.349551938789,-94.6522042518842,
-1.95220788294063E-15));
#20211=CARTESIAN_POINT('Ctrl Pts',(-202.374003831615,-94.5631450482855,
-2.02615701994091E-15));
#20212=CARTESIAN_POINT('Ctrl Pts',(-202.383516776035,-94.5284967999894,
-2.0549267366747E-15));
#20213=CARTESIAN_POINT('Ctrl Pts',(-202.393700820255,-94.4940119683205,
-2.105212970477E-15));
#20214=CARTESIAN_POINT('Ctrl Pts',(-202.40455502065,-94.4597154343389,-2.13717932240343E-15));
#20215=CARTESIAN_POINT('Ctrl Pts',(-202.410353854707,-94.4413925821662,
-2.15425727964432E-15));
#20216=CARTESIAN_POINT('Ctrl Pts',(-202.416343979603,-94.4231234896604,
-1.92388717056435E-15));
#20217=CARTESIAN_POINT('Ctrl Pts',(-202.422525347087,-94.4049120649473,
-1.9151347174784E-15));
#20218=CARTESIAN_POINT('Ctrl Pts',(-202.428042996055,-94.3886560748213,
-1.90732205080426E-15));
#20219=CARTESIAN_POINT('Ctrl Pts',(-202.433713565198,-94.3724447894493,
-2.11171038093633E-15));
#20220=CARTESIAN_POINT('Ctrl Pts',(-202.43953069679,-94.3562979493254,-2.1094237467878E-15));
#20221=CARTESIAN_POINT('Ctrl Pts',(-202.470363841107,-94.2707131823399,
-2.09730366327417E-15));
#20222=CARTESIAN_POINT('Ctrl Pts',(-202.505347374394,-94.1868267447458,
-2.98179513899234E-15));
#20223=CARTESIAN_POINT('Ctrl Pts',(-202.544417035463,-94.1050192581487,
-2.4980018054066E-15));
#20224=CARTESIAN_POINT('Ctrl Pts',(-202.5758795135,-94.0391403592833,-2.10840699665774E-15));
#20225=CARTESIAN_POINT('Ctrl Pts',(-202.609992739017,-93.9746099539844,
-1.67224799697884E-15));
#20226=CARTESIAN_POINT('Ctrl Pts',(-202.646741355094,-93.9116445196917,
-1.77635683940025E-15));
#20227=CARTESIAN_POINT('Ctrl Pts',(-202.661983680304,-93.8855281722226,
-1.81953835214335E-15));
#20228=CARTESIAN_POINT('Ctrl Pts',(-202.677679568848,-93.8596812729456,
-2.49009010979644E-15));
#20229=CARTESIAN_POINT('Ctrl Pts',(-202.693828658099,-93.8341202619796,
-2.55351295663786E-15));
#20230=CARTESIAN_POINT('Ctrl Pts',(-202.702295534382,-93.8207187683019,
-2.58676519701672E-15));
#20231=CARTESIAN_POINT('Ctrl Pts',(-202.710885570826,-93.8073982241056,
-2.09795412669662E-15));
#20232=CARTESIAN_POINT('Ctrl Pts',(-202.719593908756,-93.7941678734082,
-2.05391259555654E-15));
#20233=CARTESIAN_POINT('Ctrl Pts',(-202.767002638161,-93.7221410272768,
-1.81414778059626E-15));
#20234=CARTESIAN_POINT('Ctrl Pts',(-202.817953827573,-93.6527223685765,
-9.92560611046316E-16));
#20235=CARTESIAN_POINT('Ctrl Pts',(-202.872410768078,-93.5862671725324,
-6.66133814775094E-16));
#20236=CARTESIAN_POINT('Ctrl Pts',(-202.926867708583,-93.5198119764882,
-3.3970701850387E-16));
#20237=CARTESIAN_POINT('Ctrl Pts',(-202.984830731065,-93.4563195512772,
-4.53570776702435E-17));
#20238=CARTESIAN_POINT('Ctrl Pts',(-203.046292621091,-93.3961891673829,
3.33066907387547E-16));
#20239=CARTESIAN_POINT('Ctrl Pts',(-203.058343397196,-93.3843994584574,
4.07452946255978E-16));
#20240=CARTESIAN_POINT('Ctrl Pts',(-203.070528764207,-93.3727391521122,
-1.78805262136535E-16));
#20241=CARTESIAN_POINT('Ctrl Pts',(-203.082846138209,-93.3612093103597,
-1.66533453693773E-16));
#20242=CARTESIAN_POINT('Origin',(-205.,-95.,9.));
#20243=CARTESIAN_POINT('Origin',(-205.,95.,17.));
#20244=CARTESIAN_POINT('Ctrl Pts',(-203.086534003335,96.6359872033749,17.));
#20245=CARTESIAN_POINT('Ctrl Pts',(-203.024407982535,96.5776039990143,17.));
#20246=CARTESIAN_POINT('Ctrl Pts',(-202.965660663619,96.5159659235685,17.));
#20247=CARTESIAN_POINT('Ctrl Pts',(-202.910302607292,96.4514497134767,17.));
#20248=CARTESIAN_POINT('Ctrl Pts',(-202.853587227097,96.3853516307974,17.));
#20249=CARTESIAN_POINT('Ctrl Pts',(-202.800428883688,96.3162320542646,17.));
#20250=CARTESIAN_POINT('Ctrl Pts',(-202.750867872641,96.2444498370416,17.));
#20251=CARTESIAN_POINT('Ctrl Pts',(-202.73795912874,96.2257533205829,17.));
#20252=CARTESIAN_POINT('Ctrl Pts',(-202.725294599279,96.2068759539151,17.));
#20253=CARTESIAN_POINT('Ctrl Pts',(-202.712875369652,96.1878236473054,17.));
#20254=CARTESIAN_POINT('Ctrl Pts',(-202.702666789577,96.1721626921996,17.));
#20255=CARTESIAN_POINT('Ctrl Pts',(-202.692623482104,96.1563825746979,17.));
#20256=CARTESIAN_POINT('Ctrl Pts',(-202.682754989924,96.1405013265158,17.));
#20257=CARTESIAN_POINT('Ctrl Pts',(-202.635325886293,96.0641742289145,17.));
#20258=CARTESIAN_POINT('Ctrl Pts',(-202.591881571366,95.9854386369538,17.));
#20259=CARTESIAN_POINT('Ctrl Pts',(-202.55245519555,95.9046876041234,17.));
#20260=CARTESIAN_POINT('Ctrl Pts',(-202.520329458461,95.8388893562068,17.));
#20261=CARTESIAN_POINT('Ctrl Pts',(-202.490871898904,95.7717518764231,17.));
#20262=CARTESIAN_POINT('Ctrl Pts',(-202.464118215874,95.7034693999465,17.));
#20263=CARTESIAN_POINT('Ctrl Pts',(-202.455239378807,95.6808082589538,17.));
#20264=CARTESIAN_POINT('Ctrl Pts',(-202.446658487047,95.6580208940291,17.));
#20265=CARTESIAN_POINT('Ctrl Pts',(-202.438377277411,95.6351140931728,17.));
#20266=CARTESIAN_POINT('Ctrl Pts',(-202.431690505786,95.6166176955754,17.));
#20267=CARTESIAN_POINT('Ctrl Pts',(-202.425198327662,95.5980406868312,17.));
#20268=CARTESIAN_POINT('Ctrl Pts',(-202.418909348376,95.5794101202441,17.));
#20269=CARTESIAN_POINT('Ctrl Pts',(-202.389394173141,95.4919739223399,17.));
#20270=CARTESIAN_POINT('Ctrl Pts',(-202.364312526072,95.4032571051593,17.));
#20271=CARTESIAN_POINT('Ctrl Pts',(-202.343695486232,95.3136579957359,17.));
#20272=CARTESIAN_POINT('Ctrl Pts',(-202.322619877632,95.2220660031035,17.));
#20273=CARTESIAN_POINT('Ctrl Pts',(-202.306209135304,95.1295512442093,17.));
#20274=CARTESIAN_POINT('Ctrl Pts',(-202.294539294593,95.0365052928358,17.));
#20275=CARTESIAN_POINT('Ctrl Pts',(-202.28303676288,94.9447933292428,17.));
#20276=CARTESIAN_POINT('Ctrl Pts',(-202.276139875649,94.8525643337987,17.));
#20277=CARTESIAN_POINT('Ctrl Pts',(-202.273968539135,94.7601740929499,17.));
#20278=CARTESIAN_POINT('Ctrl Pts',(-202.272844064581,94.712327766861,17.));
#20279=CARTESIAN_POINT('Ctrl Pts',(-202.272987744046,94.6644379678861,17.));
#20280=CARTESIAN_POINT('Ctrl Pts',(-202.274421710976,94.6165533352961,17.));
#20281=CARTESIAN_POINT('Ctrl Pts',(-202.275071818331,94.5948442211265,17.));
#20282=CARTESIAN_POINT('Ctrl Pts',(-202.27598770662,94.5731290901658,17.));
#20283=CARTESIAN_POINT('Ctrl Pts',(-202.277169213423,94.5514506162179,17.));
#20284=CARTESIAN_POINT('Ctrl Pts',(-202.282380583036,94.4558315812025,17.));
#20285=CARTESIAN_POINT('Ctrl Pts',(-202.292755622429,94.3608204174972,17.));
#20286=CARTESIAN_POINT('Ctrl Pts',(-202.308361288381,94.2668143079404,17.));
#20287=CARTESIAN_POINT('Ctrl Pts',(-202.312210020092,94.2436301454694,17.));
#20288=CARTESIAN_POINT('Ctrl Pts',(-202.316377126191,94.2205070204909,17.));
#20289=CARTESIAN_POINT('Ctrl Pts',(-202.320864073854,94.1974507357616,17.));
#20290=CARTESIAN_POINT('Ctrl Pts',(-202.338369541768,94.1074984825093,17.));
#20291=CARTESIAN_POINT('Ctrl Pts',(-202.360739116816,94.018563693276,17.));
#20292=CARTESIAN_POINT('Ctrl Pts',(-202.38766964512,93.930876392274,17.));
#20293=CARTESIAN_POINT('Ctrl Pts',(-202.415202275748,93.8412286125482,17.));
#20294=CARTESIAN_POINT('Ctrl Pts',(-202.447502301944,93.752884024605,17.));
#20295=CARTESIAN_POINT('Ctrl Pts',(-202.48429995413,93.6660928701058,17.));
#20296=CARTESIAN_POINT('Ctrl Pts',(-202.498927308279,93.631592708318,17.));
#20297=CARTESIAN_POINT('Ctrl Pts',(-202.514265915705,93.5973381158404,17.));
#20298=CARTESIAN_POINT('Ctrl Pts',(-202.53030100434,93.5633453916794,17.));
#20299=CARTESIAN_POINT('Ctrl Pts',(-202.538297772879,93.5463930720939,17.));
#20300=CARTESIAN_POINT('Ctrl Pts',(-202.546469611153,93.5295024211424,17.));
#20301=CARTESIAN_POINT('Ctrl Pts',(-202.554802372669,93.5126998655829,17.));
#20302=CARTESIAN_POINT('Ctrl Pts',(-202.597596782594,93.4264072902949,17.));
#20303=CARTESIAN_POINT('Ctrl Pts',(-202.644686342007,93.3423163357714,17.));
#20304=CARTESIAN_POINT('Ctrl Pts',(-202.69572565248,93.2606735373991,17.));
#20305=CARTESIAN_POINT('Ctrl Pts',(-202.747781901769,93.1774040373738,17.));
#20306=CARTESIAN_POINT('Ctrl Pts',(-202.80394718269,93.0966804560165,17.));
#20307=CARTESIAN_POINT('Ctrl Pts',(-202.863910132442,93.0187715614717,17.));
#20308=CARTESIAN_POINT('Ctrl Pts',(-202.924370593286,92.9402162587798,17.));
#20309=CARTESIAN_POINT('Ctrl Pts',(-202.988692466357,92.8645217114623,17.));
#20310=CARTESIAN_POINT('Ctrl Pts',(-203.056605938085,92.7919828149226,17.));
#20311=CARTESIAN_POINT('Ctrl Pts',(-203.094650995819,92.7513465989163,17.));
#20312=CARTESIAN_POINT('Ctrl Pts',(-203.133824024131,92.7117011149777,17.));
#20313=CARTESIAN_POINT('Ctrl Pts',(-203.174083422688,92.673102348505,17.));
#20314=CARTESIAN_POINT('Ctrl Pts',(-203.185629619105,92.6620324131581,17.));
#20315=CARTESIAN_POINT('Ctrl Pts',(-203.1972651951,92.6510485939825,17.));
#20316=CARTESIAN_POINT('Ctrl Pts',(-203.208989225885,92.6401522676968,17.));
#20317=CARTESIAN_POINT('Ctrl Pts',(-203.219402166174,92.6304744702682,17.));
#20318=CARTESIAN_POINT('Ctrl Pts',(-203.229881653,92.6208687455018,17.));
#20319=CARTESIAN_POINT('Ctrl Pts',(-203.240420864849,92.6113412724527,17.));
#20320=CARTESIAN_POINT('Ctrl Pts',(-203.31613092934,92.5428991906971,17.));
#20321=CARTESIAN_POINT('Ctrl Pts',(-203.39501019773,92.4784087555357,17.));
#20322=CARTESIAN_POINT('Ctrl Pts',(-203.476728217726,92.4181490409495,17.));
#20323=CARTESIAN_POINT('Ctrl Pts',(-203.558538789846,92.3578210774687,17.));
#20324=CARTESIAN_POINT('Ctrl Pts',(-203.643195128873,92.3017325904328,17.));
#20325=CARTESIAN_POINT('Ctrl Pts',(-203.730410869524,92.2501895488276,17.));
#20326=CARTESIAN_POINT('Ctrl Pts',(-203.815807914422,92.1997213259438,17.));
#20327=CARTESIAN_POINT('Ctrl Pts',(-203.903659405823,92.1536102898009,17.));
#20328=CARTESIAN_POINT('Ctrl Pts',(-203.993730337174,92.1121794018575,17.));
#20329=CARTESIAN_POINT('Ctrl Pts',(-204.04409635998,92.08901200461,17.));
#20330=CARTESIAN_POINT('Ctrl Pts',(-204.095156919867,92.0673087145635,17.));
#20331=CARTESIAN_POINT('Ctrl Pts',(-204.146874522078,92.0471322125037,17.));
#20332=CARTESIAN_POINT('Ctrl Pts',(-204.165970757723,92.0396822298796,17.));
#20333=CARTESIAN_POINT('Ctrl Pts',(-204.185156595851,92.0324404568016,17.));
#20334=CARTESIAN_POINT('Ctrl Pts',(-204.204429069408,92.0254062069443,17.));
#20335=CARTESIAN_POINT('Ctrl Pts',(-205.793799282533,92.0307770462543,17.));
#20336=CARTESIAN_POINT('Ctrl Pts',(-205.888625439193,92.0654648779461,17.));
#20337=CARTESIAN_POINT('Ctrl Pts',(-205.981405837457,92.105147830213,17.));
#20338=CARTESIAN_POINT('Ctrl Pts',(-206.071900643333,92.1495042740275,17.));
#20339=CARTESIAN_POINT('Ctrl Pts',(-206.163682037882,92.1944913451757,17.));
#20340=CARTESIAN_POINT('Ctrl Pts',(-206.253113055814,92.2442864444201,17.));
#20341=CARTESIAN_POINT('Ctrl Pts',(-206.339909452525,92.2985947378519,17.));
#20342=CARTESIAN_POINT('Ctrl Pts',(-206.364289257077,92.3138491220152,17.));
#20343=CARTESIAN_POINT('Ctrl Pts',(-206.388460961959,92.3294597884703,17.));
#20344=CARTESIAN_POINT('Ctrl Pts',(-206.412417682282,92.3454206513343,17.));
#20345=CARTESIAN_POINT('Ctrl Pts',(-206.431857110393,92.3583719252173,17.));
#20346=CARTESIAN_POINT('Ctrl Pts',(-206.451157193771,92.3715554798855,17.));
#20347=CARTESIAN_POINT('Ctrl Pts',(-206.470294701023,92.3849541090983,17.));
#20348=CARTESIAN_POINT('Ctrl Pts',(-206.553006045271,92.4428623109673,17.));
#20349=CARTESIAN_POINT('Ctrl Pts',(-206.632761485621,92.5048354140007,17.));
#20350=CARTESIAN_POINT('Ctrl Pts',(-206.709295609939,92.5705745565257,17.));
#20351=CARTESIAN_POINT('Ctrl Pts',(-206.768823569185,92.6217062188,17.));
#20352=CARTESIAN_POINT('Ctrl Pts',(-206.826402117093,92.6751171275772,17.));
#20353=CARTESIAN_POINT('Ctrl Pts',(-206.881888242456,92.7306787828074,17.));
#20354=CARTESIAN_POINT('Ctrl Pts',(-206.912065039079,92.7608966572574,17.));
#20355=CARTESIAN_POINT('Ctrl Pts',(-206.941622633342,92.7917508510965,17.));
#20356=CARTESIAN_POINT('Ctrl Pts',(-206.970535764831,92.8232216127412,17.));
#20357=CARTESIAN_POINT('Ctrl Pts',(-206.98234105479,92.8360711882562,17.));
#20358=CARTESIAN_POINT('Ctrl Pts',(-206.994033802991,92.8490180878463,17.));
#20359=CARTESIAN_POINT('Ctrl Pts',(-207.00560763218,92.8620550677975,17.));
#20360=CARTESIAN_POINT('Ctrl Pts',(-207.071007128224,92.9357222962328,17.));
#20361=CARTESIAN_POINT('Ctrl Pts',(-207.132664441688,93.0123192022955,17.));
#20362=CARTESIAN_POINT('Ctrl Pts',(-207.190334457617,93.0915674062453,17.));
#20363=CARTESIAN_POINT('Ctrl Pts',(-207.247546914657,93.1701868480969,17.));
#20364=CARTESIAN_POINT('Ctrl Pts',(-207.30083553606,93.2514164669213,17.));
#20365=CARTESIAN_POINT('Ctrl Pts',(-207.349914694167,93.3350062931376,17.));
#20366=CARTESIAN_POINT('Ctrl Pts',(-207.397475463616,93.4160100553518,17.));
#20367=CARTESIAN_POINT('Ctrl Pts',(-207.441083386685,93.499230945498,17.));
#20368=CARTESIAN_POINT('Ctrl Pts',(-207.480430624137,93.5844511813323,17.));
#20369=CARTESIAN_POINT('Ctrl Pts',(-207.501046370163,93.6291018061788,17.));
#20370=CARTESIAN_POINT('Ctrl Pts',(-207.520491662325,93.6743013859238,17.));
#20371=CARTESIAN_POINT('Ctrl Pts',(-207.538716459085,93.7200187685398,17.));
#20372=CARTESIAN_POINT('Ctrl Pts',(-207.545013503871,93.7358150712166,17.));
#20373=CARTESIAN_POINT('Ctrl Pts',(-207.551164803887,93.7516731900739,17.));
#20374=CARTESIAN_POINT('Ctrl Pts',(-207.557168177544,93.7675918326183,17.));
#20375=CARTESIAN_POINT('Ctrl Pts',(-207.562729535398,93.7823384189236,17.));
#20376=CARTESIAN_POINT('Ctrl Pts',(-207.568161177558,93.7971297270081,17.));
#20377=CARTESIAN_POINT('Ctrl Pts',(-207.573459278408,93.8119574010363,17.));
#20378=CARTESIAN_POINT('Ctrl Pts',(-207.604693559378,93.8993720709009,17.));
#20379=CARTESIAN_POINT('Ctrl Pts',(-207.631320320326,93.9881282654993,17.));
#20380=CARTESIAN_POINT('Ctrl Pts',(-207.653087336967,94.07800225261,17.));
#20381=CARTESIAN_POINT('Ctrl Pts',(-207.658248256261,94.0993112083491,17.));
#20382=CARTESIAN_POINT('Ctrl Pts',(-207.663135756651,94.1206830429499,17.));
#20383=CARTESIAN_POINT('Ctrl Pts',(-207.667746045347,94.142114835567,17.));
#20384=CARTESIAN_POINT('Ctrl Pts',(-207.687556359468,94.2342068002817,17.));
#20385=CARTESIAN_POINT('Ctrl Pts',(-207.702252352955,94.3274062210526,17.));
#20386=CARTESIAN_POINT('Ctrl Pts',(-207.711945471377,94.4213210251117,17.));
#20387=CARTESIAN_POINT('Ctrl Pts',(-207.722114172796,94.5198436635245,17.));
#20388=CARTESIAN_POINT('Ctrl Pts',(-207.726777055298,94.6191548874199,17.));
#20389=CARTESIAN_POINT('Ctrl Pts',(-207.726004510103,94.7187860623211,17.));
#20390=CARTESIAN_POINT('Ctrl Pts',(-207.725764562221,94.7497309048235,17.));
#20391=CARTESIAN_POINT('Ctrl Pts',(-207.724999859398,94.7807064222678,17.));
#20392=CARTESIAN_POINT('Ctrl Pts',(-207.723711444567,94.8116979686419,17.));
#20393=CARTESIAN_POINT('Ctrl Pts',(-207.723122838063,94.8258563168052,17.));
#20394=CARTESIAN_POINT('Ctrl Pts',(-207.72242484411,94.8400180917865,17.));
#20395=CARTESIAN_POINT('Ctrl Pts',(-207.721618574493,94.8541673752309,17.));
#20396=CARTESIAN_POINT('Ctrl Pts',(-207.716327457255,94.9470215718848,17.));
#20397=CARTESIAN_POINT('Ctrl Pts',(-207.706371961745,95.0394947841683,17.));
#20398=CARTESIAN_POINT('Ctrl Pts',(-207.691879894166,95.131215897366,17.));
#20399=CARTESIAN_POINT('Ctrl Pts',(-207.67741843296,95.2227433010943,17.));
#20400=CARTESIAN_POINT('Ctrl Pts',(-207.658439124386,95.3135227252561,17.));
#20401=CARTESIAN_POINT('Ctrl Pts',(-207.635020244211,95.4031684384919,17.));
#20402=CARTESIAN_POINT('Ctrl Pts',(-207.611996292461,95.4913023953998,17.));
#20403=CARTESIAN_POINT('Ctrl Pts',(-207.584680766522,95.5783413425628,17.));
#20404=CARTESIAN_POINT('Ctrl Pts',(-207.553107669616,95.6638896101273,17.));
#20405=CARTESIAN_POINT('Ctrl Pts',(-207.536805015492,95.708062147942,17.));
#20406=CARTESIAN_POINT('Ctrl Pts',(-207.519366615784,95.7518366999759,17.));
#20407=CARTESIAN_POINT('Ctrl Pts',(-207.500793440028,95.7951546486274,17.));
#20408=CARTESIAN_POINT('Ctrl Pts',(-207.494983232573,95.8087057112732,17.));
#20409=CARTESIAN_POINT('Ctrl Pts',(-207.489061185403,95.8222137843736,17.));
#20410=CARTESIAN_POINT('Ctrl Pts',(-207.48302971481,95.8356715889093,17.));
#20411=CARTESIAN_POINT('Ctrl Pts',(-207.446486009935,95.9172102501051,17.));
#20412=CARTESIAN_POINT('Ctrl Pts',(-207.406052548468,95.9966328231811,17.));
#20413=CARTESIAN_POINT('Ctrl Pts',(-207.361809031731,96.0735940904104,17.));
#20414=CARTESIAN_POINT('Ctrl Pts',(-207.318276147011,96.1493192185477,17.));
#20415=CARTESIAN_POINT('Ctrl Pts',(-207.271054151283,96.2226621614719,17.));
#20416=CARTESIAN_POINT('Ctrl Pts',(-207.22018182407,96.2932611166533,17.));
#20417=CARTESIAN_POINT('Ctrl Pts',(-207.170938066514,96.3615999960239,17.));
#20418=CARTESIAN_POINT('Ctrl Pts',(-207.118273489373,96.4273682047813,17.));
#20419=CARTESIAN_POINT('Ctrl Pts',(-207.062195039505,96.4901984373505,17.));
#20420=CARTESIAN_POINT('Ctrl Pts',(-207.027351919219,96.5292366303853,17.));
#20421=CARTESIAN_POINT('Ctrl Pts',(-206.991190347134,96.5671398225301,17.));
#20422=CARTESIAN_POINT('Ctrl Pts',(-206.953707348215,96.6038107958082,17.));
#20423=CARTESIAN_POINT('Ctrl Pts',(-206.941658583283,96.615598538241,17.));
#20424=CARTESIAN_POINT('Ctrl Pts',(-206.929473251158,96.6272588980258,17.));
#20425=CARTESIAN_POINT('Ctrl Pts',(-206.917153830491,96.638790656604,17.));
#20426=CARTESIAN_POINT('Origin',(-205.,95.,-2.20842344717744));
#20427=CARTESIAN_POINT('Ctrl Pts',(-201.923720806533,95.0022768293025,0.291576552822547));
#20428=CARTESIAN_POINT('Ctrl Pts',(-201.922485619479,95.1502545480464,0.299259877064296));
#20429=CARTESIAN_POINT('Ctrl Pts',(-201.99954223613,96.317136758203,0.359912640907481));
#20430=CARTESIAN_POINT('Ctrl Pts',(-203.493269023741,98.307102300781,0.473534844352101));
#20431=CARTESIAN_POINT('Ctrl Pts',(-206.963865970602,98.0574884319591,0.632443163156409));
#20432=CARTESIAN_POINT('Ctrl Pts',(-208.633932648393,95.0051905167663,0.791351481960714));
#20433=CARTESIAN_POINT('Ctrl Pts',(-206.972489133437,91.9479467192658,0.950259800765022));
#20434=CARTESIAN_POINT('Ctrl Pts',(-203.50267093535,91.6888818401662,1.10916811956933));
#20435=CARTESIAN_POINT('Ctrl Pts',(-202.001246091317,93.6767401604291,1.22294037025517));
#20436=CARTESIAN_POINT('Ctrl Pts',(-201.922516654998,94.8467460489523,1.28374318133958));
#20437=CARTESIAN_POINT('Ctrl Pts',(-201.923792939525,94.9976530037673,1.29157655282255));
#20438=CARTESIAN_POINT('Ctrl Pts',(-201.929615821727,94.9968993793473,0.208423447177457));
#20439=CARTESIAN_POINT('Ctrl Pts',(-201.934957629034,95.7021699935174,0.244887843987842));
#20440=CARTESIAN_POINT('Ctrl Pts',(-202.525017792303,97.4423245699489,0.334321680399662));
#20441=CARTESIAN_POINT('Ctrl Pts',(-205.417647311761,98.6092821234889,0.476724956412918));
#20442=CARTESIAN_POINT('Ctrl Pts',(-208.260128930045,96.6049848945777,0.635633275217225));
#20443=CARTESIAN_POINT('Ctrl Pts',(-208.114979909401,93.1280855192232,0.794541594021532));
#20444=CARTESIAN_POINT('Ctrl Pts',(-205.113462578231,91.3679026833885,0.953449912825839));
#20445=CARTESIAN_POINT('Ctrl Pts',(-202.417551634193,92.7304286396575,1.09141053054448));
#20446=CARTESIAN_POINT('Ctrl Pts',(-201.933584023895,94.3813001345165,1.17640170866169));
#20447=CARTESIAN_POINT('Ctrl Pts',(-201.930545984431,95.0016532623852,1.20842344717746));
#20448=CARTESIAN_POINT('Ctrl Pts',(-206.913465996665,96.6359872033749,0.));
#20449=CARTESIAN_POINT('Ctrl Pts',(-207.457950030113,95.9991535645904,0.0529694396014356));
#20450=CARTESIAN_POINT('Ctrl Pts',(-207.850594391536,94.1490681946565,0.158908318804307));
#20451=CARTESIAN_POINT('Ctrl Pts',(-205.826561431148,92.1388044389514,0.317816637608613));
#20452=CARTESIAN_POINT('Ctrl Pts',(-203.043475148172,92.7574356177759,0.47672495641292));
#20453=CARTESIAN_POINT('Ctrl Pts',(-202.054677609388,95.4292087310772,0.635633275217227));
#20454=CARTESIAN_POINT('Ctrl Pts',(-203.765838544743,97.7088433519493,0.794541594021533));
#20455=CARTESIAN_POINT('Ctrl Pts',(-206.608600156496,97.5043849446744,0.953449912825841));
#20456=CARTESIAN_POINT('Ctrl Pts',(-207.976549680276,95.0042515457814,1.11235823163015));
#20457=CARTESIAN_POINT('Ctrl Pts',(-206.615663378372,92.5000669808854,1.27126655043445));
#20458=CARTESIAN_POINT('Ctrl Pts',(-203.773539638765,92.2878672629311,1.43017486923876));
#20459=CARTESIAN_POINT('Ctrl Pts',(-202.055828455909,94.5620846373259,1.58908318804307));
#20460=CARTESIAN_POINT('Ctrl Pts',(-203.037297256324,97.2377952804476,1.74799150684737));
#20461=CARTESIAN_POINT('Ctrl Pts',(-205.818151727977,97.8619118255793,1.90689982565168));
#20462=CARTESIAN_POINT('Ctrl Pts',(-207.848933001711,95.8622636572055,2.06580814445599));
#20463=CARTESIAN_POINT('Ctrl Pts',(-207.267844746755,93.0720998408888,2.2247164632603));
#20464=CARTESIAN_POINT('Ctrl Pts',(-204.607621579145,92.0494142928463,2.3836247820646));
#20465=CARTESIAN_POINT('Ctrl Pts',(-202.307126657076,93.7317922834607,2.54253310086891));
#20466=CARTESIAN_POINT('Ctrl Pts',(-202.47542787224,96.5768491563952,2.70144141967321));
#20467=CARTESIAN_POINT('Ctrl Pts',(-204.958228619701,97.9762682393428,2.86034973847752));
#20468=CARTESIAN_POINT('Ctrl Pts',(-207.479324891018,96.6470779176025,3.01925805728183));
#20469=CARTESIAN_POINT('Ctrl Pts',(-207.727403818342,93.8078649448984,3.17816637608613));
#20470=CARTESIAN_POINT('Ctrl Pts',(-205.475029406128,92.0615880786317,3.33707469489044));
#20471=CARTESIAN_POINT('Ctrl Pts',(-202.787153344895,93.0092144139677,3.49598301369475));
#20472=CARTESIAN_POINT('Ctrl Pts',(-202.127990363946,95.7819707268259,3.65489133249905));
#20473=CARTESIAN_POINT('Ctrl Pts',(-204.101853717757,97.8378250158782,3.81379965130336));
#20474=CARTESIAN_POINT('Ctrl Pts',(-206.899127544596,97.2919930488229,3.97270797010767));
#20475=CARTESIAN_POINT('Ctrl Pts',(-207.955302464772,94.6448874714171,4.13161628891197));
#20476=CARTESIAN_POINT('Ctrl Pts',(-206.302089116017,92.3233450913524,4.29052460771628));
#20477=CARTESIAN_POINT('Ctrl Pts',(-203.455135018895,92.4557300150421,4.44943292652059));
#20478=CARTESIAN_POINT('Ctrl Pts',(-202.024495869805,94.9206732241979,4.60834124532489));
#20479=CARTESIAN_POINT('Ctrl Pts',(-203.321765650688,97.4583423347725,4.7672495641292));
#20480=CARTESIAN_POINT('Ctrl Pts',(-206.15762192574,97.7422306692202,4.9261578829335));
#20481=CARTESIAN_POINT('Ctrl Pts',(-207.932183357775,95.5120725754678,5.08506620173781));
#20482=CARTESIAN_POINT('Ctrl Pts',(-207.018551859809,92.8124520678579,5.24397452054212));
#20483=CARTESIAN_POINT('Ctrl Pts',(-204.254334577707,92.1183510546639,5.40288283934642));
#20484=CARTESIAN_POINT('Ctrl Pts',(-202.173735020615,94.06611358696,5.56179115815073));
#20485=CARTESIAN_POINT('Ctrl Pts',(-202.684223608044,96.8700527448756,5.72069947695504));
#20486=CARTESIAN_POINT('Ctrl Pts',(-205.317790108664,97.9595484474823,5.87960779575935));
#20487=CARTESIAN_POINT('Ctrl Pts',(-207.660010189536,96.3357632116982,6.03851611456365));
#20488=CARTESIAN_POINT('Ctrl Pts',(-207.563562659025,93.4873651929785,6.19742443336796));
#20489=CARTESIAN_POINT('Ctrl Pts',(-205.11686953513,92.0257338589296,6.35633275217227));
#20490=CARTESIAN_POINT('Ctrl Pts',(-202.563031727655,93.2908764802563,6.51524107097657));
#20491=CARTESIAN_POINT('Ctrl Pts',(-202.243379194775,96.1229244419638,6.67414938978088));
#20492=CARTESIAN_POINT('Ctrl Pts',(-204.450965805945,97.9254878259732,6.83305770858519));
#20493=CARTESIAN_POINT('Ctrl Pts',(-207.161900829783,97.045996668703,6.99196602738949));
#20494=CARTESIAN_POINT('Ctrl Pts',(-207.890829335995,94.2907586332476,7.15087434619381));
#20495=CARTESIAN_POINT('Ctrl Pts',(-205.969477817168,92.1857451557867,7.3097826649981));
#20496=CARTESIAN_POINT('Ctrl Pts',(-203.159319871215,92.660809065156,7.46869098380242));
#20497=CARTESIAN_POINT('Ctrl Pts',(-202.036676894431,95.2804170789368,7.62759930260672));
#20498=CARTESIAN_POINT('Ctrl Pts',(-203.630775420383,97.6429418489121,7.78650762141103));
#20499=CARTESIAN_POINT('Ctrl Pts',(-206.480163737388,97.5824470714193,7.94541594021534));
#20500=CARTESIAN_POINT('Ctrl Pts',(-207.972554483439,95.1543936823264,8.10432425901963));
#20501=CARTESIAN_POINT('Ctrl Pts',(-206.739740502701,92.5847938909029,8.26323257782395));
#20502=CARTESIAN_POINT('Ctrl Pts',(-203.911951873806,92.2294280660402,8.42214089662825));
#20503=CARTESIAN_POINT('Ctrl Pts',(-202.081673606117,94.4140916241222,8.58104921543256));
#20504=CARTESIAN_POINT('Ctrl Pts',(-202.926884358809,97.1359094326323,8.73995753423688));
#20505=CARTESIAN_POINT('Ctrl Pts',(-205.67270436056,97.899549345923,8.89886585304117));
#20506=CARTESIAN_POINT('Ctrl Pts',(-207.801796523227,96.0049148265353,9.05777417184549));
#20507=CARTESIAN_POINT('Ctrl Pts',(-207.3622329485,93.188985625905,9.21668249064978));
#20508=CARTESIAN_POINT('Ctrl Pts',(-204.757000608778,92.033374162112,9.3755908094541));
#20509=CARTESIAN_POINT('Ctrl Pts',(-202.374547394973,93.5975321091309,9.5344991282584));
#20510=CARTESIAN_POINT('Ctrl Pts',(-202.399079785317,96.4474569434051,9.69340744706271));
#20511=CARTESIAN_POINT('Ctrl Pts',(-204.808106758534,97.9703694298923,9.85231576586701));
#20512=CARTESIAN_POINT('Ctrl Pts',(-207.393059310776,96.7700804222594,10.0112240846713));
#20513=CARTESIAN_POINT('Ctrl Pts',(-207.784081833628,93.9470014673218,10.1701324034756));
#20514=CARTESIAN_POINT('Ctrl Pts',(-205.622689248516,92.0892997979969,10.3290407222799));
#20515=CARTESIAN_POINT('Ctrl Pts',(-202.890422120034,92.9000955415738,10.4879490410842));
#20516=CARTESIAN_POINT('Ctrl Pts',(-202.092192413589,95.6360602224381,10.6468573598885));
#20517=CARTESIAN_POINT('Ctrl Pts',(-203.959808202401,97.7888920004845,10.8057656786928));
#20518=CARTESIAN_POINT('Ctrl Pts',(-206.781060205243,97.3848987633562,10.9646739974972));
#20519=CARTESIAN_POINT('Ctrl Pts',(-207.96945611846,94.7944569955031,11.1235823163015));
#20520=CARTESIAN_POINT('Ctrl Pts',(-206.43548785127,92.3924547568613,11.2824906351058));
#20521=CARTESIAN_POINT('Ctrl Pts',(-203.585480366186,92.3810208531348,11.4413989539101));
#20522=CARTESIAN_POINT('Ctrl Pts',(-202.03228867159,94.7706377594659,11.6003072727144));
#20523=CARTESIAN_POINT('Ctrl Pts',(-203.199861553383,97.3705314043844,11.7592155915187));
#20524=CARTESIAN_POINT('Ctrl Pts',(-206.017781243261,97.7971483527026,11.918123910323));
#20525=CARTESIAN_POINT('Ctrl Pts',(-207.902610464846,95.6593709544117,12.0770322291273));
#20526=CARTESIAN_POINT('Ctrl Pts',(-207.126358854139,92.9170896347696,12.2359405479316));
#20527=CARTESIAN_POINT('Ctrl Pts',(-204.400685211829,92.0843972577109,12.3948488667359));
#20528=CARTESIAN_POINT('Ctrl Pts',(-202.2244566689,93.9246968876966,12.5537571855402));
#20529=CARTESIAN_POINT('Ctrl Pts',(-202.592815230243,96.7508223925955,12.7126655043445));
#20530=CARTESIAN_POINT('Ctrl Pts',(-205.168053883906,97.9718134965553,12.8715738231488));
#20531=CARTESIAN_POINT('Ctrl Pts',(-207.589222615081,96.4682792021923,13.0304821419532));
#20532=CARTESIAN_POINT('Ctrl Pts',(-207.636620992011,93.6186429459658,13.1893904607575));
#20533=CARTESIAN_POINT('Ctrl Pts',(-205.266794712318,92.0354193976255,13.3482987795618));
#20534=CARTESIAN_POINT('Ctrl Pts',(-202.652374022519,93.1700902112655,13.5072070983661));
#20535=CARTESIAN_POINT('Ctrl Pts',(-202.190230589454,95.9824018662228,13.6661154171704));
#20536=CARTESIAN_POINT('Ctrl Pts',(-204.30405234878,97.8940584713035,13.8250237359747));
#20537=CARTESIAN_POINT('Ctrl Pts',(-207.055911134185,97.1524746141731,13.983932054779));
#20538=CARTESIAN_POINT('Ctrl Pts',(-207.922933574598,94.4375260926946,14.1428403735833));
#20539=CARTESIAN_POINT('Ctrl Pts',(-206.110243173882,92.2382473541743,14.3017486923876));
#20540=CARTESIAN_POINT('Ctrl Pts',(-203.279694258837,92.5709125915988,14.4606570111919));
#20541=CARTESIAN_POINT('Ctrl Pts',(-202.026302381485,95.1305379788577,14.6195653299962));
#20542=CARTESIAN_POINT('Ctrl Pts',(-203.499163323573,97.5704876821364,14.7784736488005));
#20543=CARTESIAN_POINT('Ctrl Pts',(-206.347974392351,97.6538428510329,14.9373819676048));
#20544=CARTESIAN_POINT('Ctrl Pts',(-207.960977942727,95.3041848805748,15.0962902864091));
#20545=CARTESIAN_POINT('Ctrl Pts',(-206.859389309675,92.6756529394601,15.2551986052134));
#20546=CARTESIAN_POINT('Ctrl Pts',(-204.053134786262,92.1780577939307,15.4141069240178));
#20547=CARTESIAN_POINT('Ctrl Pts',(-202.114952716846,94.2675848505183,15.573015242822));
#20548=CARTESIAN_POINT('Ctrl Pts',(-202.821755934838,97.0285878680713,15.7319235616264));
#20549=CARTESIAN_POINT('Ctrl Pts',(-205.525536181393,97.9297919249001,15.8908318804307));
#20550=CARTESIAN_POINT('Ctrl Pts',(-207.747537161995,96.1450208713066,16.049740199235));
#20551=CARTESIAN_POINT('Ctrl Pts',(-207.450572136011,93.3104550077017,16.2086485180393));
#20552=CARTESIAN_POINT('Ctrl Pts',(-204.907062940556,92.0249535940473,16.3675568368436));
#20553=CARTESIAN_POINT('Ctrl Pts',(-202.448523832117,93.4667171925034,16.5264651556479));
#20554=CARTESIAN_POINT('Ctrl Pts',(-202.32963244197,96.3146411010228,16.6853734744522));
#20555=CARTESIAN_POINT('Ctrl Pts',(-204.657905606643,97.9563585591527,16.8442817932565));
#20556=CARTESIAN_POINT('Ctrl Pts',(-207.301870809105,96.8897181314193,17.0031901120608));
#20557=CARTESIAN_POINT('Ctrl Pts',(-207.831183483043,94.0865595762447,17.1620984308651));
#20558=CARTESIAN_POINT('Ctrl Pts',(-206.459639356019,92.7843106836636,17.268037310068));
#20559=CARTESIAN_POINT('Ctrl Pts',(-205.650199997975,92.567913197965,17.3210067496694));
#20560=CARTESIAN_POINT('Ctrl Pts',(-207.054331550342,96.7564253212268,-0.107002249889811));
#20561=CARTESIAN_POINT('Ctrl Pts',(-207.63889941333,96.0727092589846,-0.0540328102883751));
#20562=CARTESIAN_POINT('Ctrl Pts',(-208.060449470211,94.086424290814,0.0519060689144962));
#20563=CARTESIAN_POINT('Ctrl Pts',(-205.887411236606,91.9281689233017,0.210814387718803));
#20564=CARTESIAN_POINT('Ctrl Pts',(-202.899439687382,92.5923424967542,0.369722706523109));
#20565=CARTESIAN_POINT('Ctrl Pts',(-201.837848844186,95.4608062225673,0.528631025327416));
#20566=CARTESIAN_POINT('Ctrl Pts',(-203.674982037743,97.9082630015598,0.687539344131723));
#20567=CARTESIAN_POINT('Ctrl Pts',(-206.727022094531,97.6887527737694,0.84644766293603));
#20568=CARTESIAN_POINT('Ctrl Pts',(-208.195677336315,95.0045645361097,1.00535598174034));
#20569=CARTESIAN_POINT('Ctrl Pts',(-206.734605296727,92.3160268936789,1.16426430054464));
#20570=CARTESIAN_POINT('Ctrl Pts',(-203.68325007096,92.0882054553427,1.32317261934895));
#20571=CARTESIAN_POINT('Ctrl Pts',(-201.839084413736,94.5298461809676,1.48208093815326));
#20572=CARTESIAN_POINT('Ctrl Pts',(-202.892806991447,97.4025373097,1.64098925695756));
#20573=CARTESIAN_POINT('Ctrl Pts',(-205.878382427845,98.0726000711963,1.79989757576187));
#20574=CARTESIAN_POINT('Ctrl Pts',(-208.058665772177,95.9257417894009,1.95880589456617));
#20575=CARTESIAN_POINT('Ctrl Pts',(-207.434798957837,92.9301716729358,2.11771421337049));
#20576=CARTESIAN_POINT('Ctrl Pts',(-204.578735461701,91.8321980527698,2.27662253217479));
#20577=CARTESIAN_POINT('Ctrl Pts',(-202.108882687706,93.638429358549,2.4355308509791));
#20578=CARTESIAN_POINT('Ctrl Pts',(-202.289573902954,96.6929336490738,2.5944391697834));
#20579=CARTESIAN_POINT('Ctrl Pts',(-204.955153493922,98.1953751762611,2.75334748858771));
#20580=CARTESIAN_POINT('Ctrl Pts',(-207.661847848901,96.7683325117351,2.91225580739201));
#20581=CARTESIAN_POINT('Ctrl Pts',(-207.928189852503,93.7201023377304,3.07116412619633));
#20582=CARTESIAN_POINT('Ctrl Pts',(-205.510000124407,91.8452680484058,3.23007244500063));
#20583=CARTESIAN_POINT('Ctrl Pts',(-202.624247983725,92.8626567461976,3.38898076380494));
#20584=CARTESIAN_POINT('Ctrl Pts',(-201.916558737644,95.8395378534879,3.54788908260924));
#20585=CARTESIAN_POINT('Ctrl Pts',(-204.03573397821,98.0467400385633,3.70679740141355));
#20586=CARTESIAN_POINT('Ctrl Pts',(-207.038937530004,97.4607250097823,3.86570572021785));
#20587=CARTESIAN_POINT('Ctrl Pts',(-208.172865943145,94.6187447947018,4.02461403902216));
#20588=CARTESIAN_POINT('Ctrl Pts',(-206.397946322042,92.1262950907953,4.18352235782647));
#20589=CARTESIAN_POINT('Ctrl Pts',(-203.341405137465,92.2684259287611,4.34243067663078));
#20590=CARTESIAN_POINT('Ctrl Pts',(-201.80544518508,94.9148333450394,4.50133899543508));
#20591=CARTESIAN_POINT('Ctrl Pts',(-203.198217382139,97.6393205986763,4.66024731423939));
#20592=CARTESIAN_POINT('Ctrl Pts',(-206.242843745099,97.9441082265968,4.8191556330437));
#20593=CARTESIAN_POINT('Ctrl Pts',(-208.148044853561,95.5497703380577,4.978063951848));
#20594=CARTESIAN_POINT('Ctrl Pts',(-207.167153625324,92.651409148259,5.13697227065232));
#20595=CARTESIAN_POINT('Ctrl Pts',(-204.199440175218,91.9062098016209,5.29588058945661));
#20596=CARTESIAN_POINT('Ctrl Pts',(-201.965671024781,93.9973627302039,5.45478890826093));
#20597=CARTESIAN_POINT('Ctrl Pts',(-202.513740764756,97.0077223014663,5.61369722706523));
#20598=CARTESIAN_POINT('Ctrl Pts',(-205.341185183198,98.1774245066414,5.77260554586953));
#20599=CARTESIAN_POINT('Ctrl Pts',(-207.85583483904,96.4340994375446,5.93151386467385));
#20600=CARTESIAN_POINT('Ctrl Pts',(-207.752287033526,93.3760080327397,6.09042218347815));
#20601=CARTESIAN_POINT('Ctrl Pts',(-205.125473237418,91.8067743124966,6.24933050228246));
#20602=CARTESIAN_POINT('Ctrl Pts',(-202.383626979634,93.1650542125334,6.40823882108677));
#20603=CARTESIAN_POINT('Ctrl Pts',(-202.040442264261,96.2055919017098,6.56714713989107));
#20604=CARTESIAN_POINT('Ctrl Pts',(-204.410547002649,98.1408564100502,6.72605545869538));
#20605=CARTESIAN_POINT('Ctrl Pts',(-207.321055660813,97.1966188663592,6.88496377749968));
#20606=CARTESIAN_POINT('Ctrl Pts',(-208.103646431104,94.2385456971451,7.04387209630399));
#20607=CARTESIAN_POINT('Ctrl Pts',(-206.040848842172,91.978565322171,7.2027804151083));
#20608=CARTESIAN_POINT('Ctrl Pts',(-203.02381266809,92.4886024898798,7.36168873391261));
#20609=CARTESIAN_POINT('Ctrl Pts',(-201.818522952465,95.3010608254961,7.52059705271691));
#20610=CARTESIAN_POINT('Ctrl Pts',(-203.529975835309,97.8375099611922,7.67950537152122));
#20611=CARTESIAN_POINT('Ctrl Pts',(-206.589130442186,97.7725616787294,7.83841369032553));
#20612=CARTESIAN_POINT('Ctrl Pts',(-208.191388021049,95.1657598375562,7.99732200912982));
#20613=CARTESIAN_POINT('Ctrl Pts',(-206.867816731698,92.4069912299749,8.15623032793414));
#20614=CARTESIAN_POINT('Ctrl Pts',(-203.831851938928,92.0254640812297,8.31513864673844));
#20615=CARTESIAN_POINT('Ctrl Pts',(-201.866832232399,94.3709582170401,8.47404696554276));
#20616=CARTESIAN_POINT('Ctrl Pts',(-202.774265716439,97.2931508287983,8.63295528434705));
#20617=CARTESIAN_POINT('Ctrl Pts',(-205.722227515074,98.1130083907867,8.79186360315136));
#20618=CARTESIAN_POINT('Ctrl Pts',(-208.008059200078,96.0788946535532,8.95077192195567));
#20619=CARTESIAN_POINT('Ctrl Pts',(-207.536135830906,93.0556623565245,9.10968024075997));
#20620=CARTESIAN_POINT('Ctrl Pts',(-204.739111477825,91.8149770795743,9.26858855956429));
#20621=CARTESIAN_POINT('Ctrl Pts',(-202.181266805977,93.4942852177277,9.42749687836859));
#20622=CARTESIAN_POINT('Ctrl Pts',(-202.207605222011,96.5540158392056,9.5864051971729));
#20623=CARTESIAN_POINT('Ctrl Pts',(-204.793979960486,98.1890421082134,9.7453135159772));
#20624=CARTESIAN_POINT('Ctrl Pts',(-207.569231568544,96.9003902156756,9.90422183478152));
#20625=CARTESIAN_POINT('Ctrl Pts',(-207.989040390331,93.8694818136749,10.0631301535858));
#20626=CARTESIAN_POINT('Ctrl Pts',(-205.668530390149,91.8750198493291,10.2220384723901));
#20627=CARTESIAN_POINT('Ctrl Pts',(-202.735119200304,92.7455047598612,10.3809467911944));
#20628=CARTESIAN_POINT('Ctrl Pts',(-201.878125413517,95.6828857085255,10.5398551099987));
#20629=CARTESIAN_POINT('Ctrl Pts',(-203.88323135507,97.9942046720859,10.698763428803));
#20630=CARTESIAN_POINT('Ctrl Pts',(-206.912178308403,97.5604702578846,10.8576717476073));
#20631=CARTESIAN_POINT('Ctrl Pts',(-208.188061560614,94.7793253291012,11.0165800664117));
#20632=CARTESIAN_POINT('Ctrl Pts',(-206.541165606359,92.2004924721629,11.175488385216));
#20633=CARTESIAN_POINT('Ctrl Pts',(-203.481346249483,92.1882168272285,11.3343967040203));
#20634=CARTESIAN_POINT('Ctrl Pts',(-201.813811677403,94.7537525683722,11.4933050228246));
#20635=CARTESIAN_POINT('Ctrl Pts',(-203.067338948111,97.5450452025753,11.6522133416289));
#20636=CARTESIAN_POINT('Ctrl Pts',(-206.092708270239,98.0030688405018,11.8111216604332));
#20637=CARTESIAN_POINT('Ctrl Pts',(-208.116294863185,95.7079125301353,11.9700299792375));
#20638=CARTESIAN_POINT('Ctrl Pts',(-207.282897155748,92.7637499243336,12.1289382980418));
#20639=CARTESIAN_POINT('Ctrl Pts',(-204.356564851388,91.8697563937965,12.2878466168461));
#20640=CARTESIAN_POINT('Ctrl Pts',(-202.020126699738,93.8455352153444,12.4467549356504));
#20641=CARTESIAN_POINT('Ctrl Pts',(-202.415603084333,96.8797144482438,12.6056632544547));
#20642=CARTESIAN_POINT('Ctrl Pts',(-205.180425675956,98.1905924841865,12.764571573259));
#20643=CARTESIAN_POINT('Ctrl Pts',(-207.779836024414,96.5763709911918,12.9234798920633));
#20644=CARTESIAN_POINT('Ctrl Pts',(-207.830723775401,93.5169501923025,13.0823882108676));
#20645=CARTESIAN_POINT('Ctrl Pts',(-205.286435607392,91.8171728812507,13.241296529672));
#20646=CARTESIAN_POINT('Ctrl Pts',(-202.479546476212,93.0353758991123,13.4002048484763));
#20647=CARTESIAN_POINT('Ctrl Pts',(-201.983380964526,96.0547243339646,13.5591131672806));
#20648=CARTESIAN_POINT('Ctrl Pts',(-204.252818069524,98.1071132889195,13.7180214860849));
#20649=CARTESIAN_POINT('Ctrl Pts',(-207.207263215033,97.3109355059944,13.8769298048892));
#20650=CARTESIAN_POINT('Ctrl Pts',(-208.138114119778,94.3961178844905,14.0358381236935));
#20651=CARTESIAN_POINT('Ctrl Pts',(-206.191977063942,92.0349326277818,14.1947464424978));
#20652=CARTESIAN_POINT('Ctrl Pts',(-203.153048778256,92.3920880170776,14.3536547613021));
#20653=CARTESIAN_POINT('Ctrl Pts',(-201.80738468855,95.1401479247359,14.5125630801064));
#20654=CARTESIAN_POINT('Ctrl Pts',(-203.388674718198,97.7597218630391,14.6714713989107));
#20655=CARTESIAN_POINT('Ctrl Pts',(-206.447209580983,97.8492134733665,14.830379717715));
#20656=CARTESIAN_POINT('Ctrl Pts',(-208.178959238477,95.3265783653281,14.9892880365193));
#20657=CARTESIAN_POINT('Ctrl Pts',(-206.996273845415,92.5045391406305,15.1481963553236));
#20658=CARTESIAN_POINT('Ctrl Pts',(-203.983428456062,91.970312032054,15.3071046741279));
#20659=CARTESIAN_POINT('Ctrl Pts',(-201.902561284944,94.21366590671,15.4660129929322));
#20660=CARTESIAN_POINT('Ctrl Pts',(-202.661397947386,97.1779284645159,15.6249213117365));
#20661=CARTESIAN_POINT('Ctrl Pts',(-205.564225107822,98.1454773681632,15.7838296305409));
#20662=CARTESIAN_POINT('Ctrl Pts',(-207.949805372795,96.229315026149,15.9427379493452));
#20663=CARTESIAN_POINT('Ctrl Pts',(-207.630978373366,93.1860740721548,16.1016462681495));
#20664=CARTESIAN_POINT('Ctrl Pts',(-204.900221099437,91.8059366060685,16.2605545869538));
#20665=CARTESIAN_POINT('Ctrl Pts',(-202.260689241009,93.3538399676152,16.4194629057581));
#20666=CARTESIAN_POINT('Ctrl Pts',(-202.133045303636,96.4114223591716,16.5783712245624));
#20667=CARTESIAN_POINT('Ctrl Pts',(-204.632721299102,98.1739997850896,16.7372795433667));
#20668=CARTESIAN_POINT('Ctrl Pts',(-207.471329951093,97.0288354145798,16.896187862171));
#20669=CARTESIAN_POINT('Ctrl Pts',(-208.039609569315,94.0193139124767,17.0550961809753));
#20670=CARTESIAN_POINT('Ctrl Pts',(-206.56709509676,92.6211960514381,17.1610350601782));
#20671=CARTESIAN_POINT('Ctrl Pts',(-205.698066426161,92.3888678140614,17.2140044997796));
#20672=CARTESIAN_POINT('Ctrl Pts',(-207.195197104019,96.8768634390787,-0.214004499779621));
#20673=CARTESIAN_POINT('Ctrl Pts',(-207.819848796546,96.1462649533789,-0.161035060178185));
#20674=CARTESIAN_POINT('Ctrl Pts',(-208.270304548887,94.0237803869714,-0.0550961809753146));
#20675=CARTESIAN_POINT('Ctrl Pts',(-205.948261042063,91.7175334076522,0.103812137828992));
#20676=CARTESIAN_POINT('Ctrl Pts',(-202.755404226592,92.4272493757325,0.262720456633299));
#20677=CARTESIAN_POINT('Ctrl Pts',(-201.621020078985,95.4924037140574,0.421628775437605));
#20678=CARTESIAN_POINT('Ctrl Pts',(-203.584125530742,98.1076826511703,0.580537094241912));
#20679=CARTESIAN_POINT('Ctrl Pts',(-206.845444032567,97.8731206028643,0.739445413046219));
#20680=CARTESIAN_POINT('Ctrl Pts',(-208.414804992354,95.004877526438,0.898353731850526));
#20681=CARTESIAN_POINT('Ctrl Pts',(-206.853547215082,92.1319868064724,1.05726205065483));
#20682=CARTESIAN_POINT('Ctrl Pts',(-203.592960503155,91.8885436477545,1.21617036945914));
#20683=CARTESIAN_POINT('Ctrl Pts',(-201.622340371563,94.4976077246091,1.37507868826345));
#20684=CARTESIAN_POINT('Ctrl Pts',(-202.74831672657,97.5672793389525,1.53398700706775));
#20685=CARTESIAN_POINT('Ctrl Pts',(-205.938613127714,98.2832883168132,1.69289532587206));
#20686=CARTESIAN_POINT('Ctrl Pts',(-208.268398542644,95.9892199215965,1.85180364467636));
#20687=CARTESIAN_POINT('Ctrl Pts',(-207.601753168919,92.7882435049825,2.01071196348067));
#20688=CARTESIAN_POINT('Ctrl Pts',(-204.549849344257,91.6149818126935,2.16962028228498));
#20689=CARTESIAN_POINT('Ctrl Pts',(-201.910638718336,93.5450664336372,2.32852860108929));
#20690=CARTESIAN_POINT('Ctrl Pts',(-202.103719933668,96.8090181417526,2.48743691989359));
#20691=CARTESIAN_POINT('Ctrl Pts',(-204.952078368144,98.4144821131792,2.6463452386979));
#20692=CARTESIAN_POINT('Ctrl Pts',(-207.844370806783,96.8895871058678,2.8052535575022));
#20693=CARTESIAN_POINT('Ctrl Pts',(-208.128975886664,93.6323397305624,2.96416187630651));
#20694=CARTESIAN_POINT('Ctrl Pts',(-205.544970842687,91.6289480181799,3.12307019511082));
#20695=CARTESIAN_POINT('Ctrl Pts',(-202.461342622555,92.7160990784275,3.28197851391512));
#20696=CARTESIAN_POINT('Ctrl Pts',(-201.705127111342,95.89710498015,3.44088683271943));
#20697=CARTESIAN_POINT('Ctrl Pts',(-203.969614238663,98.2556550612482,3.59979515152374));
#20698=CARTESIAN_POINT('Ctrl Pts',(-207.178747515412,97.6294569707416,3.75870347032805));
#20699=CARTESIAN_POINT('Ctrl Pts',(-208.390429421518,94.5926021179864,3.91761178913235));
#20700=CARTESIAN_POINT('Ctrl Pts',(-206.493803528068,91.9292450902381,4.07652010793666));
#20701=CARTESIAN_POINT('Ctrl Pts',(-203.227675256036,92.0811218424802,4.23542842674097));
#20702=CARTESIAN_POINT('Ctrl Pts',(-201.586394500355,94.9089934658807,4.39433674554527));
#20703=CARTESIAN_POINT('Ctrl Pts',(-203.074669113589,97.8202988625801,4.55324506434958));
#20704=CARTESIAN_POINT('Ctrl Pts',(-206.328065564458,98.1459857839733,4.71215338315389));
#20705=CARTESIAN_POINT('Ctrl Pts',(-208.363906349347,95.5874681006477,4.8710617019582));
#20706=CARTESIAN_POINT('Ctrl Pts',(-207.31575539084,92.49036622866,5.0299700207625));
#20707=CARTESIAN_POINT('Ctrl Pts',(-204.14454577273,91.6940685485779,5.18887833956681));
#20708=CARTESIAN_POINT('Ctrl Pts',(-201.757607028947,93.9286118734479,5.34778665837111));
#20709=CARTESIAN_POINT('Ctrl Pts',(-202.343257921469,97.1453918580569,5.50669497717542));
#20710=CARTESIAN_POINT('Ctrl Pts',(-205.364580257732,98.3953005658008,5.66560329597973));
#20711=CARTESIAN_POINT('Ctrl Pts',(-208.051659488544,96.5324356633908,5.82451161478403));
#20712=CARTESIAN_POINT('Ctrl Pts',(-207.941011408027,93.2646508725009,5.98341993358834));
#20713=CARTESIAN_POINT('Ctrl Pts',(-205.134076939706,91.5878147660635,6.14232825239264));
#20714=CARTESIAN_POINT('Ctrl Pts',(-202.204222231614,93.0392319448105,6.30123657119695));
#20715=CARTESIAN_POINT('Ctrl Pts',(-201.837505333748,96.2882593614559,6.46014489000126));
#20716=CARTESIAN_POINT('Ctrl Pts',(-204.370128199352,98.3562249941271,6.61905320880556));
#20717=CARTESIAN_POINT('Ctrl Pts',(-207.480210491844,97.3472410640154,6.77796152760988));
#20718=CARTESIAN_POINT('Ctrl Pts',(-208.316463526213,94.1863327610426,6.93686984641418));
#20719=CARTESIAN_POINT('Ctrl Pts',(-206.112219867177,91.7713854885552,7.09577816521849));
#20720=CARTESIAN_POINT('Ctrl Pts',(-202.888305464964,92.3163959146037,7.25468648402279));
#20721=CARTESIAN_POINT('Ctrl Pts',(-201.600369010499,95.3217045720554,7.4135948028271));
#20722=CARTESIAN_POINT('Ctrl Pts',(-203.429176250236,98.0320780734722,7.5725031216314));
#20723=CARTESIAN_POINT('Ctrl Pts',(-206.698097146984,97.9626762860395,7.73141144043571));
#20724=CARTESIAN_POINT('Ctrl Pts',(-208.410221558658,95.177125992786,7.89031975924002));
#20725=CARTESIAN_POINT('Ctrl Pts',(-206.995892960696,92.229188569047,8.04922807804433));
#20726=CARTESIAN_POINT('Ctrl Pts',(-203.751752004051,91.8215000964192,8.20813639684864));
#20727=CARTESIAN_POINT('Ctrl Pts',(-201.651990858682,94.3278248099579,8.36704471565293));
#20728=CARTESIAN_POINT('Ctrl Pts',(-202.621647074068,97.4503922249643,8.52595303445725));
#20729=CARTESIAN_POINT('Ctrl Pts',(-205.771750669589,98.3264674356504,8.68486135326155));
#20730=CARTESIAN_POINT('Ctrl Pts',(-208.214321876929,96.1528744805713,8.84376967206586));
#20731=CARTESIAN_POINT('Ctrl Pts',(-207.710038713311,92.9223390871439,9.00267799087017));
#20732=CARTESIAN_POINT('Ctrl Pts',(-204.721222346873,91.5965799970367,9.16158630967447));
#20733=CARTESIAN_POINT('Ctrl Pts',(-201.987986216981,93.3910383263244,9.32049462847878));
#20734=CARTESIAN_POINT('Ctrl Pts',(-202.016130658706,96.660574735006,9.47940294728309));
#20735=CARTESIAN_POINT('Ctrl Pts',(-204.779853162439,98.4077147865346,9.63831126608739));
#20736=CARTESIAN_POINT('Ctrl Pts',(-207.745403826312,97.0307000090919,9.7972195848917));
#20737=CARTESIAN_POINT('Ctrl Pts',(-208.193998947033,93.7919621600278,9.956127903696));
#20738=CARTESIAN_POINT('Ctrl Pts',(-205.71437153178,91.6607399006612,10.1150362225003));
#20739=CARTESIAN_POINT('Ctrl Pts',(-202.579816280574,92.5909139781486,10.2739445413046));
#20740=CARTESIAN_POINT('Ctrl Pts',(-201.664058413444,95.7297111946129,10.4328528601089));
#20741=CARTESIAN_POINT('Ctrl Pts',(-203.80665450774,98.1995173436874,10.5917611789132));
#20742=CARTESIAN_POINT('Ctrl Pts',(-207.043296411563,97.736041752413,10.7506694977175));
#20743=CARTESIAN_POINT('Ctrl Pts',(-208.406667002767,94.7641936626994,10.9095778165219));
#20744=CARTESIAN_POINT('Ctrl Pts',(-206.646843361447,92.0085301874643,11.0684861353262));
#20745=CARTESIAN_POINT('Ctrl Pts',(-203.37721213278,91.9954128013223,11.2273944541305));
#20746=CARTESIAN_POINT('Ctrl Pts',(-201.595334683216,94.7368673772781,11.3863027729348));
#20747=CARTESIAN_POINT('Ctrl Pts',(-202.934816342839,97.7195590007664,11.5452110917391));
#20748=CARTESIAN_POINT('Ctrl Pts',(-206.167635297217,98.2089893283008,11.7041194105434));
#20749=CARTESIAN_POINT('Ctrl Pts',(-208.329979261524,95.7564541058591,11.8630277293477));
#20750=CARTESIAN_POINT('Ctrl Pts',(-207.439435457357,92.6104102138975,12.021936048152));
#20751=CARTESIAN_POINT('Ctrl Pts',(-204.312444490949,91.6551155298822,12.1808443669563));
#20752=CARTESIAN_POINT('Ctrl Pts',(-201.815796730576,93.7663735429921,12.3397526857606));
#20753=CARTESIAN_POINT('Ctrl Pts',(-202.238390938423,97.0086065038919,12.4986610045649));
#20754=CARTESIAN_POINT('Ctrl Pts',(-205.192797468005,98.4093714718177,12.6575693233692));
#20755=CARTESIAN_POINT('Ctrl Pts',(-207.970449433746,96.6844627801914,12.8164776421735));
#20756=CARTESIAN_POINT('Ctrl Pts',(-208.024826558792,93.4152574386389,12.9753859609778));
#20757=CARTESIAN_POINT('Ctrl Pts',(-205.306076502467,91.5989263648761,13.1342942797821));
#20758=CARTESIAN_POINT('Ctrl Pts',(-202.306718929906,92.9006615869591,13.2932025985864));
#20759=CARTESIAN_POINT('Ctrl Pts',(-201.776531339599,96.1270468017065,13.4521109173908));
#20760=CARTESIAN_POINT('Ctrl Pts',(-204.201583790268,98.3201681065354,13.6110192361951));
#20761=CARTESIAN_POINT('Ctrl Pts',(-207.358615295882,97.4693963978157,13.7699275549994));
#20762=CARTESIAN_POINT('Ctrl Pts',(-208.353294664959,94.3547096762863,13.9288358738037));
#20763=CARTESIAN_POINT('Ctrl Pts',(-206.273710954002,91.8316179013893,14.087744192608));
#20764=CARTESIAN_POINT('Ctrl Pts',(-203.026403297675,92.2132634425565,14.2466525114123));
#20765=CARTESIAN_POINT('Ctrl Pts',(-201.588466995615,95.149757870614,14.4055608302166));
#20766=CARTESIAN_POINT('Ctrl Pts',(-203.278186112823,97.9489560439418,14.5644691490209));
#20767=CARTESIAN_POINT('Ctrl Pts',(-206.546444769616,98.0445840957001,14.7233774678252));
#20768=CARTESIAN_POINT('Ctrl Pts',(-208.396940534228,95.3489718500814,14.8822857866295));
#20769=CARTESIAN_POINT('Ctrl Pts',(-207.133158381155,92.333425341801,15.0411941054338));
#20770=CARTESIAN_POINT('Ctrl Pts',(-203.913722125861,91.7625662701771,15.2001024242381));
#20771=CARTESIAN_POINT('Ctrl Pts',(-201.690169853043,94.1597469629018,15.3590107430424));
#20772=CARTESIAN_POINT('Ctrl Pts',(-202.501039959935,97.3272690609605,15.5179190618467));
#20773=CARTESIAN_POINT('Ctrl Pts',(-205.602914034251,98.3611628114263,15.676827380651));
#20774=CARTESIAN_POINT('Ctrl Pts',(-208.152073583596,96.3136091809913,15.8357356994554));
#20775=CARTESIAN_POINT('Ctrl Pts',(-207.81138461072,93.0616931366079,15.9946440182597));
#20776=CARTESIAN_POINT('Ctrl Pts',(-204.893379258318,91.5869196180898,16.153552337064));
#20777=CARTESIAN_POINT('Ctrl Pts',(-202.072854649901,93.240962742727,16.3124606558683));
#20778=CARTESIAN_POINT('Ctrl Pts',(-201.936458165303,96.5082036173204,16.4713689746726));
#20779=CARTESIAN_POINT('Ctrl Pts',(-204.607536991561,98.3916410110266,16.6302772934769));
#20780=CARTESIAN_POINT('Ctrl Pts',(-207.640789093081,97.1679526977402,16.7891856122812));
#20781=CARTESIAN_POINT('Ctrl Pts',(-208.248035655587,93.9520682487087,16.9480939310855));
#20782=CARTESIAN_POINT('Ctrl Pts',(-206.674550837501,92.4580814192126,17.0540328102884));
#20783=CARTESIAN_POINT('Ctrl Pts',(-205.745932854347,92.2098224301579,17.1070022498898));
#20784=CARTESIAN_POINT('Ctrl Pts',(-207.336062657696,96.9973015569306,-0.321006749669432));
#20785=CARTESIAN_POINT('Ctrl Pts',(-208.000798179763,96.2198206477731,-0.268037310067996));
#20786=CARTESIAN_POINT('Ctrl Pts',(-208.480159627562,93.9611364831289,-0.162098430865125));
#20787=CARTESIAN_POINT('Ctrl Pts',(-206.009110847521,91.5068978920026,-0.00319011206081825));
#20788=CARTESIAN_POINT('Ctrl Pts',(-202.611368765802,92.2621562547108,0.155718206743488));
#20789=CARTESIAN_POINT('Ctrl Pts',(-201.404191313785,95.5240012055474,0.314626525547795));
#20790=CARTESIAN_POINT('Ctrl Pts',(-203.493269023741,98.307102300781,0.473534844352101));
#20791=CARTESIAN_POINT('Ctrl Pts',(-206.963865970602,98.0574884319591,0.632443163156409));
#20792=CARTESIAN_POINT('Ctrl Pts',(-208.633932648393,95.0051905167663,0.791351481960714));
#20793=CARTESIAN_POINT('Ctrl Pts',(-206.972489133437,91.9479467192658,0.950259800765022));
#20794=CARTESIAN_POINT('Ctrl Pts',(-203.50267093535,91.6888818401662,1.10916811956933));
#20795=CARTESIAN_POINT('Ctrl Pts',(-201.405596329389,94.4653692682509,1.26807643837364));
#20796=CARTESIAN_POINT('Ctrl Pts',(-202.603826461693,97.7320213682048,1.42698475717794));
#20797=CARTESIAN_POINT('Ctrl Pts',(-205.998843827582,98.4939765624303,1.58589307598225));
#20798=CARTESIAN_POINT('Ctrl Pts',(-208.478131313111,96.0526980537919,1.74480139478655));
#20799=CARTESIAN_POINT('Ctrl Pts',(-207.768707380001,92.6463153370295,1.90370971359086));
#20800=CARTESIAN_POINT('Ctrl Pts',(-204.520963226813,91.3977655726169,2.06261803239517));
#20801=CARTESIAN_POINT('Ctrl Pts',(-201.712394748966,93.4517035087255,2.22152635119947));
#20802=CARTESIAN_POINT('Ctrl Pts',(-201.917865964382,96.9251026344312,2.38043467000378));
#20803=CARTESIAN_POINT('Ctrl Pts',(-204.949003242364,98.6335890500974,2.53934298880809));
#20804=CARTESIAN_POINT('Ctrl Pts',(-208.026893764665,97.0108417000006,2.69825130761239));
#20805=CARTESIAN_POINT('Ctrl Pts',(-208.329761920824,93.5445771233942,2.8571596264167));
#20806=CARTESIAN_POINT('Ctrl Pts',(-205.579941560967,91.4126279879542,3.01606794522101));
#20807=CARTESIAN_POINT('Ctrl Pts',(-202.298437261384,92.5695414106573,3.17497626402532));
#20808=CARTESIAN_POINT('Ctrl Pts',(-201.49369548504,95.9546721068121,3.33388458282962));
#20809=CARTESIAN_POINT('Ctrl Pts',(-203.903494499117,98.4645700839332,3.49279290163393));
#20810=CARTESIAN_POINT('Ctrl Pts',(-207.318557500821,97.7981889317011,3.65170122043824));
#20811=CARTESIAN_POINT('Ctrl Pts',(-208.607992899891,94.5664594412711,3.81060953924254));
#20812=CARTESIAN_POINT('Ctrl Pts',(-206.589660734093,91.732195089681,3.96951785804685));
#20813=CARTESIAN_POINT('Ctrl Pts',(-203.113945374607,91.8938177561992,4.12842617685116));
#20814=CARTESIAN_POINT('Ctrl Pts',(-201.367343815629,94.903153586722,4.28733449565546));
#20815=CARTESIAN_POINT('Ctrl Pts',(-202.95112084504,98.0012771264839,4.44624281445977));
#20816=CARTESIAN_POINT('Ctrl Pts',(-206.413287383817,98.3478633413499,4.60515113326407));
#20817=CARTESIAN_POINT('Ctrl Pts',(-208.579767845133,95.6251658632375,4.76405945206838));
#20818=CARTESIAN_POINT('Ctrl Pts',(-207.464357156355,92.3293233090611,4.92296777087269));
#20819=CARTESIAN_POINT('Ctrl Pts',(-204.089651370241,91.481927295535,5.081876089677));
#20820=CARTESIAN_POINT('Ctrl Pts',(-201.549543033112,93.8598610166918,5.2407844084813));
#20821=CARTESIAN_POINT('Ctrl Pts',(-202.172775078182,97.2830614146476,5.3996927272856));
#20822=CARTESIAN_POINT('Ctrl Pts',(-205.387975332266,98.61317662496,5.55860104608992));
#20823=CARTESIAN_POINT('Ctrl Pts',(-208.247484138049,96.6307718892372,5.71750936489422));
#20824=CARTESIAN_POINT('Ctrl Pts',(-208.129735782527,93.1532937122619,5.87641768369853));
#20825=CARTESIAN_POINT('Ctrl Pts',(-205.142680641995,91.3688552196306,6.03532600250283));
#20826=CARTESIAN_POINT('Ctrl Pts',(-202.024817483593,92.9134096770875,6.19423432130715));
#20827=CARTESIAN_POINT('Ctrl Pts',(-201.634568403234,96.3709268212019,6.35314264011144));
#20828=CARTESIAN_POINT('Ctrl Pts',(-204.329709396056,98.5715935782041,6.51205095891576));
#20829=CARTESIAN_POINT('Ctrl Pts',(-207.639365322875,97.4978632616717,6.67095927772006));
#20830=CARTESIAN_POINT('Ctrl Pts',(-208.529280621322,94.13411982494,6.82986759652437));
#20831=CARTESIAN_POINT('Ctrl Pts',(-206.183590892181,91.5642056549396,6.98877591532867));
#20832=CARTESIAN_POINT('Ctrl Pts',(-202.752798261839,92.1441893393276,7.14768423413298));
#20833=CARTESIAN_POINT('Ctrl Pts',(-201.382215068533,95.3423483186146,7.30659255293729));
#20834=CARTESIAN_POINT('Ctrl Pts',(-203.328376665162,98.2266461857523,7.46550087174159));
#20835=CARTESIAN_POINT('Ctrl Pts',(-206.807063851782,98.1527908933495,7.6244091905459));
#20836=CARTESIAN_POINT('Ctrl Pts',(-208.629055096267,95.1884921480159,7.78331750935021));
#20837=CARTESIAN_POINT('Ctrl Pts',(-207.123969189693,92.0513859081191,7.94222582815452));
#20838=CARTESIAN_POINT('Ctrl Pts',(-203.671652069173,91.6175361116086,8.10113414695882));
#20839=CARTESIAN_POINT('Ctrl Pts',(-201.437149484965,94.2846914028758,8.26004246576313));
#20840=CARTESIAN_POINT('Ctrl Pts',(-202.469028431698,97.6076336211302,8.41895078456744));
#20841=CARTESIAN_POINT('Ctrl Pts',(-205.821273824104,98.5399264805142,8.57785910337175));
#20842=CARTESIAN_POINT('Ctrl Pts',(-208.420584553779,96.2268543075893,8.73676742217604));
#20843=CARTESIAN_POINT('Ctrl Pts',(-207.883941595716,92.7890158177634,8.89567574098036));
#20844=CARTESIAN_POINT('Ctrl Pts',(-204.70333321592,91.3781829144989,9.05458405978466));
#20845=CARTESIAN_POINT('Ctrl Pts',(-201.794705627984,93.2877914349212,9.21349237858898));
#20846=CARTESIAN_POINT('Ctrl Pts',(-201.824656095401,96.7671336308065,9.37240069739327));
#20847=CARTESIAN_POINT('Ctrl Pts',(-204.765726364391,98.6263874648557,9.53130901619759));
#20848=CARTESIAN_POINT('Ctrl Pts',(-207.92157608408,97.1610098025081,9.69021733500189));
#20849=CARTESIAN_POINT('Ctrl Pts',(-208.398957503736,93.7144425063808,9.84912565380619));
#20850=CARTESIAN_POINT('Ctrl Pts',(-205.760212673412,91.4464599519933,10.0080339726105));
#20851=CARTESIAN_POINT('Ctrl Pts',(-202.424513360844,92.4363231964359,10.1669422914148));
#20852=CARTESIAN_POINT('Ctrl Pts',(-201.449991413372,95.7765366807004,10.3258506102191));
#20853=CARTESIAN_POINT('Ctrl Pts',(-203.730077660409,98.4048300152887,10.4847589290234));
#20854=CARTESIAN_POINT('Ctrl Pts',(-207.174414514723,97.9116132469416,10.6436672478277));
#20855=CARTESIAN_POINT('Ctrl Pts',(-208.625272444921,94.7490619962975,10.802575566632));
#20856=CARTESIAN_POINT('Ctrl Pts',(-206.752521116536,91.8165679027658,10.9614838854363));
#20857=CARTESIAN_POINT('Ctrl Pts',(-203.273078016077,91.802608775416,11.1203922042406));
#20858=CARTESIAN_POINT('Ctrl Pts',(-201.376857689029,94.7199821861842,11.279300523045));
#20859=CARTESIAN_POINT('Ctrl Pts',(-202.802293737567,97.8940727989574,11.4382088418493));
#20860=CARTESIAN_POINT('Ctrl Pts',(-206.242562324195,98.4149098161,11.5971171606536));
#20861=CARTESIAN_POINT('Ctrl Pts',(-208.543663659863,95.8049956815827,11.7560254794579));
#20862=CARTESIAN_POINT('Ctrl Pts',(-207.595973758966,92.4570705034615,11.9149337982622));
#20863=CARTESIAN_POINT('Ctrl Pts',(-204.268324130509,91.4404746659679,12.0738421170665));
#20864=CARTESIAN_POINT('Ctrl Pts',(-201.611466761415,93.6872118706398,12.2327504358708));
#20865=CARTESIAN_POINT('Ctrl Pts',(-202.061178792513,97.1374985595401,12.3916587546751));
#20866=CARTESIAN_POINT('Ctrl Pts',(-205.205169260054,98.628150459449,12.5505670734794));
#20867=CARTESIAN_POINT('Ctrl Pts',(-208.161062843079,96.7925545691908,12.7094753922837));
#20868=CARTESIAN_POINT('Ctrl Pts',(-208.218929342183,93.3135646849756,12.868383711088));
#20869=CARTESIAN_POINT('Ctrl Pts',(-205.325717397541,91.3806798485012,13.0272920298923));
#20870=CARTESIAN_POINT('Ctrl Pts',(-202.133891383599,92.765947274806,13.1862003486966));
#20871=CARTESIAN_POINT('Ctrl Pts',(-201.569681714672,96.1993692694483,13.3451086675009));
#20872=CARTESIAN_POINT('Ctrl Pts',(-204.150349511013,98.5332229241514,13.5040169863052));
#20873=CARTESIAN_POINT('Ctrl Pts',(-207.50996737673,97.6278572896369,13.6629253051096));
#20874=CARTESIAN_POINT('Ctrl Pts',(-208.568475210139,94.3133014680822,13.8218336239139));
#20875=CARTESIAN_POINT('Ctrl Pts',(-206.355444844063,91.6283031749969,13.9807419427182));
#20876=CARTESIAN_POINT('Ctrl Pts',(-202.899757817094,92.0344388680353,14.1396502615225));
#20877=CARTESIAN_POINT('Ctrl Pts',(-201.369549302679,95.1593678164922,14.2985585803268));
#20878=CARTESIAN_POINT('Ctrl Pts',(-203.167697507449,98.1381902248446,14.4574668991311));
#20879=CARTESIAN_POINT('Ctrl Pts',(-206.645679958249,98.2399547180336,14.6163752179354));
#20880=CARTESIAN_POINT('Ctrl Pts',(-208.614921829979,95.3713653348348,14.7752835367397));
#20881=CARTESIAN_POINT('Ctrl Pts',(-207.270042916896,92.1623115429714,14.934191855544));
#20882=CARTESIAN_POINT('Ctrl Pts',(-203.844015795661,91.5548205083004,15.0931001743483));
#20883=CARTESIAN_POINT('Ctrl Pts',(-201.477778421142,94.1058280190935,15.2520084931526));
#20884=CARTESIAN_POINT('Ctrl Pts',(-202.340681972483,97.4766096574051,15.4109168119569));
#20885=CARTESIAN_POINT('Ctrl Pts',(-205.64160296068,98.5768482546894,15.5698251307612));
#20886=CARTESIAN_POINT('Ctrl Pts',(-208.354341794396,96.3979033358336,15.7287334495655));
#20887=CARTESIAN_POINT('Ctrl Pts',(-207.991790848075,92.937312201061,15.8876417683699));
#20888=CARTESIAN_POINT('Ctrl Pts',(-204.886537417199,91.367902630111,16.0465500871741));
#20889=CARTESIAN_POINT('Ctrl Pts',(-201.885020058793,93.1280855178388,16.2054584059785));
#20890=CARTESIAN_POINT('Ctrl Pts',(-201.739871026969,96.6049848754692,16.3643667247828));
#20891=CARTESIAN_POINT('Ctrl Pts',(-204.582352684019,98.6092822369636,16.5232750435871));
#20892=CARTESIAN_POINT('Ctrl Pts',(-207.810248235069,97.3070699809007,16.6821833623914));
#20893=CARTESIAN_POINT('Ctrl Pts',(-208.45646174186,93.8848225849406,16.8410916811957));
#20894=CARTESIAN_POINT('Ctrl Pts',(-206.782006578242,92.2949667869871,16.9470305603986));
#20895=CARTESIAN_POINT('Ctrl Pts',(-205.793799282533,92.0307770462543,17.));
#20896=CARTESIAN_POINT('Ctrl Pts',(-206.913465996665,96.6359872033749,0.));
#20897=CARTESIAN_POINT('Ctrl Pts',(-206.975062233787,96.5781018655823,3.0968450357692E-17));
#20898=CARTESIAN_POINT('Ctrl Pts',(-207.033286127394,96.517064861521,4.93396470770506E-17));
#20899=CARTESIAN_POINT('Ctrl Pts',(-207.088141455004,96.4532612528611,2.77555756156289E-17));
#20900=CARTESIAN_POINT('Ctrl Pts',(-207.144450798064,96.3877664423286,5.59938883280038E-18));
#20901=CARTESIAN_POINT('Ctrl Pts',(-207.197211066199,96.3193559864889,1.56478474477103E-16));
#20902=CARTESIAN_POINT('Ctrl Pts',(-207.246400774978,96.2483978328537,8.32667268468867E-17));
#20903=CARTESIAN_POINT('Ctrl Pts',(-207.297350807049,96.1749003413407,7.43499329068896E-18));
#20904=CARTESIAN_POINT('Ctrl Pts',(-207.344470743098,96.0986690282088,2.71682604868357E-17));
#20905=CARTESIAN_POINT('Ctrl Pts',(-207.387701617095,96.0200685851594,-3.46944695195361E-17));
#20906=CARTESIAN_POINT('Ctrl Pts',(-207.406615124468,95.9856808913252,-6.17594138973238E-17));
#20907=CARTESIAN_POINT('Ctrl Pts',(-207.424783744567,95.9508392224169,2.01136707471298E-16));
#20908=CARTESIAN_POINT('Ctrl Pts',(-207.442200082494,95.9155720190512,2.15105711021124E-16));
#20909=CARTESIAN_POINT('Ctrl Pts',(-207.451657198057,95.8964218383858,2.22690915294919E-16));
#20910=CARTESIAN_POINT('Ctrl Pts',(-207.460892474714,95.8771461685267,3.72933574804102E-16));
#20911=CARTESIAN_POINT('Ctrl Pts',(-207.469904527905,95.8577494362717,3.88578058618805E-16));
#20912=CARTESIAN_POINT('Ctrl Pts',(-207.478555310542,95.8391302702473,4.03595394409402E-16));
#20913=CARTESIAN_POINT('Ctrl Pts',(-207.487002900789,95.8203935450865,3.88581800676704E-16));
#20914=CARTESIAN_POINT('Ctrl Pts',(-207.495231967652,95.8015759912223,3.60822483003176E-16));
#20915=CARTESIAN_POINT('Ctrl Pts',(-207.531772133063,95.7180189437175,2.37560626425314E-16));
#20916=CARTESIAN_POINT('Ctrl Pts',(-207.564052932394,95.6327781953704,1.86682596890399E-16));
#20917=CARTESIAN_POINT('Ctrl Pts',(-207.592050831023,95.5462530210923,2.22044604925031E-16));
#20918=CARTESIAN_POINT('Ctrl Pts',(-207.620513276378,95.458292203845,2.57993346458143E-16));
#20919=CARTESIAN_POINT('Ctrl Pts',(-207.644550007454,95.3690032283074,-2.49369539605486E-16));
#20920=CARTESIAN_POINT('Ctrl Pts',(-207.664097180383,95.278768433218,-3.46944695195361E-16));
#20921=CARTESIAN_POINT('Ctrl Pts',(-207.683347083547,95.1899059120856,-4.43035945993059E-16));
#20922=CARTESIAN_POINT('Ctrl Pts',(-207.698243217594,95.1001252116962,-1.09324133867228E-16));
#20923=CARTESIAN_POINT('Ctrl Pts',(-207.708681596094,95.0097684816411,-1.94289029309402E-16));
#20924=CARTESIAN_POINT('Ctrl Pts',(-207.712775443857,94.9743313017009,-2.27611575250926E-16));
#20925=CARTESIAN_POINT('Ctrl Pts',(-207.716183130269,94.9388053405125,4.4208590596913E-16));
#20926=CARTESIAN_POINT('Ctrl Pts',(-207.71889639163,94.903210714114,4.85722573273506E-16));
#20927=CARTESIAN_POINT('Ctrl Pts',(-207.720491854529,94.8822802182006,5.1138198254676E-16));
#20928=CARTESIAN_POINT('Ctrl Pts',(-207.721847182612,94.8613259758214,7.42875535366934E-17));
#20929=CARTESIAN_POINT('Ctrl Pts',(-207.722960502641,94.8403520552435,6.93889390390723E-17));
#20930=CARTESIAN_POINT('Ctrl Pts',(-207.723721970302,94.8260067081621,6.60384769771266E-17));
#20931=CARTESIAN_POINT('Ctrl Pts',(-207.724370161868,94.8116517728123,2.77396210343816E-16));
#20932=CARTESIAN_POINT('Ctrl Pts',(-207.724904092468,94.7973039113478,2.77555756156289E-16));
#20933=CARTESIAN_POINT('Ctrl Pts',(-207.728446434094,94.7021135872458,2.78614256591085E-16));
#20934=CARTESIAN_POINT('Ctrl Pts',(-207.726972757336,94.6070734840445,4.25745817027648E-17));
#20935=CARTESIAN_POINT('Ctrl Pts',(-207.720425227949,94.5125829664624,2.77555756156289E-17));
#20936=CARTESIAN_POINT('Ctrl Pts',(-207.713899630728,94.41840896242,1.29862085419292E-17));
#20937=CARTESIAN_POINT('Ctrl Pts',(-207.702334474037,94.3247799136568,-6.21676310273157E-17));
#20938=CARTESIAN_POINT('Ctrl Pts',(-207.685624510351,94.2320732634053,-8.32667268468867E-17));
#20939=CARTESIAN_POINT('Ctrl Pts',(-207.683541691529,94.2205178130349,-8.58966304615819E-17));
#20940=CARTESIAN_POINT('Ctrl Pts',(-207.681378875184,94.2089766813724,8.3661212389091E-17));
#20941=CARTESIAN_POINT('Ctrl Pts',(-207.679135800651,94.197450591266,8.32667268468867E-17));
#20942=CARTESIAN_POINT('Ctrl Pts',(-207.661515002607,94.1069057150043,8.1200767834121E-17));
#20943=CARTESIAN_POINT('Ctrl Pts',(-207.638945751039,94.017288753037,1.06755513380276E-16));
#20944=CARTESIAN_POINT('Ctrl Pts',(-207.611703055832,93.9288370382536,1.38777878078145E-16));
#20945=CARTESIAN_POINT('Ctrl Pts',(-207.600776295581,93.8933599801309,1.51621713795702E-16));
#20946=CARTESIAN_POINT('Ctrl Pts',(-207.589097112068,93.8580704314563,2.10854356106776E-16));
#20947=CARTESIAN_POINT('Ctrl Pts',(-207.576680955897,93.8229840703899,2.4980018054066E-16));
#20948=CARTESIAN_POINT('Ctrl Pts',(-207.570899597757,93.8066467421239,2.67934597990291E-16));
#20949=CARTESIAN_POINT('Ctrl Pts',(-207.564958436528,93.7903534718742,8.50030008580217E-17));
#20950=CARTESIAN_POINT('Ctrl Pts',(-207.55885894084,93.7741058681104,8.32667268468867E-17));
#20951=CARTESIAN_POINT('Ctrl Pts',(-207.553795395264,93.7606177887079,8.18253449626879E-17));
#20952=CARTESIAN_POINT('Ctrl Pts',(-207.54862605565,93.7471700690316,4.26988678161571E-17));
#20953=CARTESIAN_POINT('Ctrl Pts',(-207.543352966221,93.7337654693977,5.55111512312578E-17));
#20954=CARTESIAN_POINT('Ctrl Pts',(-207.509119317179,93.646740895753,1.38690323460505E-16));
#20955=CARTESIAN_POINT('Ctrl Pts',(-207.470507251376,93.5615075862816,3.77458317449025E-16));
#20956=CARTESIAN_POINT('Ctrl Pts',(-207.427849249462,93.4782966850494,3.60822483003176E-16));
#20957=CARTESIAN_POINT('Ctrl Pts',(-207.383612733185,93.3920066521892,3.43571057051397E-16));
#20958=CARTESIAN_POINT('Ctrl Pts',(-207.335025179508,93.3078907458115,-1.10988550360456E-16));
#20959=CARTESIAN_POINT('Ctrl Pts',(-207.282401401832,93.2262103191478,-2.22044604925031E-16));
#20960=CARTESIAN_POINT('Ctrl Pts',(-207.22920174438,93.1436360359813,-3.34315983412545E-16));
#20961=CARTESIAN_POINT('Ctrl Pts',(-207.171876621466,93.0635500123343,3.41627951812914E-16));
#20962=CARTESIAN_POINT('Ctrl Pts',(-207.11069968939,92.9862376762064,4.44089209850063E-16));
#20963=CARTESIAN_POINT('Ctrl Pts',(-207.086606803213,92.955790295941,4.8444081532694E-16));
#20964=CARTESIAN_POINT('Ctrl Pts',(-207.061915990083,92.9257733393162,2.50658725338041E-16));
#20965=CARTESIAN_POINT('Ctrl Pts',(-207.036642028582,92.896205321917,2.4980018054066E-16));
#20966=CARTESIAN_POINT('Ctrl Pts',(-207.022295011884,92.8794207414964,2.49312819010743E-16));
#20967=CARTESIAN_POINT('Ctrl Pts',(-207.007760063825,92.8627808390425,4.63072277927187E-16));
#20968=CARTESIAN_POINT('Ctrl Pts',(-206.993039745212,92.8462891116921,4.71844785465692E-16));
#20969=CARTESIAN_POINT('Ctrl Pts',(-206.979027736376,92.8305909304621,4.80195178984602E-16));
#20970=CARTESIAN_POINT('Ctrl Pts',(-206.964844946112,92.8150241309821,9.01246990176946E-16));
#20971=CARTESIAN_POINT('Ctrl Pts',(-206.950512567364,92.7996118404543,8.60422844084496E-16));
#20972=CARTESIAN_POINT('Ctrl Pts',(-206.881794961135,92.7257165206168,6.64688580759402E-16));
#20973=CARTESIAN_POINT('Ctrl Pts',(-206.809566114702,92.655283034501,1.95353569017064E-16));
#20974=CARTESIAN_POINT('Ctrl Pts',(-206.734139541689,92.5885980814127,2.22044604925031E-16));
#20975=CARTESIAN_POINT('Ctrl Pts',(-206.669026438941,92.5310313111255,2.45086035737897E-16));
#20976=CARTESIAN_POINT('Ctrl Pts',(-206.601529266805,92.4762579626061,-8.3008266997134E-17));
#20977=CARTESIAN_POINT('Ctrl Pts',(-206.531823161522,92.42447802842,-1.66533453693773E-16));
#20978=CARTESIAN_POINT('Ctrl Pts',(-206.504658151372,92.4042989862542,-1.99083867106794E-16));
#20979=CARTESIAN_POINT('Ctrl Pts',(-206.477157425522,92.384574749707,2.57352051279242E-16));
#20980=CARTESIAN_POINT('Ctrl Pts',(-206.449330482091,92.3653179595526,2.77555756156289E-16));
#20981=CARTESIAN_POINT('Ctrl Pts',(-206.434060293588,92.3547506898726,2.88642650506663E-16));
#20982=CARTESIAN_POINT('Ctrl Pts',(-206.4186931394,92.344325166916,5.01730169144111E-17));
#20983=CARTESIAN_POINT('Ctrl Pts',(-206.403240754609,92.3340499669156,5.55111512312578E-17));
#20984=CARTESIAN_POINT('Ctrl Pts',(-206.316661516034,92.2764783361116,8.54205542659342E-17));
#20985=CARTESIAN_POINT('Ctrl Pts',(-206.227325727871,92.2235642261423,1.65945870128525E-16));
#20986=CARTESIAN_POINT('Ctrl Pts',(-206.135543256089,92.1756305450252,5.55111512312578E-17));
#20987=CARTESIAN_POINT('Ctrl Pts',(-206.043760784307,92.1276968639081,-5.49235676660085E-17));
#20988=CARTESIAN_POINT('Ctrl Pts',(-205.949530976973,92.0847426931351,-5.98436115446713E-17));
#20989=CARTESIAN_POINT('Ctrl Pts',(-205.853125481029,92.0471321793771,-2.22044604925031E-16));
#20990=CARTESIAN_POINT('Ctrl Pts',(-205.834025098342,92.03968057925,-2.54180750436268E-16));
#20991=CARTESIAN_POINT('Ctrl Pts',(-205.814839209604,92.0324388923413,-1.04868572471002E-16));
#20992=CARTESIAN_POINT('Ctrl Pts',(-205.79557093555,92.025406175614,-1.11022302462516E-16));
#20993=CARTESIAN_POINT('Ctrl Pts',(-202.480282650156,94.9980775783256,1.61258330249198));
#20994=CARTESIAN_POINT('Ctrl Pts',(-202.479237247099,94.8744698806693,1.60474993100901));
#20995=CARTESIAN_POINT('Ctrl Pts',(-202.487545284979,94.7510033134378,1.59691655952604));
#20996=CARTESIAN_POINT('Ctrl Pts',(-202.505691786454,94.6290001821137,1.58908318804307));
#20997=CARTESIAN_POINT('Ctrl Pts',(-202.628398850194,93.8040121791943,1.53611374844163));
#20998=CARTESIAN_POINT('Ctrl Pts',(-203.200969244479,93.0459397210627,1.4831443088402));
#20999=CARTESIAN_POINT('Ctrl Pts',(-203.960941731557,92.702270111656,1.43017486923876));
#21000=CARTESIAN_POINT('Ctrl Pts',(-204.720914218634,92.3586005022492,1.37720542963732));
#21001=CARTESIAN_POINT('Ctrl Pts',(-205.668288798503,92.4293337415673,1.32423599003589));
#21002=CARTESIAN_POINT('Ctrl Pts',(-206.368790472088,92.8820644553757,1.27126655043445));
#21003=CARTESIAN_POINT('Ctrl Pts',(-207.069292145673,93.3347951691841,1.21829711083302));
#21004=CARTESIAN_POINT('Ctrl Pts',(-207.522920912975,94.1695233574828,1.16532767123158));
#21005=CARTESIAN_POINT('Ctrl Pts',(-207.521743709329,95.0035763514476,1.11235823163015));
#21006=CARTESIAN_POINT('Ctrl Pts',(-207.520566505683,95.8376293454124,1.05938879202871));
#21007=CARTESIAN_POINT('Ctrl Pts',(-207.064583331089,96.6710071450434,1.00641935242728));
#21008=CARTESIAN_POINT('Ctrl Pts',(-206.362798141834,97.1217724460714,0.95344991282584));
#21009=CARTESIAN_POINT('Ctrl Pts',(-205.661012952578,97.5725377470994,0.900480473224404));
#21010=CARTESIAN_POINT('Ctrl Pts',(-204.713425748661,97.6406905495243,0.847511033622969));
#21011=CARTESIAN_POINT('Ctrl Pts',(-203.954438657476,97.2948278472581,0.794541594021534));
#21012=CARTESIAN_POINT('Ctrl Pts',(-203.195451566291,96.9489651449919,0.741572154420098));
#21013=CARTESIAN_POINT('Ctrl Pts',(-202.625064587839,96.1890869380346,0.688602714818662));
#21014=CARTESIAN_POINT('Ctrl Pts',(-202.504670688411,95.3638523156723,0.635633275217227));
#21015=CARTESIAN_POINT('Ctrl Pts',(-202.487207310037,95.2441503662684,0.627949950975477));
#21016=CARTESIAN_POINT('Ctrl Pts',(-202.479211825944,95.1230733120894,0.620266626733727));
#21017=CARTESIAN_POINT('Ctrl Pts',(-202.480223566112,95.0018649480296,0.612583302491977));
#21018=CARTESIAN_POINT('Ctrl Pts',(-204.206200717467,92.0307770462543,-1.66533453693773E-15));
#21019=CARTESIAN_POINT('Ctrl Pts',(-203.217993421758,92.294966786987,0.0529694396014339));
#21020=CARTESIAN_POINT('Ctrl Pts',(-201.543538204128,93.8848222016534,0.158908318804305));
#21021=CARTESIAN_POINT('Ctrl Pts',(-202.189751811533,97.3070700667118,0.317816637608612));
#21022=CARTESIAN_POINT('Ctrl Pts',(-205.417647311761,98.6092821234889,0.476724956412918));
#21023=CARTESIAN_POINT('Ctrl Pts',(-208.260128930045,96.6049848945777,0.635633275217225));
#21024=CARTESIAN_POINT('Ctrl Pts',(-208.114979909401,93.1280855192232,0.794541594021532));
#21025=CARTESIAN_POINT('Ctrl Pts',(-205.113462578231,91.3679026833885,0.953449912825839));
#21026=CARTESIAN_POINT('Ctrl Pts',(-202.008209188913,92.9373122193729,1.11235823163015));
#21027=CARTESIAN_POINT('Ctrl Pts',(-201.645658243496,96.3979033225417,1.27126655043445));
#21028=CARTESIAN_POINT('Ctrl Pts',(-204.35839704753,98.5768482113765,1.43017486923876));
#21029=CARTESIAN_POINT('Ctrl Pts',(-207.659317996079,97.4766096293226,1.58908318804307));
#21030=CARTESIAN_POINT('Ctrl Pts',(-208.522221537982,94.105828029106,1.74799150684737));
#21031=CARTESIAN_POINT('Ctrl Pts',(-206.155984190728,91.5548205487187,1.90689982565168));
#21032=CARTESIAN_POINT('Ctrl Pts',(-202.729957109659,92.1623115759729,2.06580814445599));
#21033=CARTESIAN_POINT('Ctrl Pts',(-201.385078212169,95.371365330558,2.22471646326029));
#21034=CARTESIAN_POINT('Ctrl Pts',(-203.354320060973,98.2399546801978,2.3836247820646));
#21035=CARTESIAN_POINT('Ctrl Pts',(-206.832302471161,98.13819018824,2.54253310086891));
#21036=CARTESIAN_POINT('Ctrl Pts',(-208.630450654962,95.1593678146252,2.70144141967321));
#21037=CARTESIAN_POINT('Ctrl Pts',(-207.100242158396,92.0344389026441,2.86034973847752));
#21038=CARTESIAN_POINT('Ctrl Pts',(-203.644555171756,91.6283032143389,3.01925805728183));
#21039=CARTESIAN_POINT('Ctrl Pts',(-201.4315248315,94.3133014760961,3.17816637608613));
#21040=CARTESIAN_POINT('Ctrl Pts',(-202.490032652559,97.6278572589721,3.33707469489044));
#21041=CARTESIAN_POINT('Ctrl Pts',(-205.849650479072,98.5332228829228,3.49598301369474));
#21042=CARTESIAN_POINT('Ctrl Pts',(-208.430318245301,96.1993692554529,3.65489133249905));
#21043=CARTESIAN_POINT('Ctrl Pts',(-207.866108582956,92.7659473008752,3.81379965130336));
#21044=CARTESIAN_POINT('Ctrl Pts',(-204.67428260626,91.3806798907347,3.97270797010767));
#21045=CARTESIAN_POINT('Ctrl Pts',(-201.781070695379,93.3135647046544,4.13161628891197));
#21046=CARTESIAN_POINT('Ctrl Pts',(-201.838937193807,96.7925545482736,4.29052460771628));
#21047=CARTESIAN_POINT('Ctrl Pts',(-204.79483074234,98.6281504171124,4.44943292652058));
#21048=CARTESIAN_POINT('Ctrl Pts',(-207.938821173194,97.1374985345979,4.60834124532489));
#21049=CARTESIAN_POINT('Ctrl Pts',(-208.388533199045,93.6872118859588,4.76724956412919));
#21050=CARTESIAN_POINT('Ctrl Pts',(-205.731675860954,91.4404747075036,4.92615788293351));
#21051=CARTESIAN_POINT('Ctrl Pts',(-202.404026271327,92.4570705331348,5.08506620173781));
#21052=CARTESIAN_POINT('Ctrl Pts',(-201.456336381487,95.8049956721891,5.24397452054212));
#21053=CARTESIAN_POINT('Ctrl Pts',(-203.757437690304,98.4149097762516,5.40288283934642));
#21054=CARTESIAN_POINT('Ctrl Pts',(-207.197706236788,97.8940727651868,5.56179115815073));
#21055=CARTESIAN_POINT('Ctrl Pts',(-208.623142268693,94.7199821894518,5.72069947695504));
#21056=CARTESIAN_POINT('Ctrl Pts',(-206.726921963772,91.8026088127262,5.87960779575934));
#21057=CARTESIAN_POINT('Ctrl Pts',(-203.247478903914,91.8165679399129,6.03851611456365));
#21058=CARTESIAN_POINT('Ctrl Pts',(-201.374727597382,94.7490619992257,6.19742443336796));
#21059=CARTESIAN_POINT('Ctrl Pts',(-202.82558551065,97.9116132129659,6.35633275217227));
#21060=CARTESIAN_POINT('Ctrl Pts',(-206.269922324772,98.4048299755582,6.51524107097657));
#21061=CARTESIAN_POINT('Ctrl Pts',(-208.550008545203,95.7765366716391,6.67414938978089));
#21062=CARTESIAN_POINT('Ctrl Pts',(-207.575486609103,92.4363232263514,6.83305770858518));
#21063=CARTESIAN_POINT('Ctrl Pts',(-204.239787335459,91.4464599934592,6.9919660273895));
#21064=CARTESIAN_POINT('Ctrl Pts',(-201.601042535926,93.7144425213819,7.1508743461938));
#21065=CARTESIAN_POINT('Ctrl Pts',(-202.078423950012,97.1610097772913,7.30978266499811));
#21066=CARTESIAN_POINT('Ctrl Pts',(-205.234273632875,98.6263874225397,7.46869098380241));
#21067=CARTESIAN_POINT('Ctrl Pts',(-208.175343867546,96.7671336101861,7.62759930260672));
#21068=CARTESIAN_POINT('Ctrl Pts',(-208.205294334613,93.2877914549009,7.78650762141103));
#21069=CARTESIAN_POINT('Ctrl Pts',(-205.296666780619,91.3781829567617,7.94541594021533));
#21070=CARTESIAN_POINT('Ctrl Pts',(-202.116058437936,92.789015843563,8.10432425901964));
#21071=CARTESIAN_POINT('Ctrl Pts',(-201.579415486135,96.2268542932731,8.26323257782395));
#21072=CARTESIAN_POINT('Ctrl Pts',(-204.17872618548,98.5399264392071,8.42214089662825));
#21073=CARTESIAN_POINT('Ctrl Pts',(-207.530971538769,97.6076335907019,8.58104921543256));
#21074=CARTESIAN_POINT('Ctrl Pts',(-208.56285047346,94.2846914112228,8.73995753423687));
#21075=CARTESIAN_POINT('Ctrl Pts',(-206.328347915327,91.6175361510784,8.89886585304118));
#21076=CARTESIAN_POINT('Ctrl Pts',(-202.876030835092,92.0513859425261,9.05777417184547));
#21077=CARTESIAN_POINT('Ctrl Pts',(-201.37094494608,95.1884921458163,9.2166824906498));
#21078=CARTESIAN_POINT('Ctrl Pts',(-203.192936169305,98.1527908565597,9.37559080945409));
#21079=CARTESIAN_POINT('Ctrl Pts',(-206.671623315332,98.2266461481009,9.5344991282584));
#21080=CARTESIAN_POINT('Ctrl Pts',(-208.617784889251,95.3423483146199,9.6934074470627));
#21081=CARTESIAN_POINT('Ctrl Pts',(-207.247201711938,92.1441893726518,9.85231576586701));
#21082=CARTESIAN_POINT('Ctrl Pts',(-203.81640912163,91.5642056950316,10.0112240846713));
#21083=CARTESIAN_POINT('Ctrl Pts',(-201.47071941986,94.1341198350438,10.1701324034756));
#21084=CARTESIAN_POINT('Ctrl Pts',(-202.360634707924,97.4978632325243,10.3290407222799));
#21085=CARTESIAN_POINT('Ctrl Pts',(-205.670290596122,98.5715935365275,10.4879490410842));
#21086=CARTESIAN_POINT('Ctrl Pts',(-208.365431557495,96.3709268052048,10.6468573598885));
#21087=CARTESIAN_POINT('Ctrl Pts',(-207.975182481689,92.9134097014358,10.8057656786928));
#21088=CARTESIAN_POINT('Ctrl Pts',(-204.85731935967,91.3688552620022,10.9646739974972));
#21089=CARTESIAN_POINT('Ctrl Pts',(-201.870264253993,93.153293733811,11.1235823163015));
#21090=CARTESIAN_POINT('Ctrl Pts',(-201.752515899846,96.6307718702076,11.2824906351058));
#21091=CARTESIAN_POINT('Ctrl Pts',(-204.612024672262,98.6131765827982,11.4413989539101));
#21092=CARTESIAN_POINT('Ctrl Pts',(-207.827224888828,97.2830613880067,11.6003072727144));
#21093=CARTESIAN_POINT('Ctrl Pts',(-208.450456926625,93.8598610299961,11.7592155915187));
#21094=CARTESIAN_POINT('Ctrl Pts',(-205.910348619136,91.4819273365871,11.918123910323));
#21095=CARTESIAN_POINT('Ctrl Pts',(-202.535642872402,92.3293233402249,12.0770322291273));
#21096=CARTESIAN_POINT('Ctrl Pts',(-201.420232196639,95.6251658559424,12.2359405479316));
#21097=CARTESIAN_POINT('Ctrl Pts',(-203.586712632674,98.3478633022839,12.3948488667359));
#21098=CARTESIAN_POINT('Ctrl Pts',(-207.048879131051,98.0012770914624,12.5537571855402));
#21099=CARTESIAN_POINT('Ctrl Pts',(-208.632656141981,94.9031535878521,12.7126655043445));
#21100=CARTESIAN_POINT('Ctrl Pts',(-206.886054603385,91.8938177924453,12.8715738231489));
#21101=CARTESIAN_POINT('Ctrl Pts',(-203.410339284457,91.7321951278126,13.0304821419532));
#21102=CARTESIAN_POINT('Ctrl Pts',(-201.39200714221,94.56645944633,13.1893904607574));
#21103=CARTESIAN_POINT('Ctrl Pts',(-202.681442526234,97.7981888990492,13.3482987795618));
#21104=CARTESIAN_POINT('Ctrl Pts',(-206.096505488088,98.4645700435054,13.5072070983661));
#21105=CARTESIAN_POINT('Ctrl Pts',(-208.506304474045,95.9546720956722,13.6661154171704));
#21106=CARTESIAN_POINT('Ctrl Pts',(-207.701562707091,92.569541439018,13.8250237359747));
#21107=CARTESIAN_POINT('Ctrl Pts',(-204.420058445801,91.4126280298156,13.983932054779));
#21108=CARTESIAN_POINT('Ctrl Pts',(-201.670238118031,93.5445771403762,14.1428403735833));
#21109=CARTESIAN_POINT('Ctrl Pts',(-201.973106270655,97.0108416765384,14.3017486923876));
#21110=CARTESIAN_POINT('Ctrl Pts',(-205.05099675704,98.6335890076928,14.4606570111919));
#21111=CARTESIAN_POINT('Ctrl Pts',(-208.082133999653,96.9251026119764,14.6195653299962));
#21112=CARTESIAN_POINT('Ctrl Pts',(-208.287605212672,93.451703526775,14.7784736488005));
#21113=CARTESIAN_POINT('Ctrl Pts',(-205.479036767596,91.3977656146854,14.9373819676048));
#21114=CARTESIAN_POINT('Ctrl Pts',(-202.231292652311,92.6463153644278,15.0962902864091));
#21115=CARTESIAN_POINT('Ctrl Pts',(-201.521868727466,96.0526980416367,15.2551986052134));
#21116=CARTESIAN_POINT('Ctrl Pts',(-204.001156184096,98.4939765214113,15.4141069240178));
#21117=CARTESIAN_POINT('Ctrl Pts',(-207.396173510293,97.7320213368001,15.573015242822));
#21118=CARTESIAN_POINT('Ctrl Pts',(-208.594403628795,94.4653692735856,15.7319235616264));
#21119=CARTESIAN_POINT('Ctrl Pts',(-206.497329046882,91.688881880511,15.8908318804307));
#21120=CARTESIAN_POINT('Ctrl Pts',(-203.027510890261,91.9479467516828,16.049740199235));
#21121=CARTESIAN_POINT('Ctrl Pts',(-201.366067392462,95.0051905226268,16.2086485180393));
#21122=CARTESIAN_POINT('Ctrl Pts',(-203.036134055811,98.0574883854641,16.3675568368436));
#21123=CARTESIAN_POINT('Ctrl Pts',(-206.506730950831,98.3071022816236,16.5264651556479));
#21124=CARTESIAN_POINT('Ctrl Pts',(-208.595808661615,95.5240011654517,16.6853734744522));
#21125=CARTESIAN_POINT('Ctrl Pts',(-207.388631166444,92.2621563458355,16.8442817932565));
#21126=CARTESIAN_POINT('Ctrl Pts',(-203.990889239491,91.5068978476827,17.0031901120608));
#21127=CARTESIAN_POINT('Ctrl Pts',(-201.519840110817,93.9611367684014,17.1620984308651));
#21128=CARTESIAN_POINT('Ctrl Pts',(-201.999201820237,96.219820647773,17.268037310068));
#21129=CARTESIAN_POINT('Ctrl Pts',(-202.663937342304,96.9973015569306,17.3210067496694));
#21130=CARTESIAN_POINT('Ctrl Pts',(-204.254067145653,92.2098224301578,-0.107002249889812));
#21131=CARTESIAN_POINT('Ctrl Pts',(-203.325449162499,92.4580814192125,-0.0540328102883767));
#21132=CARTESIAN_POINT('Ctrl Pts',(-201.751964293657,93.9520678885337,0.0519060689144946));
#21133=CARTESIAN_POINT('Ctrl Pts',(-202.359210950711,97.1679527783771,0.210814387718801));
#21134=CARTESIAN_POINT('Ctrl Pts',(-205.392463004474,98.3916409043943,0.369722706523108));
#21135=CARTESIAN_POINT('Ctrl Pts',(-208.063541794304,96.5082036352768,0.528631025327414));
#21136=CARTESIAN_POINT('Ctrl Pts',(-207.927145320211,93.2409627440279,0.687539344131721));
#21137=CARTESIAN_POINT('Ctrl Pts',(-205.106620737387,91.5869196681547,0.846447662936027));
#21138=CARTESIAN_POINT('Ctrl Pts',(-202.188615424038,93.0616931538156,1.00535598174034));
#21139=CARTESIAN_POINT('Ctrl Pts',(-201.847926452011,96.3136091685009,1.16426430054464));
#21140=CARTESIAN_POINT('Ctrl Pts',(-204.397085973464,98.3611627707252,1.32317261934895));
#21141=CARTESIAN_POINT('Ctrl Pts',(-207.498960010523,97.3272690345715,1.48208093815326));
#21142=CARTESIAN_POINT('Ctrl Pts',(-208.309830108546,94.1597469723104,1.64098925695756));
#21143=CARTESIAN_POINT('Ctrl Pts',(-206.086277861348,91.7625663081583,1.79989757576187));
#21144=CARTESIAN_POINT('Ctrl Pts',(-202.866841643798,92.3334253728125,1.95880589456617));
#21145=CARTESIAN_POINT('Ctrl Pts',(-201.603059505378,95.3489718460626,2.11771421337048));
#21146=CARTESIAN_POINT('Ctrl Pts',(-203.453555248447,98.0445840601458,2.27662253217479));
#21147=CARTESIAN_POINT('Ctrl Pts',(-206.721813867076,97.9489560095445,2.43553085097909));
#21148=CARTESIAN_POINT('Ctrl Pts',(-208.411532964581,95.1497578688597,2.5944391697834));
#21149=CARTESIAN_POINT('Ctrl Pts',(-206.973596679293,92.2132634750782,2.75334748858771));
#21150=CARTESIAN_POINT('Ctrl Pts',(-203.726289060862,91.8316179383591,2.91225580739202));
#21151=CARTESIAN_POINT('Ctrl Pts',(-201.64670537417,94.354709683817,3.07116412619632));
#21152=CARTESIAN_POINT('Ctrl Pts',(-202.641384731641,97.469396369,3.23007244500063));
#21153=CARTESIAN_POINT('Ctrl Pts',(-205.798416200415,98.3201680677929,3.38898076380494));
#21154=CARTESIAN_POINT('Ctrl Pts',(-208.223468622787,96.1270467885551,3.54788908260924));
#21155=CARTESIAN_POINT('Ctrl Pts',(-207.693281038666,92.9006616114564,3.70679740141355));
#21156=CARTESIAN_POINT('Ctrl Pts',(-204.693923501105,91.5989264045628,3.86570572021786));
#21157=CARTESIAN_POINT('Ctrl Pts',(-201.975173476504,93.4152574571311,4.02461403902216));
#21158=CARTESIAN_POINT('Ctrl Pts',(-202.029550600916,96.6844627605355,4.18352235782647));
#21159=CARTESIAN_POINT('Ctrl Pts',(-204.807202534245,98.4093714320339,4.34243067663077));
#21160=CARTESIAN_POINT('Ctrl Pts',(-207.761609029352,97.0086064804539,4.50133899543508));
#21161=CARTESIAN_POINT('Ctrl Pts',(-208.184203232267,93.7663735573872,4.66024731423939));
#21162=CARTESIAN_POINT('Ctrl Pts',(-205.687555501028,91.6551155689135,4.81915563304369));
#21163=CARTESIAN_POINT('Ctrl Pts',(-202.560564571109,92.6104102417814,4.978063951848));
#21164=CARTESIAN_POINT('Ctrl Pts',(-201.670020777333,95.7564540970319,5.13697227065231));
#21165=CARTESIAN_POINT('Ctrl Pts',(-203.832364716408,98.2089892908554,5.29588058945662));
#21166=CARTESIAN_POINT('Ctrl Pts',(-207.065183633062,97.7195589690321,5.45478890826092));
#21167=CARTESIAN_POINT('Ctrl Pts',(-208.404665277056,94.7368673803487,5.61369722706523));
#21168=CARTESIAN_POINT('Ctrl Pts',(-206.622787848284,91.9954128363827,5.77260554586954));
#21169=CARTESIAN_POINT('Ctrl Pts',(-203.35315665777,92.0085302223715,5.93151386467384));
#21170=CARTESIAN_POINT('Ctrl Pts',(-201.593333036985,94.7641936654509,6.09042218347815));
#21171=CARTESIAN_POINT('Ctrl Pts',(-202.95670361228,97.7360417204863,6.24933050228246));
#21172=CARTESIAN_POINT('Ctrl Pts',(-206.193345478335,98.1995173063525,6.40823882108676));
#21173=CARTESIAN_POINT('Ctrl Pts',(-208.335941547629,95.7297111860981,6.56714713989107));
#21174=CARTESIAN_POINT('Ctrl Pts',(-207.420183691185,92.59091400626,6.72605545869537));
#21175=CARTESIAN_POINT('Ctrl Pts',(-204.285628476556,91.6607399396267,6.88496377749968));
#21176=CARTESIAN_POINT('Ctrl Pts',(-201.806001090237,93.7919621741243,7.04387209630399));
#21177=CARTESIAN_POINT('Ctrl Pts',(-202.254596205724,97.0306999853957,7.2027804151083));
#21178=CARTESIAN_POINT('Ctrl Pts',(-205.220146834992,98.4077147467702,7.3616887339126));
#21179=CARTESIAN_POINT('Ctrl Pts',(-207.983869306475,96.6605747156291,7.52059705271691));
#21180=CARTESIAN_POINT('Ctrl Pts',(-208.012013747872,93.3910383450994,7.67950537152122));
#21181=CARTESIAN_POINT('Ctrl Pts',(-205.278777649875,91.5965800367509,7.83841369032552));
#21182=CARTESIAN_POINT('Ctrl Pts',(-202.289961318312,92.9223391113879,7.99732200912983));
#21183=CARTESIAN_POINT('Ctrl Pts',(-201.785678160579,96.1528744671184,8.15623032793414));
#21184=CARTESIAN_POINT('Ctrl Pts',(-204.228249339416,98.3264673968342,8.31513864673844));
#21185=CARTESIAN_POINT('Ctrl Pts',(-207.378352898179,97.4503921963708,8.47404696554275));
#21186=CARTESIAN_POINT('Ctrl Pts',(-208.34800910225,94.3278248178017,8.63295528434706));
#21187=CARTESIAN_POINT('Ctrl Pts',(-206.248247981384,91.8215001335089,8.79186360315136));
#21188=CARTESIAN_POINT('Ctrl Pts',(-203.004107062594,92.2291886013793,8.95077192195567));
#21189=CARTESIAN_POINT('Ctrl Pts',(-201.589778481136,95.1771259907191,9.10968024075998));
#21190=CARTESIAN_POINT('Ctrl Pts',(-203.301902872831,97.9626762514681,9.26858855956428));
#21191=CARTESIAN_POINT('Ctrl Pts',(-206.570823731434,98.0320780380912,9.42749687836859));
#21192=CARTESIAN_POINT('Ctrl Pts',(-208.399630949831,95.3217045683015,9.5864051971729));
#21193=CARTESIAN_POINT('Ctrl Pts',(-207.111694510394,92.3163959459186,9.7453135159772));
#21194=CARTESIAN_POINT('Ctrl Pts',(-203.887780145802,91.7713855262297,9.90422183478152));
#21195=CARTESIAN_POINT('Ctrl Pts',(-201.683536512486,94.1863327705371,10.0631301535858));
#21196=CARTESIAN_POINT('Ctrl Pts',(-202.519789537097,97.3472410366256,10.2220384723901));
#21197=CARTESIAN_POINT('Ctrl Pts',(-205.629871793297,98.3562249549636,10.3809467911944));
#21198=CARTESIAN_POINT('Ctrl Pts',(-208.16249462935,96.2882593464234,10.5398551099987));
#21199=CARTESIAN_POINT('Ctrl Pts',(-207.795777735762,93.0392319676905,10.698763428803));
#21200=CARTESIAN_POINT('Ctrl Pts',(-204.865923061858,91.5878148058802,10.8576717476073));
#21201=CARTESIAN_POINT('Ctrl Pts',(-202.058988626292,93.2646508927504,11.0165800664117));
#21202=CARTESIAN_POINT('Ctrl Pts',(-201.948340547065,96.5324356455089,11.175488385216));
#21203=CARTESIAN_POINT('Ctrl Pts',(-204.635419746522,98.3953005261812,11.3343967040203));
#21204=CARTESIAN_POINT('Ctrl Pts',(-207.65674204753,97.1453918330226,11.4933050228246));
#21205=CARTESIAN_POINT('Ctrl Pts',(-208.242392933218,93.9286118859498,11.6522133416289));
#21206=CARTESIAN_POINT('Ctrl Pts',(-205.855454217288,91.6940685871547,11.8111216604332));
#21207=CARTESIAN_POINT('Ctrl Pts',(-202.684244636183,92.4903662579446,11.9700299792375));
#21208=CARTESIAN_POINT('Ctrl Pts',(-201.636093689906,95.5874680937925,12.1289382980418));
#21209=CARTESIAN_POINT('Ctrl Pts',(-203.671934451039,98.145985747263,12.2878466168461));
#21210=CARTESIAN_POINT('Ctrl Pts',(-206.925330863944,97.8202988296705,12.4467549356504));
#21211=CARTESIAN_POINT('Ctrl Pts',(-208.413605459812,94.9089934669425,12.6056632544547));
#21212=CARTESIAN_POINT('Ctrl Pts',(-206.772324723283,92.0811218765405,12.764571573259));
#21213=CARTESIAN_POINT('Ctrl Pts',(-203.506196489364,91.9292451260705,12.9234798920633));
#21214=CARTESIAN_POINT('Ctrl Pts',(-201.609570618045,94.5926021227402,13.0823882108676));
#21215=CARTESIAN_POINT('Ctrl Pts',(-202.821252510011,97.6294569400588,13.241296529672));
#21216=CARTESIAN_POINT('Ctrl Pts',(-206.030385749313,98.2556550232583,13.4002048484762));
#21217=CARTESIAN_POINT('Ctrl Pts',(-208.29487285021,95.8971049696819,13.5591131672806));
#21218=CARTESIAN_POINT('Ctrl Pts',(-207.538657347822,92.7160991050779,13.7180214860849));
#21219=CARTESIAN_POINT('Ctrl Pts',(-204.455029163672,91.6289480575171,13.8769298048892));
#21220=CARTESIAN_POINT('Ctrl Pts',(-201.871024149848,93.6323397465202,14.0358381236935));
#21221=CARTESIAN_POINT('Ctrl Pts',(-202.155629226407,96.8895870838205,14.1947464424978));
#21222=CARTESIAN_POINT('Ctrl Pts',(-205.047921631297,98.4144820733316,14.3536547613021));
#21223=CARTESIAN_POINT('Ctrl Pts',(-207.896280032535,96.8090181206517,14.5125630801064));
#21224=CARTESIAN_POINT('Ctrl Pts',(-208.089361245615,93.5450664505984,14.6714713989107));
#21225=CARTESIAN_POINT('Ctrl Pts',(-205.450150650489,91.6149818522251,14.830379717715));
#21226=CARTESIAN_POINT('Ctrl Pts',(-202.398246861444,92.7882435307288,14.9892880365193));
#21227=CARTESIAN_POINT('Ctrl Pts',(-201.731601495486,95.9892199101742,15.1481963553236));
#21228=CARTESIAN_POINT('Ctrl Pts',(-204.06138688326,98.2832882782678,15.3071046741279));
#21229=CARTESIAN_POINT('Ctrl Pts',(-207.251683247105,97.5672793094413,15.4660129929322));
#21230=CARTESIAN_POINT('Ctrl Pts',(-208.377659589143,94.4976077296224,15.6249213117366));
#21231=CARTESIAN_POINT('Ctrl Pts',(-206.407039480148,91.8885436856663,15.7838296305408));
#21232=CARTESIAN_POINT('Ctrl Pts',(-203.146452807187,92.1319868369347,15.9427379493452));
#21233=CARTESIAN_POINT('Ctrl Pts',(-201.585195046037,95.0048775319451,16.1016462681495));
#21234=CARTESIAN_POINT('Ctrl Pts',(-203.154555992253,97.8731205591728,16.2605545869538));
#21235=CARTESIAN_POINT('Ctrl Pts',(-206.415874445363,98.1076826331683,16.4194629057581));
#21236=CARTESIAN_POINT('Ctrl Pts',(-208.378979897898,95.4924036763794,16.5783712245624));
#21237=CARTESIAN_POINT('Ctrl Pts',(-207.24459570974,92.4272494613622,16.7372795433667));
#21238=CARTESIAN_POINT('Ctrl Pts',(-204.051739039702,91.7175333660049,16.896187862171));
#21239=CARTESIAN_POINT('Ctrl Pts',(-201.729695205268,94.0237806550419,17.0550961809753));
#21240=CARTESIAN_POINT('Ctrl Pts',(-202.180151203454,96.1462649533788,17.1610350601782));
#21241=CARTESIAN_POINT('Ctrl Pts',(-202.804802895981,96.8768634390787,17.2140044997796));
#21242=CARTESIAN_POINT('Ctrl Pts',(-204.301933573839,92.3888678140614,-0.214004499779623));
#21243=CARTESIAN_POINT('Ctrl Pts',(-203.43290490324,92.6211960514381,-0.161035060178187));
#21244=CARTESIAN_POINT('Ctrl Pts',(-201.960390383187,94.0193135754141,-0.0550961809753161));
#21245=CARTESIAN_POINT('Ctrl Pts',(-202.528670089889,97.0288354900421,0.103812137828991));
#21246=CARTESIAN_POINT('Ctrl Pts',(-205.367278697187,98.1739996853001,0.262720456633297));
#21247=CARTESIAN_POINT('Ctrl Pts',(-207.866954658562,96.4114223759756,0.421628775437604));
#21248=CARTESIAN_POINT('Ctrl Pts',(-207.73931073102,93.3538399688327,0.58053709424191));
#21249=CARTESIAN_POINT('Ctrl Pts',(-205.099778896544,91.8059366529208,0.739445413046218));
#21250=CARTESIAN_POINT('Ctrl Pts',(-202.369021659162,93.1860740882583,0.898353731850525));
#21251=CARTESIAN_POINT('Ctrl Pts',(-202.050194660526,96.2293150144601,1.05726205065483));
#21252=CARTESIAN_POINT('Ctrl Pts',(-204.435774899398,98.1454773300738,1.21617036945914));
#21253=CARTESIAN_POINT('Ctrl Pts',(-207.338602024967,97.1779284398204,1.37507868826344));
#21254=CARTESIAN_POINT('Ctrl Pts',(-208.09743867911,94.2136659155149,1.53398700706775));
#21255=CARTESIAN_POINT('Ctrl Pts',(-206.016571531969,91.9703120675979,1.69289532587206));
#21256=CARTESIAN_POINT('Ctrl Pts',(-203.003726177937,92.504539169652,1.85180364467636));
#21257=CARTESIAN_POINT('Ctrl Pts',(-201.821040798587,95.3265783615671,2.01071196348067));
#21258=CARTESIAN_POINT('Ctrl Pts',(-203.55279043592,97.8492134400937,2.16962028228498));
#21259=CARTESIAN_POINT('Ctrl Pts',(-206.611325262991,97.7597218308491,2.32852860108929));
#21260=CARTESIAN_POINT('Ctrl Pts',(-208.1926152742,95.1401479230941,2.48743691989359));
#21261=CARTESIAN_POINT('Ctrl Pts',(-206.84695120019,92.3920880475125,2.6463452386979));
#21262=CARTESIAN_POINT('Ctrl Pts',(-203.808022949968,92.0349326623793,2.80525355750221));
#21263=CARTESIAN_POINT('Ctrl Pts',(-201.86188591684,94.3961178915378,2.96416187630651));
#21264=CARTESIAN_POINT('Ctrl Pts',(-202.792736810723,97.3109354790277,3.12307019511082));
#21265=CARTESIAN_POINT('Ctrl Pts',(-205.747181921757,98.1071132526631,3.28197851391513));
#21266=CARTESIAN_POINT('Ctrl Pts',(-208.016619000273,96.0547243216571,3.44088683271943));
#21267=CARTESIAN_POINT('Ctrl Pts',(-207.520453494377,93.0353759220375,3.59979515152374));
#21268=CARTESIAN_POINT('Ctrl Pts',(-204.71356439595,91.8171729183909,3.75870347032804));
#21269=CARTESIAN_POINT('Ctrl Pts',(-202.16927625763,93.5169502096079,3.91761178913235));
#21270=CARTESIAN_POINT('Ctrl Pts',(-202.220164008024,96.5763709727973,4.07652010793666));
#21271=CARTESIAN_POINT('Ctrl Pts',(-204.81957432615,98.1905924469556,4.23542842674096));
#21272=CARTESIAN_POINT('Ctrl Pts',(-207.58439688551,96.8797144263097,4.39433674554527));
#21273=CARTESIAN_POINT('Ctrl Pts',(-207.97987326549,93.8455352288158,4.55324506434958));
#21274=CARTESIAN_POINT('Ctrl Pts',(-205.643435141103,91.8697564303231,4.71215338315388));
#21275=CARTESIAN_POINT('Ctrl Pts',(-202.717102870891,92.7637499504281,4.87106170195819));
#21276=CARTESIAN_POINT('Ctrl Pts',(-201.883705173178,95.7079125218746,5.0299700207625));
#21277=CARTESIAN_POINT('Ctrl Pts',(-203.907291742512,98.0030688054592,5.18887833956681));
#21278=CARTESIAN_POINT('Ctrl Pts',(-206.932661029337,97.5450451728775,5.34778665837111));
#21279=CARTESIAN_POINT('Ctrl Pts',(-208.186188285418,94.7537525712456,5.50669497717542));
#21280=CARTESIAN_POINT('Ctrl Pts',(-206.518653732796,92.1882168600391,5.66560329597973));
#21281=CARTESIAN_POINT('Ctrl Pts',(-203.458834411625,92.20049250483,5.82451161478403));
#21282=CARTESIAN_POINT('Ctrl Pts',(-201.811938476587,94.7793253316762,5.98341993358834));
#21283=CARTESIAN_POINT('Ctrl Pts',(-203.08782171391,97.5604702280067,6.14232825239264));
#21284=CARTESIAN_POINT('Ctrl Pts',(-206.116768631898,97.9942046371468,6.30123657119695));
#21285=CARTESIAN_POINT('Ctrl Pts',(-208.121874550055,95.6828857005571,6.46014489000126));
#21286=CARTESIAN_POINT('Ctrl Pts',(-207.264880773267,92.7455047861689,6.61905320880557));
#21287=CARTESIAN_POINT('Ctrl Pts',(-204.331469617653,91.8750198857941,6.77796152760987));
#21288=CARTESIAN_POINT('Ctrl Pts',(-202.010959644548,93.8694818268668,6.93686984641418));
#21289=CARTESIAN_POINT('Ctrl Pts',(-202.430768461436,96.9003901935,7.09577816521848));
#21290=CARTESIAN_POINT('Ctrl Pts',(-205.206020037109,98.1890420710008,7.25468648402279));
#21291=CARTESIAN_POINT('Ctrl Pts',(-207.792394745404,96.5540158210718,7.4135948028271));
#21292=CARTESIAN_POINT('Ctrl Pts',(-207.818733161131,93.494285235298,7.5725031216314));
#21293=CARTESIAN_POINT('Ctrl Pts',(-205.260888519131,91.8149771167401,7.73141144043572));
#21294=CARTESIAN_POINT('Ctrl Pts',(-202.463864198688,93.0556623792128,7.89031975924001));
#21295=CARTESIAN_POINT('Ctrl Pts',(-201.991940835023,96.0788946409636,8.04922807804433));
#21296=CARTESIAN_POINT('Ctrl Pts',(-204.277772493353,98.1130083544613,8.20813639684863));
#21297=CARTESIAN_POINT('Ctrl Pts',(-207.22573425759,97.2931508020396,8.36704471565294));
#21298=CARTESIAN_POINT('Ctrl Pts',(-208.13316773104,94.3709582243806,8.52595303445724));
#21299=CARTESIAN_POINT('Ctrl Pts',(-206.168148047441,92.0254641159393,8.68486135326156));
#21300=CARTESIAN_POINT('Ctrl Pts',(-203.132183290097,92.4069912602325,8.84376967206585));
#21301=CARTESIAN_POINT('Ctrl Pts',(-201.808612016192,95.1657598356219,9.00267799087017));
#21302=CARTESIAN_POINT('Ctrl Pts',(-203.410869576358,97.7725616463765,9.16158630967448));
#21303=CARTESIAN_POINT('Ctrl Pts',(-206.470024147537,97.8375099280815,9.32049462847878));
#21304=CARTESIAN_POINT('Ctrl Pts',(-208.18147701041,95.3010608219831,9.47940294728308));
#21305=CARTESIAN_POINT('Ctrl Pts',(-206.97618730885,92.4886025191853,9.63831126608739));
#21306=CARTESIAN_POINT('Ctrl Pts',(-203.959151169973,91.9785653574278,9.7972195848917));
#21307=CARTESIAN_POINT('Ctrl Pts',(-201.896353605112,94.2385457060304,9.95612790369601));
#21308=CARTESIAN_POINT('Ctrl Pts',(-202.678944366271,97.1966188407269,10.1150362225003));
#21309=CARTESIAN_POINT('Ctrl Pts',(-205.589452990473,98.1408563733998,10.2739445413046));
#21310=CARTESIAN_POINT('Ctrl Pts',(-207.959557701204,96.2055918876419,10.4328528601089));
#21311=CARTESIAN_POINT('Ctrl Pts',(-207.616372989835,93.1650542339453,10.5917611789132));
#21312=CARTESIAN_POINT('Ctrl Pts',(-204.874526764046,91.8067743497581,10.7506694977175));
#21313=CARTESIAN_POINT('Ctrl Pts',(-202.247712998591,93.3760080516899,10.9095778165218));
#21314=CARTESIAN_POINT('Ctrl Pts',(-202.144165194284,96.43409942081,11.0684861353261));
#21315=CARTESIAN_POINT('Ctrl Pts',(-204.658814820783,98.1774244695644,11.2273944541305));
#21316=CARTESIAN_POINT('Ctrl Pts',(-207.486259206231,97.0077222780384,11.3863027729348));
#21317=CARTESIAN_POINT('Ctrl Pts',(-208.034328939812,93.9973627419037,11.5452110917391));
#21318=CARTESIAN_POINT('Ctrl Pts',(-205.80055981544,91.9062098377222,11.7041194105434));
#21319=CARTESIAN_POINT('Ctrl Pts',(-202.832846399964,92.6514091756644,11.8630277293477));
#21320=CARTESIAN_POINT('Ctrl Pts',(-201.851955183173,95.5497703316425,12.021936048152));
#21321=CARTESIAN_POINT('Ctrl Pts',(-203.757156269404,97.9441081922421,12.1808443669563));
#21322=CARTESIAN_POINT('Ctrl Pts',(-206.801782596837,97.6393205678785,12.3397526857606));
#21323=CARTESIAN_POINT('Ctrl Pts',(-208.194554777643,94.914833346033,12.4986610045649));
#21324=CARTESIAN_POINT('Ctrl Pts',(-206.658594843181,92.2684259606358,12.6575693233692));
#21325=CARTESIAN_POINT('Ctrl Pts',(-203.60205369427,92.1262951243283,12.8164776421735));
#21326=CARTESIAN_POINT('Ctrl Pts',(-201.827134093879,94.6187447991505,12.9753859609778));
#21327=CARTESIAN_POINT('Ctrl Pts',(-202.961062493788,97.4607249810683,13.1342942797821));
#21328=CARTESIAN_POINT('Ctrl Pts',(-205.964266010537,98.046740003011,13.2932025985864));
#21329=CARTESIAN_POINT('Ctrl Pts',(-208.083441226376,95.8395378436917,13.4521109173908));
#21330=CARTESIAN_POINT('Ctrl Pts',(-207.375751988553,92.8626567711379,13.6110192361951));
#21331=CARTESIAN_POINT('Ctrl Pts',(-204.489999881544,91.8452680852187,13.7699275549994));
#21332=CARTESIAN_POINT('Ctrl Pts',(-202.071810181666,93.7201023526643,13.9288358738037));
#21333=CARTESIAN_POINT('Ctrl Pts',(-202.33815218216,96.7683324911026,14.087744192608));
#21334=CARTESIAN_POINT('Ctrl Pts',(-205.044846505554,98.1953751389704,14.2466525114123));
#21335=CARTESIAN_POINT('Ctrl Pts',(-207.710426065418,96.6929336293271,14.4055608302166));
#21336=CARTESIAN_POINT('Ctrl Pts',(-207.891117278559,93.6384293744216,14.5644691490209));
#21337=CARTESIAN_POINT('Ctrl Pts',(-205.421264533382,91.8321980897649,14.7233774678252));
#21338=CARTESIAN_POINT('Ctrl Pts',(-202.565201070578,92.9301716970297,14.8822857866295));
#21339=CARTESIAN_POINT('Ctrl Pts',(-201.941334263506,95.9257417787117,15.0411941054338));
#21340=CARTESIAN_POINT('Ctrl Pts',(-204.121617582424,98.0726000351243,15.2001024242381));
#21341=CARTESIAN_POINT('Ctrl Pts',(-207.107192983917,97.4025372820827,15.3590107430424));
#21342=CARTESIAN_POINT('Ctrl Pts',(-208.160915549491,94.5298461856591,15.5179190618468));
#21343=CARTESIAN_POINT('Ctrl Pts',(-206.316749913415,92.0882054908218,15.676827380651));
#21344=CARTESIAN_POINT('Ctrl Pts',(-203.265394724113,92.3160269221865,15.8357356994554));
#21345=CARTESIAN_POINT('Ctrl Pts',(-201.804322699612,95.0045645412634,15.9946440182597));
#21346=CARTESIAN_POINT('Ctrl Pts',(-203.272977928696,97.6887527328817,16.153552337064));
#21347=CARTESIAN_POINT('Ctrl Pts',(-206.325017939896,97.9082629847128,16.3124606558683));
#21348=CARTESIAN_POINT('Ctrl Pts',(-208.16215113418,95.4608061873071,16.4713689746726));
#21349=CARTESIAN_POINT('Ctrl Pts',(-207.100560253035,92.5923425768892,16.6302772934769));
#21350=CARTESIAN_POINT('Ctrl Pts',(-204.112588839912,91.9281688843269,16.7891856122812));
#21351=CARTESIAN_POINT('Ctrl Pts',(-201.939550299719,94.0864245416824,16.9480939310855));
#21352=CARTESIAN_POINT('Ctrl Pts',(-202.36110058667,96.0727092589846,17.0540328102884));
#21353=CARTESIAN_POINT('Ctrl Pts',(-202.945668449658,96.7564253212268,17.1070022498898));
#21354=CARTESIAN_POINT('Ctrl Pts',(-204.349800002025,92.5679131979649,-0.321006749669433));
#21355=CARTESIAN_POINT('Ctrl Pts',(-203.540360643981,92.7843106836636,-0.268037310067998));
#21356=CARTESIAN_POINT('Ctrl Pts',(-202.168816472716,94.0865592622945,-0.162098430865127));
#21357=CARTESIAN_POINT('Ctrl Pts',(-202.698129229066,96.8897182017072,-0.00319011206082008));
#21358=CARTESIAN_POINT('Ctrl Pts',(-205.3420943899,97.9563584662055,0.155718206743487));
#21359=CARTESIAN_POINT('Ctrl Pts',(-207.670367522821,96.3146411166748,0.314626525547793));
#21360=CARTESIAN_POINT('Ctrl Pts',(-207.55147614183,93.4667171936373,0.4735348443521));
#21361=CARTESIAN_POINT('Ctrl Pts',(-205.092937055701,92.0249536376869,0.632443163156407));
#21362=CARTESIAN_POINT('Ctrl Pts',(-202.549427894286,93.3104550227009,0.791351481960713));
#21363=CARTESIAN_POINT('Ctrl Pts',(-202.252462869042,96.1450208604193,0.950259800765021));
#21364=CARTESIAN_POINT('Ctrl Pts',(-204.474463825331,97.9297918894226,1.10916811956933));
#21365=CARTESIAN_POINT('Ctrl Pts',(-207.178244039411,97.0285878450691,1.26807643837364));
#21366=CARTESIAN_POINT('Ctrl Pts',(-207.885047249673,94.2675848587194,1.42698475717794));
#21367=CARTESIAN_POINT('Ctrl Pts',(-205.946865202589,92.1780578270374,1.58589307598225));
#21368=CARTESIAN_POINT('Ctrl Pts',(-203.140610712076,92.6756529664916,1.74480139478655));
#21369=CARTESIAN_POINT('Ctrl Pts',(-202.039022091796,95.3041848770717,1.90370971359086));
#21370=CARTESIAN_POINT('Ctrl Pts',(-203.652025623394,97.6538428200417,2.06261803239516));
#21371=CARTESIAN_POINT('Ctrl Pts',(-206.500836658906,97.5704876521536,2.22152635119947));
#21372=CARTESIAN_POINT('Ctrl Pts',(-207.973697583819,95.1305379773285,2.38043467000378));
#21373=CARTESIAN_POINT('Ctrl Pts',(-206.720305721087,92.5709126199468,2.53934298880809));
#21374=CARTESIAN_POINT('Ctrl Pts',(-203.889756839074,92.2382473863993,2.6982513076124));
#21375=CARTESIAN_POINT('Ctrl Pts',(-202.077066459509,94.4375260992589,2.8571596264167));
#21376=CARTESIAN_POINT('Ctrl Pts',(-202.944088889806,97.1524745890555,3.01606794522101));
#21377=CARTESIAN_POINT('Ctrl Pts',(-205.695947643099,97.8940584375333,3.17497626402531));
#21378=CARTESIAN_POINT('Ctrl Pts',(-207.80976937776,95.9824018547592,3.33388458282962));
#21379=CARTESIAN_POINT('Ctrl Pts',(-207.347625950087,93.1700902326187,3.49279290163393));
#21380=CARTESIAN_POINT('Ctrl Pts',(-204.733205290795,92.0354194322189,3.65170122043824));
#21381=CARTESIAN_POINT('Ctrl Pts',(-202.363379038756,93.6186429620847,3.81060953924254));
#21382=CARTESIAN_POINT('Ctrl Pts',(-202.410777415132,96.4682791850591,3.96951785804685));
#21383=CARTESIAN_POINT('Ctrl Pts',(-204.831946118055,97.9718134618773,4.12842617685115));
#21384=CARTESIAN_POINT('Ctrl Pts',(-207.407184741668,96.7508223721654,4.28733449565546));
#21385=CARTESIAN_POINT('Ctrl Pts',(-207.775543298713,93.9246969002444,4.44624281445977));
#21386=CARTESIAN_POINT('Ctrl Pts',(-205.599314781178,92.0843972917328,4.60515113326408));
#21387=CARTESIAN_POINT('Ctrl Pts',(-202.873641170674,92.9170896590748,4.76405945206838));
#21388=CARTESIAN_POINT('Ctrl Pts',(-202.097389569024,95.6593709467175,4.92296777087269));
#21389=CARTESIAN_POINT('Ctrl Pts',(-203.982218768616,97.7971483200629,5.08187608967699));
#21390=CARTESIAN_POINT('Ctrl Pts',(-206.800138425611,97.3705313767228,5.24078440848131));
#21391=CARTESIAN_POINT('Ctrl Pts',(-207.96771129378,94.7706377621425,5.3996927272856));
#21392=CARTESIAN_POINT('Ctrl Pts',(-206.414519617308,92.3810208836956,5.55860104608992));
#21393=CARTESIAN_POINT('Ctrl Pts',(-203.564512165481,92.3924547872884,5.71750936489422));
#21394=CARTESIAN_POINT('Ctrl Pts',(-202.03054391619,94.7944569979015,5.87641768369853));
#21395=CARTESIAN_POINT('Ctrl Pts',(-203.21893981554,97.3848987355268,6.03532600250283));
#21396=CARTESIAN_POINT('Ctrl Pts',(-206.040191785461,97.7888919679414,6.19423432130714));
#21397=CARTESIAN_POINT('Ctrl Pts',(-207.90780755248,95.6360602150159,6.35314264011145));
#21398=CARTESIAN_POINT('Ctrl Pts',(-207.10957785535,92.9000955660777,6.51205095891575));
#21399=CARTESIAN_POINT('Ctrl Pts',(-204.37731075875,92.0892998319615,6.67095927772006));
#21400=CARTESIAN_POINT('Ctrl Pts',(-202.215918198859,93.9470014796092,6.82986759652437));
#21401=CARTESIAN_POINT('Ctrl Pts',(-202.606940717148,96.7700804016044,6.98877591532868));
#21402=CARTESIAN_POINT('Ctrl Pts',(-205.191893239227,97.9703693952313,7.14768423413298));
#21403=CARTESIAN_POINT('Ctrl Pts',(-207.600920184333,96.4474569265149,7.30659255293729));
#21404=CARTESIAN_POINT('Ctrl Pts',(-207.62545257439,93.5975321254964,7.46550087174159));
#21405=CARTESIAN_POINT('Ctrl Pts',(-205.242999388387,92.0333741967293,7.6244091905459));
#21406=CARTESIAN_POINT('Ctrl Pts',(-202.637767079064,93.1889856470376,7.7833175093502));
#21407=CARTESIAN_POINT('Ctrl Pts',(-202.198203509467,96.0049148148089,7.94222582815452));
#21408=CARTESIAN_POINT('Ctrl Pts',(-204.32729564729,97.8995493120883,8.10113414695882));
#21409=CARTESIAN_POINT('Ctrl Pts',(-207.073115617,97.1359094077086,8.26004246576313));
#21410=CARTESIAN_POINT('Ctrl Pts',(-207.91832635983,94.4140916309592,8.41895078456744));
#21411=CARTESIAN_POINT('Ctrl Pts',(-206.088048113498,92.22942809837,8.57785910337174));
#21412=CARTESIAN_POINT('Ctrl Pts',(-203.2602595176,92.5847939190855,8.73676742217605));
#21413=CARTESIAN_POINT('Ctrl Pts',(-202.027445551247,95.1543936805248,8.89567574098035));
#21414=CARTESIAN_POINT('Ctrl Pts',(-203.519836279884,97.5824470412848,9.05458405978466));
#21415=CARTESIAN_POINT('Ctrl Pts',(-206.36922456364,97.6429418180719,9.21349237858896));
#21416=CARTESIAN_POINT('Ctrl Pts',(-207.96332307099,95.2804170756647,9.37240069739328));
#21417=CARTESIAN_POINT('Ctrl Pts',(-206.840680107306,92.6608090924519,9.53130901619758));
#21418=CARTESIAN_POINT('Ctrl Pts',(-204.030522194145,92.185745188626,9.69021733500189));
#21419=CARTESIAN_POINT('Ctrl Pts',(-202.109170697738,94.2907586415236,9.8491256538062));
#21420=CARTESIAN_POINT('Ctrl Pts',(-202.838099195444,97.0459966448283,10.0080339726105));
#21421=CARTESIAN_POINT('Ctrl Pts',(-205.549034187648,97.9254877918359,10.1669422914148));
#21422=CARTESIAN_POINT('Ctrl Pts',(-207.756620773058,96.1229244288606,10.3258506102191));
#21423=CARTESIAN_POINT('Ctrl Pts',(-207.436968243909,93.2908765001999,10.4847589290234));
#21424=CARTESIAN_POINT('Ctrl Pts',(-204.883130466234,92.0257338936362,10.6436672478277));
#21425=CARTESIAN_POINT('Ctrl Pts',(-202.436437370889,93.4873652106293,10.802575566632));
#21426=CARTESIAN_POINT('Ctrl Pts',(-202.339989841504,96.3357631961111,10.9614838854363));
#21427=CARTESIAN_POINT('Ctrl Pts',(-204.682209895044,97.9595484129476,11.1203922042407));
#21428=CARTESIAN_POINT('Ctrl Pts',(-207.315776364933,96.8700527230541,11.279300523045));
#21429=CARTESIAN_POINT('Ctrl Pts',(-207.826264946406,94.0661135978575,11.4382088418493));
#21430=CARTESIAN_POINT('Ctrl Pts',(-205.745665413592,92.1183510882897,11.5971171606536));
#21431=CARTESIAN_POINT('Ctrl Pts',(-202.981448163745,92.8124520933842,11.7560254794579));
#21432=CARTESIAN_POINT('Ctrl Pts',(-202.06781667644,95.5120725694926,11.9149337982622));
#21433=CARTESIAN_POINT('Ctrl Pts',(-203.842378087768,97.7422306372212,12.0738421170665));
#21434=CARTESIAN_POINT('Ctrl Pts',(-206.678234329729,97.4583423060864,12.2327504358708));
#21435=CARTESIAN_POINT('Ctrl Pts',(-207.975504095473,94.9206732251237,12.3916587546751));
#21436=CARTESIAN_POINT('Ctrl Pts',(-206.544864963079,92.455730044731,12.5505670734794));
#21437=CARTESIAN_POINT('Ctrl Pts',(-203.697910899177,92.3233451225861,12.7094753922837));
#21438=CARTESIAN_POINT('Ctrl Pts',(-202.044697569714,94.6448874755608,12.868383711088));
#21439=CARTESIAN_POINT('Ctrl Pts',(-203.100872477565,97.2919930220778,13.0272920298923));
#21440=CARTESIAN_POINT('Ctrl Pts',(-205.898146271762,97.837824982764,13.1862003486966));
#21441=CARTESIAN_POINT('Ctrl Pts',(-207.872009602541,95.7819707177012,13.3451086675009));
#21442=CARTESIAN_POINT('Ctrl Pts',(-207.212846629283,93.009214437198,13.5040169863053));
#21443=CARTESIAN_POINT('Ctrl Pts',(-204.524970599415,92.0615881129203,13.6629253051095));
#21444=CARTESIAN_POINT('Ctrl Pts',(-202.272596213484,93.8078649588083,13.8218336239139));
#21445=CARTESIAN_POINT('Ctrl Pts',(-202.520675137913,96.6470778983847,13.9807419427182));
#21446=CARTESIAN_POINT('Ctrl Pts',(-205.041771379811,97.9762682046092,14.1396502615225));
#21447=CARTESIAN_POINT('Ctrl Pts',(-207.5245720983,96.5768491380024,14.2985585803268));
#21448=CARTESIAN_POINT('Ctrl Pts',(-207.692873311502,93.731792298245,14.4574668991311));
#21449=CARTESIAN_POINT('Ctrl Pts',(-205.392378416275,92.0494143273046,14.6163752179354));
#21450=CARTESIAN_POINT('Ctrl Pts',(-202.732155279711,93.0720998633307,14.7752835367397));
#21451=CARTESIAN_POINT('Ctrl Pts',(-202.151067031526,95.8622636472492,14.934191855544));
#21452=CARTESIAN_POINT('Ctrl Pts',(-204.181848281588,97.8619117919808,15.0931001743483));
#21453=CARTESIAN_POINT('Ctrl Pts',(-206.96270272073,97.237795254724,15.2520084931526));
#21454=CARTESIAN_POINT('Ctrl Pts',(-207.94417150984,94.5620846416957,15.4109168119569));
#21455=CARTESIAN_POINT('Ctrl Pts',(-206.226460346682,92.2878672959773,15.5698251307612));
#21456=CARTESIAN_POINT('Ctrl Pts',(-203.384336641039,92.5000670074382,15.7287334495655));
#21457=CARTESIAN_POINT('Ctrl Pts',(-202.023450353188,95.0042515505818,15.8876417683699));
#21458=CARTESIAN_POINT('Ctrl Pts',(-203.391399865139,97.5043849065904,16.0465500871742));
#21459=CARTESIAN_POINT('Ctrl Pts',(-206.234161434428,97.7088433362576,16.2054584059785));
#21460=CARTESIAN_POINT('Ctrl Pts',(-207.945322370463,95.4292086982347,16.3643667247828));
#21461=CARTESIAN_POINT('Ctrl Pts',(-206.956524796331,92.7574356924161,16.5232750435871));
#21462=CARTESIAN_POINT('Ctrl Pts',(-204.173438640123,92.1388044026488,16.6821833623914));
#21463=CARTESIAN_POINT('Ctrl Pts',(-202.14940539417,94.149068428323,16.8410916811957));
#21464=CARTESIAN_POINT('Ctrl Pts',(-202.542049969887,95.9991535645904,16.9470305603986));
#21465=CARTESIAN_POINT('Ctrl Pts',(-203.086534003335,96.6359872033749,17.));
#21466=CARTESIAN_POINT('Ctrl Pts',(-202.485814060779,95.0013541851486,0.887416697508031));
#21467=CARTESIAN_POINT('Ctrl Pts',(-202.484186185477,95.3337585357717,0.908364398593701));
#21468=CARTESIAN_POINT('Ctrl Pts',(-202.545408952213,95.6655886577545,0.929312099679371));
#21469=CARTESIAN_POINT('Ctrl Pts',(-202.672290532631,95.9700550589668,0.950259800765041));
#21470=CARTESIAN_POINT('Ctrl Pts',(-202.993129854472,96.7399445367538,1.00322924036648));
#21471=CARTESIAN_POINT('Ctrl Pts',(-203.733796839902,97.3348682130882,1.05619867996791));
#21472=CARTESIAN_POINT('Ctrl Pts',(-204.554760368296,97.4821293771965,1.10916811956935));
#21473=CARTESIAN_POINT('Ctrl Pts',(-205.375723896691,97.6293905413048,1.16213755917078));
#21474=CARTESIAN_POINT('Ctrl Pts',(-206.276983968051,97.3289891931869,1.21510699877222));
#21475=CARTESIAN_POINT('Ctrl Pts',(-206.845414538775,96.7186213547364,1.26807643837365));
#21476=CARTESIAN_POINT('Ctrl Pts',(-207.413845109498,96.1082535162859,1.32104587797509));
#21477=CARTESIAN_POINT('Ctrl Pts',(-207.649446179586,95.1879191875027,1.37401531757652));
#21478=CARTESIAN_POINT('Ctrl Pts',(-207.444216373449,94.3794975178307,1.42698475717796));
#21479=CARTESIAN_POINT('Ctrl Pts',(-207.238986567312,93.5710758481587,1.4799541967794));
#21480=CARTESIAN_POINT('Ctrl Pts',(-206.592925884951,92.8745668375981,1.53292363638083));
#21481=CARTESIAN_POINT('Ctrl Pts',(-205.802186462018,92.6092448555601,1.58589307598227));
#21482=CARTESIAN_POINT('Ctrl Pts',(-205.011447039085,92.3439228735221,1.6388625155837));
#21483=CARTESIAN_POINT('Ctrl Pts',(-204.07602887558,92.5097879200068,1.69183195518514));
#21484=CARTESIAN_POINT('Ctrl Pts',(-203.424721690448,93.0308090950125,1.74480139478657));
#21485=CARTESIAN_POINT('Ctrl Pts',(-202.840193630047,93.498409489736,1.79233982902706));
#21486=CARTESIAN_POINT('Ctrl Pts',(-202.484502970261,94.2520706545457,1.83987826326755));
#21487=CARTESIAN_POINT('Ctrl Pts',(-202.479323465531,95.0014637551426,1.88741669750803));
#21488=CARTESIAN_POINT('Ctrl Pts',(-204.206200717467,92.0307770462543,-1.66533453693773E-15));
#21489=CARTESIAN_POINT('Ctrl Pts',(-204.113164546597,92.0648100931486,-1.69173089419692E-15));
#21490=CARTESIAN_POINT('Ctrl Pts',(-204.022195753339,92.1036152875412,-1.82627024830213E-15));
#21491=CARTESIAN_POINT('Ctrl Pts',(-203.93350174438,92.146863146562,-1.76247905159244E-15));
#21492=CARTESIAN_POINT('Ctrl Pts',(-203.842828689001,92.1910760033496,-1.69726446968485E-15));
#21493=CARTESIAN_POINT('Ctrl Pts',(-203.754532399231,92.239932614376,-1.71252452587887E-15));
#21494=CARTESIAN_POINT('Ctrl Pts',(-203.668863408233,92.2931265192584,-1.74513181683267E-15));
#21495=CARTESIAN_POINT('Ctrl Pts',(-203.585834980389,92.3446808359581,-1.77673405788396E-15));
#21496=CARTESIAN_POINT('Ctrl Pts',(-203.505274053601,92.4003100531731,-2.01192529436932E-15));
#21497=CARTESIAN_POINT('Ctrl Pts',(-203.42744252456,92.4597659845155,-2.08166817117217E-15));
#21498=CARTESIAN_POINT('Ctrl Pts',(-203.359339936648,92.5117899244401,-2.14269318837466E-15));
#21499=CARTESIAN_POINT('Ctrl Pts',(-203.293327341741,92.5667444131619,-1.8186794360701E-15));
#21500=CARTESIAN_POINT('Ctrl Pts',(-203.229605551781,92.6244761991185,-1.81105130891979E-15));
#21501=CARTESIAN_POINT('Ctrl Pts',(-203.216356049157,92.6364802161122,-1.80946521269176E-15));
#21502=CARTESIAN_POINT('Ctrl Pts',(-203.20320393314,92.6486060983002,-8.45553191946793E-16));
#21503=CARTESIAN_POINT('Ctrl Pts',(-203.190167894587,92.6608364292545,-8.60422844084496E-16));
#21504=CARTESIAN_POINT('Ctrl Pts',(-203.117744720063,92.7287834048338,-9.43032864569248E-16));
#21505=CARTESIAN_POINT('Ctrl Pts',(-203.048787356972,92.800052338559,-1.63384023442941E-15));
#21506=CARTESIAN_POINT('Ctrl Pts',(-202.983534916614,92.8743511143521,-1.51267887105178E-15));
#21507=CARTESIAN_POINT('Ctrl Pts',(-202.918640599649,92.9482421179686,-1.39218247465811E-15));
#21508=CARTESIAN_POINT('Ctrl Pts',(-202.857410164585,93.0251305974732,-1.61166620503164E-15));
#21509=CARTESIAN_POINT('Ctrl Pts',(-202.800122429229,93.1047559605022,-1.70696790036118E-15));
#21510=CARTESIAN_POINT('Ctrl Pts',(-202.744171241289,93.1825236296888,-1.80004616629764E-15));
#21511=CARTESIAN_POINT('Ctrl Pts',(-202.691980644036,93.2629027086335,-1.49993186602241E-15));
#21512=CARTESIAN_POINT('Ctrl Pts',(-202.643857548798,93.3456645933452,-1.47104550762833E-15));
#21513=CARTESIAN_POINT('Ctrl Pts',(-202.623078179889,93.3814008593852,-1.45857248828985E-15));
#21514=CARTESIAN_POINT('Ctrl Pts',(-202.603057818574,93.4175815121137,-2.11179019747899E-15));
#21515=CARTESIAN_POINT('Ctrl Pts',(-202.58382418876,93.4541884794612,-2.15105711021124E-15));
#21516=CARTESIAN_POINT('Ctrl Pts',(-202.569909256858,93.480672479761,-2.17946549812013E-15));
#21517=CARTESIAN_POINT('Ctrl Pts',(-202.556406144173,93.5073796196226,-1.83372961098251E-15));
#21518=CARTESIAN_POINT('Ctrl Pts',(-202.543325986125,93.5343030584598,-1.87350135405495E-15));
#21519=CARTESIAN_POINT('Ctrl Pts',(-202.537164396374,93.5469857175079,-1.89223638490238E-15));
#21520=CARTESIAN_POINT('Ctrl Pts',(-202.53109884915,93.559711973925,-1.76798935478286E-15));
#21521=CARTESIAN_POINT('Ctrl Pts',(-202.525133507599,93.5724739887755,-1.76247905159244E-15));
#21522=CARTESIAN_POINT('Ctrl Pts',(-202.485117234082,93.6580832154258,-1.72551523355393E-15));
#21523=CARTESIAN_POINT('Ctrl Pts',(-202.449559207413,93.7453964352435,-1.29272896296815E-15));
#21524=CARTESIAN_POINT('Ctrl Pts',(-202.418711137482,93.8341759498457,-1.38777878078145E-15));
#21525=CARTESIAN_POINT('Ctrl Pts',(-202.388547297845,93.9209862769557,-1.48072033169087E-15));
#21526=CARTESIAN_POINT('Ctrl Pts',(-202.362886576913,94.0091992471836,-1.88906384068916E-15));
#21527=CARTESIAN_POINT('Ctrl Pts',(-202.342013489097,94.0986011792945,-1.97064586870965E-15));
#21528=CARTESIAN_POINT('Ctrl Pts',(-202.338634265004,94.1130748003348,-1.98385349554043E-15));
#21529=CARTESIAN_POINT('Ctrl Pts',(-202.335380633682,94.1275795899092,-2.29719255525669E-15));
#21530=CARTESIAN_POINT('Ctrl Pts',(-202.332253933038,94.1421146450262,-2.3037127760972E-15));
#21531=CARTESIAN_POINT('Ctrl Pts',(-202.312215536415,94.2352668948282,-2.34442810623525E-15));
#21532=CARTESIAN_POINT('Ctrl Pts',(-202.297386423123,94.3296632853158,-1.89809370242541E-15));
#21533=CARTESIAN_POINT('Ctrl Pts',(-202.287688012511,94.4248955183014,-1.88737914186277E-15));
#21534=CARTESIAN_POINT('Ctrl Pts',(-202.284332068712,94.4578487551403,-1.88367157940438E-15));
#21535=CARTESIAN_POINT('Ctrl Pts',(-202.281590899577,94.4909019448947,-1.99130593283213E-15));
#21536=CARTESIAN_POINT('Ctrl Pts',(-202.279462603563,94.5240376464396,-2.02615701994091E-15));
#21537=CARTESIAN_POINT('Ctrl Pts',(-202.278435428223,94.5400298652337,-2.04297713191284E-15));
#21538=CARTESIAN_POINT('Ctrl Pts',(-202.277551019282,94.5560412983696,-1.44883699021621E-15));
#21539=CARTESIAN_POINT('Ctrl Pts',(-202.276809217809,94.5720699538646,-1.4432899320127E-15));
#21540=CARTESIAN_POINT('Ctrl Pts',(-202.276232566489,94.5845300872998,-1.43897783700198E-15));
#21541=CARTESIAN_POINT('Ctrl Pts',(-202.275742191968,94.5969994802251,-1.93405229558996E-15));
#21542=CARTESIAN_POINT('Ctrl Pts',(-202.275338169858,94.6094673056919,-1.9151347174784E-15));
#21543=CARTESIAN_POINT('Ctrl Pts',(-202.272318849975,94.7026412989672,-1.77376072243412E-15));
#21544=CARTESIAN_POINT('Ctrl Pts',(-202.274110256434,94.7958785363416,-1.40451656878397E-15));
#21545=CARTESIAN_POINT('Ctrl Pts',(-202.280572703129,94.8888046622951,-1.47104550762833E-15));
#21546=CARTESIAN_POINT('Ctrl Pts',(-202.287048646371,94.9819248605413,-1.5377133893541E-15));
#21547=CARTESIAN_POINT('Ctrl Pts',(-202.298215544432,95.0747336270844,-1.60767188909222E-15));
#21548=CARTESIAN_POINT('Ctrl Pts',(-202.313983907893,95.166842280173,-1.69309011255336E-15));
#21549=CARTESIAN_POINT('Ctrl Pts',(-202.329531048883,95.2576586936497,-1.77730995987682E-15));
#21550=CARTESIAN_POINT('Ctrl Pts',(-202.34955191658,95.3477953472331,-1.39699777228343E-15));
#21551=CARTESIAN_POINT('Ctrl Pts',(-202.374003812269,95.4368545695215,-1.36002320516582E-15));
#21552=CARTESIAN_POINT('Ctrl Pts',(-202.383516754342,95.4715028124848,-1.34563835256958E-15));
#21553=CARTESIAN_POINT('Ctrl Pts',(-202.39370079569,95.5059876390941,-2.03473279209489E-15));
#21554=CARTESIAN_POINT('Ctrl Pts',(-202.404554992678,95.5402841682775,-2.05391259555654E-15));
#21555=CARTESIAN_POINT('Ctrl Pts',(-202.410353828332,95.5586070286854,-2.06415937182937E-15));
#21556=CARTESIAN_POINT('Ctrl Pts',(-202.4163439549,95.5768761294375,-1.49239684807345E-15));
#21557=CARTESIAN_POINT('Ctrl Pts',(-202.422525324126,95.5950875623995,-1.49880108324396E-15));
#21558=CARTESIAN_POINT('Ctrl Pts',(-202.428042981199,95.6113435791845,-1.50451767647659E-15));
#21559=CARTESIAN_POINT('Ctrl Pts',(-202.433713558872,95.6275548911267,-1.38447419983314E-15));
#21560=CARTESIAN_POINT('Ctrl Pts',(-202.439530699397,95.6437017576532,-1.41553435639707E-15));
#21561=CARTESIAN_POINT('Ctrl Pts',(-202.470363847948,95.7292865449133,-1.58016548698939E-15));
#21562=CARTESIAN_POINT('Ctrl Pts',(-202.505347385225,95.8131730030787,-1.91068776190809E-15));
#21563=CARTESIAN_POINT('Ctrl Pts',(-202.54441704991,95.8949805098665,-1.77635683940025E-15));
#21564=CARTESIAN_POINT('Ctrl Pts',(-202.575879531626,95.9608594265972,-1.66818124518231E-15));
#21565=CARTESIAN_POINT('Ctrl Pts',(-202.609992760709,96.025389849449,-1.40994256838161E-15));
#21566=CARTESIAN_POINT('Ctrl Pts',(-202.646741380164,96.0883553006046,-1.4432899320127E-15));
#21567=CARTESIAN_POINT('Ctrl Pts',(-202.66198370497,96.1144716519744,-1.4571215086927E-15));
#21568=CARTESIAN_POINT('Ctrl Pts',(-202.677679592969,96.1403185550972,-1.31270100888093E-15));
#21569=CARTESIAN_POINT('Ctrl Pts',(-202.693828681531,96.165879569832,-1.33226762955019E-15));
#21570=CARTESIAN_POINT('Ctrl Pts',(-202.702295555836,96.1792810629265,-1.3425262962934E-15));
#21571=CARTESIAN_POINT('Ctrl Pts',(-202.71088559022,96.1926016065556,-1.61636770759439E-15));
#21572=CARTESIAN_POINT('Ctrl Pts',(-202.719593926003,96.2058319566941,-1.60982338570648E-15));
#21573=CARTESIAN_POINT('Ctrl Pts',(-202.767002660722,96.2778588256104,-1.57419568048102E-15));
#21574=CARTESIAN_POINT('Ctrl Pts',(-202.817953855461,96.347277505506,-1.59581768743097E-15));
#21575=CARTESIAN_POINT('Ctrl Pts',(-202.872410801174,96.4137327204673,-1.22124532708767E-15));
#21576=CARTESIAN_POINT('Ctrl Pts',(-202.926867746887,96.4801879354285,-8.46672966744377E-16));
#21577=CARTESIAN_POINT('Ctrl Pts',(-202.984830774458,96.5436803772796,-3.7899909010744E-16));
#21578=CARTESIAN_POINT('Ctrl Pts',(-203.046292669322,96.6038107748045,-2.22044604925031E-16));
#21579=CARTESIAN_POINT('Ctrl Pts',(-203.058343445767,96.6156004858078,-1.91270685291611E-16));
#21580=CARTESIAN_POINT('Ctrl Pts',(-203.070528813095,96.6272607941278,-2.35826789791532E-16));
#21581=CARTESIAN_POINT('Ctrl Pts',(-203.082846187392,96.6387906377555,-2.22044604925031E-16));
#21582=CARTESIAN_POINT('Origin',(-205.,95.,9.));
#21583=CARTESIAN_POINT('Origin',(-205.,65.,18.));
#21584=CARTESIAN_POINT('Origin',(-205.,-95.,18.));
#21585=CARTESIAN_POINT('Origin',(-205.,-65.,18.));
#21586=CARTESIAN_POINT('Origin',(-205.,95.,18.));
#21587=CARTESIAN_POINT('Origin',(170.,-120.,0.));
#21588=CARTESIAN_POINT('',(170.,-120.,0.));
#21589=CARTESIAN_POINT('',(-170.,-120.,0.));
#21590=CARTESIAN_POINT('',(-170.,-120.,0.));
#21591=CARTESIAN_POINT('',(-170.,-120.,20.));
#21592=CARTESIAN_POINT('',(-170.,-120.,0.));
#21593=CARTESIAN_POINT('',(170.,-120.,20.));
#21594=CARTESIAN_POINT('',(-170.,-120.,20.));
#21595=CARTESIAN_POINT('',(170.,-120.,0.));
#21596=CARTESIAN_POINT('Origin',(170.,120.,0.));
#21597=CARTESIAN_POINT('',(170.,120.,0.));
#21598=CARTESIAN_POINT('',(170.,-120.,0.));
#21599=CARTESIAN_POINT('',(170.,120.,20.));
#21600=CARTESIAN_POINT('',(170.,-120.,20.));
#21601=CARTESIAN_POINT('',(170.,120.,0.));
#21602=CARTESIAN_POINT('Origin',(-170.,120.,0.));
#21603=CARTESIAN_POINT('',(-170.,120.,0.));
#21604=CARTESIAN_POINT('',(170.,120.,0.));
#21605=CARTESIAN_POINT('',(-170.,120.,20.));
#21606=CARTESIAN_POINT('',(170.,120.,20.));
#21607=CARTESIAN_POINT('',(-170.,120.,0.));
#21608=CARTESIAN_POINT('Origin',(-170.,-120.,0.));
#21609=CARTESIAN_POINT('',(-170.,120.,0.));
#21610=CARTESIAN_POINT('',(-170.,120.,20.));
#21611=CARTESIAN_POINT('Origin',(215.,155.,0.));
#21612=CARTESIAN_POINT('',(220.,155.,0.));
#21613=CARTESIAN_POINT('',(-220.,155.,0.));
#21614=CARTESIAN_POINT('',(107.5,155.,0.));
#21615=CARTESIAN_POINT('',(-220.,155.,20.));
#21616=CARTESIAN_POINT('',(-220.,155.,0.));
#21617=CARTESIAN_POINT('',(220.,155.,20.));
#21618=CARTESIAN_POINT('',(107.5,155.,20.));
#21619=CARTESIAN_POINT('',(220.,155.,0.));
#21620=CARTESIAN_POINT('Origin',(220.,-150.,0.));
#21621=CARTESIAN_POINT('',(220.,-155.,0.));
#21622=CARTESIAN_POINT('',(220.,-75.,0.));
#21623=CARTESIAN_POINT('',(220.,-155.,20.));
#21624=CARTESIAN_POINT('',(220.,-75.,20.));
#21625=CARTESIAN_POINT('',(220.,-155.,0.));
#21626=CARTESIAN_POINT('Origin',(-215.,-155.,0.));
#21627=CARTESIAN_POINT('',(-220.,-155.,0.));
#21628=CARTESIAN_POINT('',(-107.5,-155.,0.));
#21629=CARTESIAN_POINT('',(-220.,-155.,20.));
#21630=CARTESIAN_POINT('',(-107.5,-155.,20.));
#21631=CARTESIAN_POINT('',(-220.,-155.,0.));
#21632=CARTESIAN_POINT('Origin',(-220.,150.,0.));
#21633=CARTESIAN_POINT('',(-220.,75.,0.));
#21634=CARTESIAN_POINT('',(-220.,75.,20.));
#21635=CARTESIAN_POINT('Origin',(0.,0.,20.));
#21636=CARTESIAN_POINT('Origin',(0.,0.,0.));
#32589=UNCERTAINTY_MEASURE_WITH_UNIT(LENGTH_MEASURE(0.01),#32628,
'DISTANCE_ACCURACY_VALUE',
'Maximum model space distance between geometric entities at asserted c
onnectivities');
#32607=UNCERTAINTY_MEASURE_WITH_UNIT(LENGTH_MEASURE(0.01),#32628,
'DISTANCE_ACCURACY_VALUE',
'Maximum model space distance between geometric entities at asserted c
onnectivities');
#32609=(
GEOMETRIC_REPRESENTATION_CONTEXT(3)
GLOBAL_UNCERTAINTY_ASSIGNED_CONTEXT((#32589))
GLOBAL_UNIT_ASSIGNED_CONTEXT((#32628,#32630,#32631))
REPRESENTATION_CONTEXT('','3D')
);
#32627=(
GEOMETRIC_REPRESENTATION_CONTEXT(3)
GLOBAL_UNCERTAINTY_ASSIGNED_CONTEXT((#32607))
GLOBAL_UNIT_ASSIGNED_CONTEXT((#32628,#32630,#32631))
REPRESENTATION_CONTEXT('','3D')
);
#32628=(
LENGTH_UNIT()
NAMED_UNIT(*)
SI_UNIT(.MILLI.,.METRE.)
);
#32630=(
NAMED_UNIT(*)
PLANE_ANGLE_UNIT()
SI_UNIT($,.RADIAN.)
);
#32631=(
NAMED_UNIT(*)
SI_UNIT($,.STERADIAN.)
SOLID_ANGLE_UNIT()
);
#32633=SHAPE_DEFINITION_REPRESENTATION(#32652,#32708);
#32652=PRODUCT_DEFINITION_SHAPE('',$,#32728);
#32708=SHAPE_REPRESENTATION('',(#8893),#32609);
#32726=PRODUCT_DEFINITION_CONTEXT('part definition',#32785,'design');
#32728=PRODUCT_DEFINITION('Mounting frame','Mounting frame',#32747,#32726);
#32747=PRODUCT_DEFINITION_FORMATION('',$,#32788);
#32785=APPLICATION_CONTEXT(
'Core Data for Automotive Mechanical Design Process');
#32786=PRODUCT_CONTEXT('part definition',#32785,'mechanical');
#32788=PRODUCT('Mounting frame','Mounting frame',$,(#32786));
#32807=PRESENTATION_STYLE_ASSIGNMENT((#32814));
#32814=SURFACE_STYLE_USAGE(.BOTH.,#32821);
#32821=SURFACE_SIDE_STYLE('',(#32828));
#32828=SURFACE_STYLE_FILL_AREA(#32835);
#32835=FILL_AREA_STYLE('Dark blue',(#32842));
#32842=FILL_AREA_STYLE_COLOUR('Dark blue',#32849);
#32849=COLOUR_RGB('Dark blue',0.0901960784313725,0.270588235294118,0.513725490196078);
ENDSEC;
END-ISO-10303-21;
